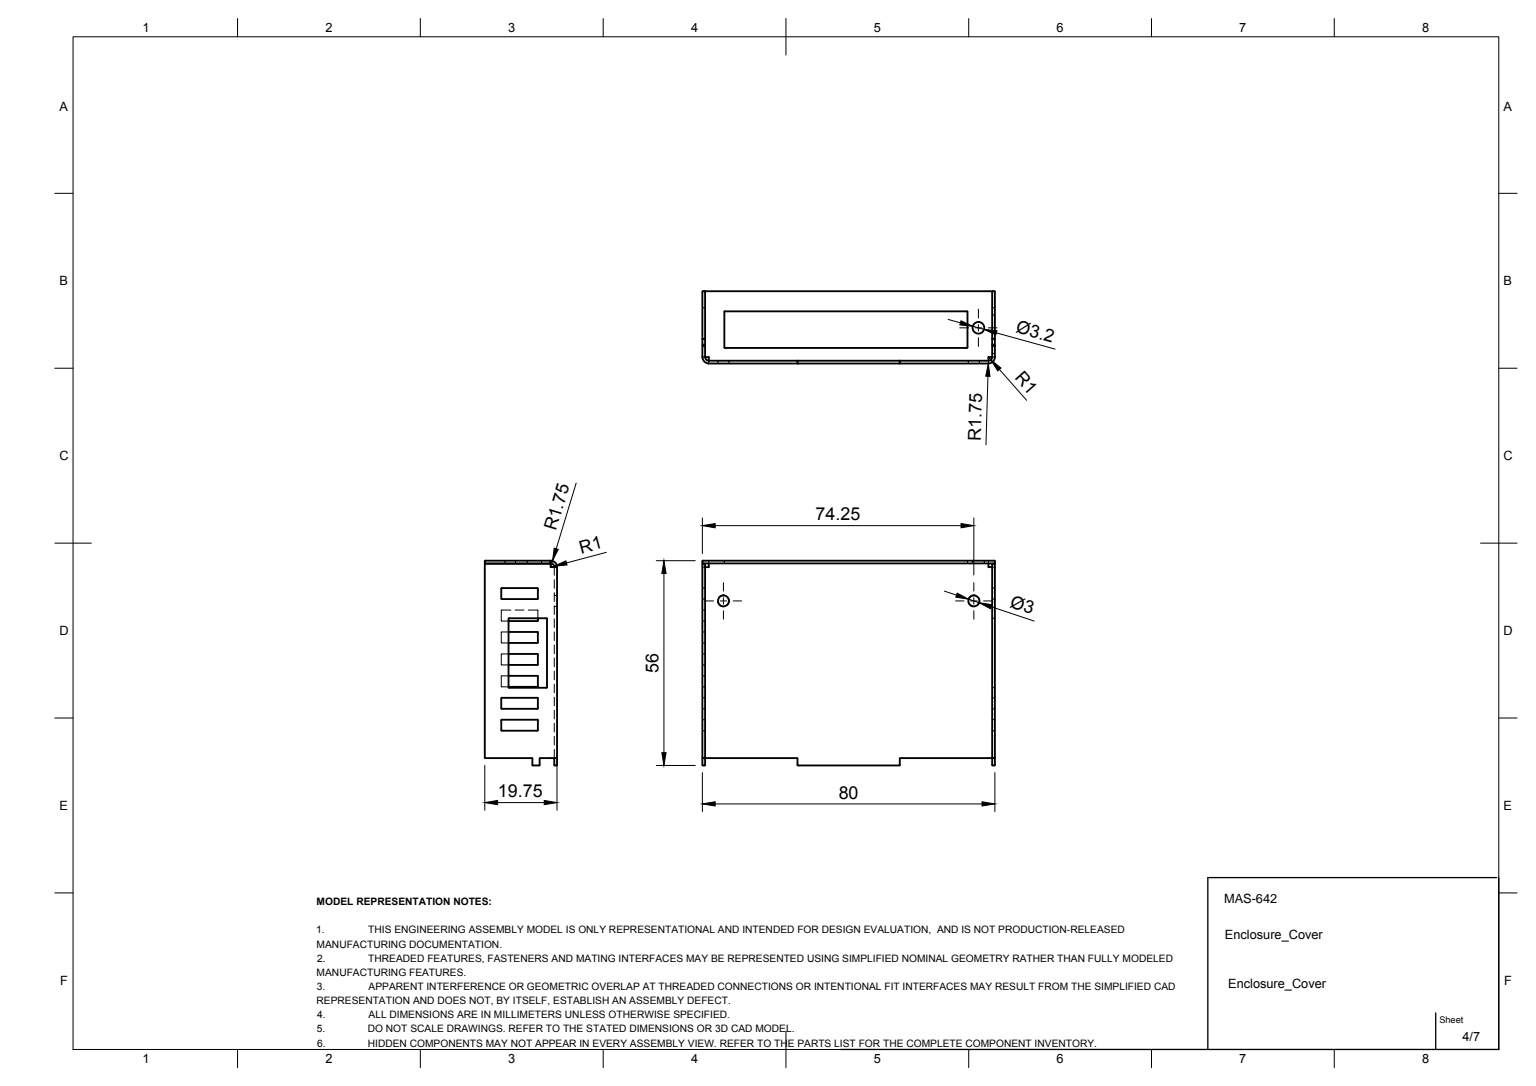
ISO-10303-21;
HEADER;
FILE_DESCRIPTION((''),'2;1');
FILE_NAME('Enclosure_Cover.step','2026-10-09T09:51:33-07:00',(''),(''),'','','');
FILE_SCHEMA (('AUTOMOTIVE_DESIGN { 1 0 10303 214 3 1 1 }'));
ENDSEC;
DATA;
#10=MECHANICAL_DESIGN_GEOMETRIC_PRESENTATION_REPRESENTATION('',(#481),#126571);
#469=SHAPE_REPRESENTATION_RELATIONSHIP('SRR','None',#126599,#475) ;
#475=ADVANCED_BREP_SHAPE_REPRESENTATION('',(#4172),#126565) ;
#481=STYLED_ITEM('',(#126638),#4172) ;
#4172=MANIFOLD_SOLID_BREP('Body1',#67686) ;
#4182=SPHERICAL_SURFACE('',#68025,0.15) ;
#4183=SPHERICAL_SURFACE('',#68034,0.15) ;
#4184=SPHERICAL_SURFACE('',#68036,0.15) ;
#4185=SPHERICAL_SURFACE('',#68045,0.15) ;
#4186=SPHERICAL_SURFACE('',#68058,0.15) ;
#4187=SPHERICAL_SURFACE('',#68067,0.15) ;
#4188=SPHERICAL_SURFACE('',#68069,0.15) ;
#4189=SPHERICAL_SURFACE('',#68081,0.15) ;
#4190=SPHERICAL_SURFACE('',#68086,0.15) ;
#4191=SPHERICAL_SURFACE('',#68107,0.15) ;
#4192=SPHERICAL_SURFACE('',#68110,0.15) ;
#4193=SPHERICAL_SURFACE('',#68130,0.15) ;
#4194=SPHERICAL_SURFACE('',#68146,0.15) ;
#4195=SPHERICAL_SURFACE('',#68149,0.15) ;
#4196=SPHERICAL_SURFACE('',#68166,0.15) ;
#4197=SPHERICAL_SURFACE('',#68168,0.15) ;
#4198=SPHERICAL_SURFACE('',#68174,0.15) ;
#4199=SPHERICAL_SURFACE('',#68177,0.15) ;
#4200=SPHERICAL_SURFACE('',#68195,0.15) ;
#4201=SPHERICAL_SURFACE('',#68201,0.15) ;
#4202=SPHERICAL_SURFACE('',#68757,0.15) ;
#4203=SPHERICAL_SURFACE('',#68763,0.15) ;
#4204=SPHERICAL_SURFACE('',#68773,0.15) ;
#4205=SPHERICAL_SURFACE('',#68775,0.15) ;
#4840=ELLIPSE('',#68022,0.212132034355858,0.149999999999913) ;
#4841=ELLIPSE('',#68024,0.212132034356981,0.150000000000627) ;
#4842=ELLIPSE('',#68079,0.21213203435611,0.150000000000114) ;
#4843=ELLIPSE('',#68090,0.212132034356462,0.150000000000298) ;
#4844=ELLIPSE('',#68749,0.212132034356202,0.150000000000162) ;
#4845=ELLIPSE('',#68753,0.212132034355904,0.149999999999933) ;
#4846=ELLIPSE('',#68760,0.212132034354929,0.149999999999304) ;
#4847=ELLIPSE('',#68762,0.212132034356004,0.150000000000028) ;
#4989=FACE_BOUND('',#20413,.T.) ;
#4990=FACE_BOUND('',#20414,.T.) ;
#4991=FACE_BOUND('',#20416,.T.) ;
#4992=FACE_BOUND('',#20417,.T.) ;
#4993=FACE_BOUND('',#20419,.T.) ;
#4994=FACE_BOUND('',#20420,.T.) ;
#4995=FACE_BOUND('',#20421,.T.) ;
#4996=FACE_BOUND('',#20422,.T.) ;
#4997=FACE_BOUND('',#20424,.T.) ;
#4998=FACE_BOUND('',#20425,.T.) ;
#4999=FACE_BOUND('',#20426,.T.) ;
#5000=FACE_BOUND('',#20427,.T.) ;
#5001=FACE_BOUND('',#20429,.T.) ;
#5002=FACE_BOUND('',#20430,.T.) ;
#5003=FACE_BOUND('',#20431,.T.) ;
#5004=FACE_BOUND('',#20432,.T.) ;
#5005=FACE_BOUND('',#20433,.T.) ;
#5006=FACE_BOUND('',#20434,.T.) ;
#5007=FACE_BOUND('',#20435,.T.) ;
#5008=FACE_BOUND('',#20437,.T.) ;
#5009=FACE_BOUND('',#20438,.T.) ;
#5010=FACE_BOUND('',#20439,.T.) ;
#5011=FACE_BOUND('',#20440,.T.) ;
#5012=FACE_BOUND('',#20441,.T.) ;
#5013=FACE_BOUND('',#20442,.T.) ;
#5014=FACE_BOUND('',#20443,.T.) ;
#5015=FACE_BOUND('',#20445,.T.) ;
#5016=FACE_BOUND('',#20446,.T.) ;
#5017=FACE_BOUND('',#20448,.T.) ;
#5018=FACE_BOUND('',#20449,.T.) ;
#5065=PLANE('',#67802) ;
#5066=PLANE('',#67807) ;
#5067=PLANE('',#67812) ;
#5068=PLANE('',#67831) ;
#5069=PLANE('',#67850) ;
#5070=PLANE('',#67881) ;
#5071=PLANE('',#67912) ;
#5072=PLANE('',#67915) ;
#5073=PLANE('',#67918) ;
#5074=PLANE('',#67919) ;
#5075=PLANE('',#67920) ;
#5076=PLANE('',#67921) ;
#5077=PLANE('',#67922) ;
#5078=PLANE('',#67923) ;
#5079=PLANE('',#67926) ;
#5080=PLANE('',#67933) ;
#5081=PLANE('',#67934) ;
#5082=PLANE('',#67935) ;
#5083=PLANE('',#67936) ;
#5084=PLANE('',#67937) ;
#5085=PLANE('',#67938) ;
#5086=PLANE('',#67939) ;
#5087=PLANE('',#67940) ;
#5088=PLANE('',#67941) ;
#5089=PLANE('',#67942) ;
#5090=PLANE('',#67943) ;
#5091=PLANE('',#67944) ;
#5092=PLANE('',#67945) ;
#5093=PLANE('',#67946) ;
#5094=PLANE('',#67949) ;
#5095=PLANE('',#67954) ;
#5096=PLANE('',#67957) ;
#5097=PLANE('',#67964) ;
#5098=PLANE('',#67965) ;
#5099=PLANE('',#67966) ;
#5100=PLANE('',#67967) ;
#5101=PLANE('',#67968) ;
#5102=PLANE('',#67969) ;
#5103=PLANE('',#67970) ;
#5104=PLANE('',#67971) ;
#5105=PLANE('',#67972) ;
#5106=PLANE('',#67973) ;
#5107=PLANE('',#67974) ;
#5108=PLANE('',#67975) ;
#5109=PLANE('',#67976) ;
#5110=PLANE('',#67977) ;
#5111=PLANE('',#67978) ;
#5112=PLANE('',#67979) ;
#5113=PLANE('',#67980) ;
#5114=PLANE('',#67981) ;
#5115=PLANE('',#67982) ;
#5116=PLANE('',#67983) ;
#5117=PLANE('',#67984) ;
#5118=PLANE('',#67985) ;
#5119=PLANE('',#67986) ;
#5120=PLANE('',#67987) ;
#5121=PLANE('',#67988) ;
#5122=PLANE('',#67989) ;
#5123=PLANE('',#67990) ;
#5124=PLANE('',#67991) ;
#5125=PLANE('',#67992) ;
#5126=PLANE('',#67993) ;
#5127=PLANE('',#67994) ;
#5128=PLANE('',#67995) ;
#5129=PLANE('',#67996) ;
#5130=PLANE('',#67997) ;
#5131=PLANE('',#67998) ;
#5132=PLANE('',#67999) ;
#5133=PLANE('',#68000) ;
#5134=PLANE('',#68001) ;
#5135=PLANE('',#68002) ;
#5136=PLANE('',#68003) ;
#5137=PLANE('',#68004) ;
#5138=PLANE('',#68005) ;
#5139=PLANE('',#68006) ;
#5140=PLANE('',#68007) ;
#5141=PLANE('',#68008) ;
#5142=PLANE('',#68009) ;
#5143=PLANE('',#68010) ;
#5144=PLANE('',#68011) ;
#5145=PLANE('',#68012) ;
#5146=PLANE('',#68013) ;
#5147=PLANE('',#68014) ;
#5148=PLANE('',#68015) ;
#5149=PLANE('',#68016) ;
#5150=PLANE('',#68017) ;
#5151=PLANE('',#68018) ;
#5152=PLANE('',#68019) ;
#5947=CYLINDRICAL_SURFACE('',#67797,1.49999999999999) ;
#5948=CYLINDRICAL_SURFACE('',#67800,1.49999999999999) ;
#5949=CYLINDRICAL_SURFACE('',#67801,1.6) ;
#5950=CYLINDRICAL_SURFACE('',#67929,1.75) ;
#5951=CYLINDRICAL_SURFACE('',#67931,1.) ;
#5952=CYLINDRICAL_SURFACE('',#67952,1.75) ;
#5953=CYLINDRICAL_SURFACE('',#67953,1.) ;
#5954=CYLINDRICAL_SURFACE('',#67960,1.75) ;
#5955=CYLINDRICAL_SURFACE('',#67962,1.) ;
#5956=CYLINDRICAL_SURFACE('',#68020,0.149999999999997) ;
#5957=CYLINDRICAL_SURFACE('',#68023,0.15) ;
#5958=CYLINDRICAL_SURFACE('',#68028,0.149999999999997) ;
#5959=CYLINDRICAL_SURFACE('',#68030,0.149999999999997) ;
#5960=CYLINDRICAL_SURFACE('',#68032,0.149999999999997) ;
#5961=CYLINDRICAL_SURFACE('',#68039,0.149999999999997) ;
#5962=CYLINDRICAL_SURFACE('',#68041,0.15) ;
#5963=CYLINDRICAL_SURFACE('',#68043,0.149999999999997) ;
#5964=CYLINDRICAL_SURFACE('',#68050,0.149999999999997) ;
#5965=CYLINDRICAL_SURFACE('',#68052,0.15) ;
#5966=CYLINDRICAL_SURFACE('',#68054,0.149999999999997) ;
#5967=CYLINDRICAL_SURFACE('',#68061,0.149999999999997) ;
#5968=CYLINDRICAL_SURFACE('',#68063,0.15) ;
#5969=CYLINDRICAL_SURFACE('',#68065,0.149999999999997) ;
#5970=CYLINDRICAL_SURFACE('',#68072,0.149999999999997) ;
#5971=CYLINDRICAL_SURFACE('',#68074,0.15) ;
#5972=CYLINDRICAL_SURFACE('',#68076,0.149999999999997) ;
#5973=CYLINDRICAL_SURFACE('',#68078,0.149999999999997) ;
#5974=CYLINDRICAL_SURFACE('',#68089,0.15) ;
#5975=CYLINDRICAL_SURFACE('',#68091,0.149999999999997) ;
#5976=CYLINDRICAL_SURFACE('',#68093,0.15) ;
#5977=CYLINDRICAL_SURFACE('',#68095,0.149999999999997) ;
#5978=CYLINDRICAL_SURFACE('',#68097,0.150000000000001) ;
#5979=CYLINDRICAL_SURFACE('',#68099,0.150000000000001) ;
#5980=CYLINDRICAL_SURFACE('',#68101,0.149999999999997) ;
#5981=CYLINDRICAL_SURFACE('',#68112,0.149999999999997) ;
#5982=CYLINDRICAL_SURFACE('',#68114,0.15) ;
#5983=CYLINDRICAL_SURFACE('',#68116,0.15) ;
#5984=CYLINDRICAL_SURFACE('',#68118,0.15) ;
#5985=CYLINDRICAL_SURFACE('',#68120,0.150000000000001) ;
#5986=CYLINDRICAL_SURFACE('',#68132,0.15) ;
#5987=CYLINDRICAL_SURFACE('',#68134,0.150000000000001) ;
#5988=CYLINDRICAL_SURFACE('',#68136,0.15) ;
#5989=CYLINDRICAL_SURFACE('',#68138,0.15) ;
#5990=CYLINDRICAL_SURFACE('',#68140,0.15) ;
#5991=CYLINDRICAL_SURFACE('',#68142,0.15) ;
#5992=CYLINDRICAL_SURFACE('',#68154,0.15) ;
#5993=CYLINDRICAL_SURFACE('',#68156,0.150000000000001) ;
#5994=CYLINDRICAL_SURFACE('',#68158,0.15) ;
#5995=CYLINDRICAL_SURFACE('',#68160,0.15) ;
#5996=CYLINDRICAL_SURFACE('',#68162,0.15) ;
#5997=CYLINDRICAL_SURFACE('',#68164,0.15) ;
#5998=CYLINDRICAL_SURFACE('',#68179,0.15) ;
#5999=CYLINDRICAL_SURFACE('',#68181,0.150000000000001) ;
#6000=CYLINDRICAL_SURFACE('',#68183,0.15) ;
#6001=CYLINDRICAL_SURFACE('',#68185,0.15) ;
#6002=CYLINDRICAL_SURFACE('',#68187,0.15) ;
#6003=CYLINDRICAL_SURFACE('',#68189,0.15) ;
#6004=CYLINDRICAL_SURFACE('',#68191,0.15) ;
#6005=CYLINDRICAL_SURFACE('',#68193,0.15) ;
#6006=CYLINDRICAL_SURFACE('',#68203,0.15) ;
#6007=CYLINDRICAL_SURFACE('',#68205,0.150000000000001) ;
#6008=CYLINDRICAL_SURFACE('',#68207,0.15) ;
#6009=CYLINDRICAL_SURFACE('',#68209,0.15) ;
#6010=CYLINDRICAL_SURFACE('',#68215,0.15) ;
#6011=CYLINDRICAL_SURFACE('',#68217,0.15) ;
#6012=CYLINDRICAL_SURFACE('',#68220,0.149999999999997) ;
#6013=CYLINDRICAL_SURFACE('',#68229,0.15) ;
#6014=CYLINDRICAL_SURFACE('',#68231,0.149999999999997) ;
#6015=CYLINDRICAL_SURFACE('',#68233,0.149999999999997) ;
#6016=CYLINDRICAL_SURFACE('',#68236,0.149999999999997) ;
#6017=CYLINDRICAL_SURFACE('',#68238,0.15) ;
#6018=CYLINDRICAL_SURFACE('',#68240,0.149999999999997) ;
#6019=CYLINDRICAL_SURFACE('',#68251,0.149999999999997) ;
#6020=CYLINDRICAL_SURFACE('',#68253,0.150000000000001) ;
#6021=CYLINDRICAL_SURFACE('',#68255,0.150000000000001) ;
#6022=CYLINDRICAL_SURFACE('',#68257,0.149999999999997) ;
#6023=CYLINDRICAL_SURFACE('',#68263,0.149999999999997) ;
#6024=CYLINDRICAL_SURFACE('',#68264,0.149999999999997) ;
#6025=CYLINDRICAL_SURFACE('',#68273,0.150000000000001) ;
#6026=CYLINDRICAL_SURFACE('',#68275,0.149999999999997) ;
#6027=CYLINDRICAL_SURFACE('',#68277,0.149999999999997) ;
#6028=CYLINDRICAL_SURFACE('',#68280,0.149999999999997) ;
#6029=CYLINDRICAL_SURFACE('',#68282,0.150000000000001) ;
#6030=CYLINDRICAL_SURFACE('',#68284,0.149999999999997) ;
#6031=CYLINDRICAL_SURFACE('',#68295,0.149999999999997) ;
#6032=CYLINDRICAL_SURFACE('',#68297,0.15) ;
#6033=CYLINDRICAL_SURFACE('',#68299,0.15) ;
#6034=CYLINDRICAL_SURFACE('',#68301,0.149999999999997) ;
#6035=CYLINDRICAL_SURFACE('',#68307,0.149999999999997) ;
#6036=CYLINDRICAL_SURFACE('',#68308,0.149999999999997) ;
#6037=CYLINDRICAL_SURFACE('',#68317,0.15) ;
#6038=CYLINDRICAL_SURFACE('',#68319,0.149999999999997) ;
#6039=CYLINDRICAL_SURFACE('',#68321,0.149999999999997) ;
#6040=CYLINDRICAL_SURFACE('',#68324,0.149999999999997) ;
#6041=CYLINDRICAL_SURFACE('',#68326,0.15) ;
#6042=CYLINDRICAL_SURFACE('',#68328,0.149999999999997) ;
#6043=CYLINDRICAL_SURFACE('',#68339,0.149999999999997) ;
#6044=CYLINDRICAL_SURFACE('',#68341,0.150000000000001) ;
#6045=CYLINDRICAL_SURFACE('',#68343,0.150000000000001) ;
#6046=CYLINDRICAL_SURFACE('',#68345,0.149999999999997) ;
#6047=CYLINDRICAL_SURFACE('',#68351,0.149999999999997) ;
#6048=CYLINDRICAL_SURFACE('',#68352,0.149999999999997) ;
#6049=CYLINDRICAL_SURFACE('',#68361,0.150000000000001) ;
#6050=CYLINDRICAL_SURFACE('',#68363,0.149999999999997) ;
#6051=CYLINDRICAL_SURFACE('',#68365,0.149999999999997) ;
#6052=CYLINDRICAL_SURFACE('',#68368,0.149999999999997) ;
#6053=CYLINDRICAL_SURFACE('',#68370,0.150000000000001) ;
#6054=CYLINDRICAL_SURFACE('',#68372,0.149999999999997) ;
#6055=CYLINDRICAL_SURFACE('',#68383,0.149999999999997) ;
#6056=CYLINDRICAL_SURFACE('',#68385,0.15) ;
#6057=CYLINDRICAL_SURFACE('',#68387,0.15) ;
#6058=CYLINDRICAL_SURFACE('',#68389,0.149999999999997) ;
#6059=CYLINDRICAL_SURFACE('',#68395,0.149999999999997) ;
#6060=CYLINDRICAL_SURFACE('',#68396,0.149999999999997) ;
#6061=CYLINDRICAL_SURFACE('',#68405,0.149999999999997) ;
#6062=CYLINDRICAL_SURFACE('',#68407,0.150000000000001) ;
#6063=CYLINDRICAL_SURFACE('',#68409,0.149999999999997) ;
#6064=CYLINDRICAL_SURFACE('',#68412,0.150000000000001) ;
#6065=CYLINDRICAL_SURFACE('',#68414,0.149999999999997) ;
#6066=CYLINDRICAL_SURFACE('',#68416,0.149999999999997) ;
#6067=CYLINDRICAL_SURFACE('',#68427,0.15) ;
#6068=CYLINDRICAL_SURFACE('',#68429,0.149999999999997) ;
#6069=CYLINDRICAL_SURFACE('',#68431,0.149999999999997) ;
#6070=CYLINDRICAL_SURFACE('',#68433,0.15) ;
#6071=CYLINDRICAL_SURFACE('',#68439,0.149999999999997) ;
#6072=CYLINDRICAL_SURFACE('',#68440,0.149999999999997) ;
#6073=CYLINDRICAL_SURFACE('',#68449,0.149999999999997) ;
#6074=CYLINDRICAL_SURFACE('',#68451,0.149999999999997) ;
#6075=CYLINDRICAL_SURFACE('',#68453,0.149999999999997) ;
#6076=CYLINDRICAL_SURFACE('',#68456,0.149999999999997) ;
#6077=CYLINDRICAL_SURFACE('',#68458,0.149999999999997) ;
#6078=CYLINDRICAL_SURFACE('',#68460,0.149999999999997) ;
#6079=CYLINDRICAL_SURFACE('',#68471,0.149999999999997) ;
#6080=CYLINDRICAL_SURFACE('',#68473,0.149999999999997) ;
#6081=CYLINDRICAL_SURFACE('',#68475,0.149999999999997) ;
#6082=CYLINDRICAL_SURFACE('',#68477,0.149999999999997) ;
#6083=CYLINDRICAL_SURFACE('',#68483,0.149999999999997) ;
#6084=CYLINDRICAL_SURFACE('',#68484,0.149999999999997) ;
#6085=CYLINDRICAL_SURFACE('',#68493,0.149999999999997) ;
#6086=CYLINDRICAL_SURFACE('',#68495,0.149999999999997) ;
#6087=CYLINDRICAL_SURFACE('',#68497,0.149999999999997) ;
#6088=CYLINDRICAL_SURFACE('',#68500,0.149999999999997) ;
#6089=CYLINDRICAL_SURFACE('',#68502,0.149999999999997) ;
#6090=CYLINDRICAL_SURFACE('',#68504,0.149999999999997) ;
#6091=CYLINDRICAL_SURFACE('',#68515,0.149999999999997) ;
#6092=CYLINDRICAL_SURFACE('',#68517,0.149999999999997) ;
#6093=CYLINDRICAL_SURFACE('',#68519,0.149999999999997) ;
#6094=CYLINDRICAL_SURFACE('',#68521,0.149999999999997) ;
#6095=CYLINDRICAL_SURFACE('',#68527,0.149999999999997) ;
#6096=CYLINDRICAL_SURFACE('',#68528,0.149999999999997) ;
#6097=CYLINDRICAL_SURFACE('',#68537,0.149999999999997) ;
#6098=CYLINDRICAL_SURFACE('',#68539,0.149999999999997) ;
#6099=CYLINDRICAL_SURFACE('',#68541,0.149999999999997) ;
#6100=CYLINDRICAL_SURFACE('',#68544,0.149999999999997) ;
#6101=CYLINDRICAL_SURFACE('',#68546,0.149999999999997) ;
#6102=CYLINDRICAL_SURFACE('',#68548,0.149999999999997) ;
#6103=CYLINDRICAL_SURFACE('',#68559,0.149999999999997) ;
#6104=CYLINDRICAL_SURFACE('',#68561,0.149999999999997) ;
#6105=CYLINDRICAL_SURFACE('',#68563,0.149999999999997) ;
#6106=CYLINDRICAL_SURFACE('',#68565,0.149999999999997) ;
#6107=CYLINDRICAL_SURFACE('',#68571,0.149999999999997) ;
#6108=CYLINDRICAL_SURFACE('',#68572,0.149999999999997) ;
#6109=CYLINDRICAL_SURFACE('',#68581,0.150000000000001) ;
#6110=CYLINDRICAL_SURFACE('',#68583,0.150000000000001) ;
#6111=CYLINDRICAL_SURFACE('',#68585,0.149999999999997) ;
#6112=CYLINDRICAL_SURFACE('',#68588,0.149999999999997) ;
#6113=CYLINDRICAL_SURFACE('',#68590,0.150000000000001) ;
#6114=CYLINDRICAL_SURFACE('',#68592,0.149999999999997) ;
#6115=CYLINDRICAL_SURFACE('',#68603,0.150000000000001) ;
#6116=CYLINDRICAL_SURFACE('',#68605,0.150000000000001) ;
#6117=CYLINDRICAL_SURFACE('',#68607,0.150000000000001) ;
#6118=CYLINDRICAL_SURFACE('',#68609,0.149999999999997) ;
#6119=CYLINDRICAL_SURFACE('',#68615,0.149999999999997) ;
#6120=CYLINDRICAL_SURFACE('',#68616,0.149999999999997) ;
#6121=CYLINDRICAL_SURFACE('',#68625,0.150000000000001) ;
#6122=CYLINDRICAL_SURFACE('',#68627,0.149999999999997) ;
#6123=CYLINDRICAL_SURFACE('',#68629,0.149999999999997) ;
#6124=CYLINDRICAL_SURFACE('',#68632,0.150000000000001) ;
#6125=CYLINDRICAL_SURFACE('',#68634,0.150000000000001) ;
#6126=CYLINDRICAL_SURFACE('',#68636,0.149999999999997) ;
#6127=CYLINDRICAL_SURFACE('',#68647,0.149999999999997) ;
#6128=CYLINDRICAL_SURFACE('',#68649,0.150000000000001) ;
#6129=CYLINDRICAL_SURFACE('',#68651,0.150000000000001) ;
#6130=CYLINDRICAL_SURFACE('',#68653,0.150000000000001) ;
#6131=CYLINDRICAL_SURFACE('',#68659,0.149999999999997) ;
#6132=CYLINDRICAL_SURFACE('',#68660,0.149999999999997) ;
#6133=CYLINDRICAL_SURFACE('',#68669,0.150000000000001) ;
#6134=CYLINDRICAL_SURFACE('',#68671,0.150000000000001) ;
#6135=CYLINDRICAL_SURFACE('',#68673,0.149999999999997) ;
#6136=CYLINDRICAL_SURFACE('',#68676,0.149999999999997) ;
#6137=CYLINDRICAL_SURFACE('',#68678,0.150000000000001) ;
#6138=CYLINDRICAL_SURFACE('',#68680,0.149999999999997) ;
#6139=CYLINDRICAL_SURFACE('',#68691,0.150000000000001) ;
#6140=CYLINDRICAL_SURFACE('',#68693,0.150000000000001) ;
#6141=CYLINDRICAL_SURFACE('',#68695,0.150000000000001) ;
#6142=CYLINDRICAL_SURFACE('',#68697,0.149999999999997) ;
#6143=CYLINDRICAL_SURFACE('',#68703,0.149999999999997) ;
#6144=CYLINDRICAL_SURFACE('',#68704,0.149999999999997) ;
#6145=CYLINDRICAL_SURFACE('',#68713,0.150000000000001) ;
#6146=CYLINDRICAL_SURFACE('',#68715,0.150000000000001) ;
#6147=CYLINDRICAL_SURFACE('',#68717,0.149999999999997) ;
#6148=CYLINDRICAL_SURFACE('',#68720,0.15) ;
#6149=CYLINDRICAL_SURFACE('',#68722,0.15) ;
#6150=CYLINDRICAL_SURFACE('',#68724,0.149999999999997) ;
#6151=CYLINDRICAL_SURFACE('',#68735,0.150000000000001) ;
#6152=CYLINDRICAL_SURFACE('',#68737,0.150000000000001) ;
#6153=CYLINDRICAL_SURFACE('',#68739,0.15) ;
#6154=CYLINDRICAL_SURFACE('',#68741,0.15) ;
#6155=CYLINDRICAL_SURFACE('',#68747,0.149999999999997) ;
#6156=CYLINDRICAL_SURFACE('',#68748,0.149999999999997) ;
#6157=CYLINDRICAL_SURFACE('',#68751,0.149999999999997) ;
#6158=CYLINDRICAL_SURFACE('',#68754,0.150000000000001) ;
#6159=CYLINDRICAL_SURFACE('',#68759,0.15) ;
#6160=CYLINDRICAL_SURFACE('',#68761,0.15) ;
#6161=CYLINDRICAL_SURFACE('',#68765,0.150000000000001) ;
#6162=CYLINDRICAL_SURFACE('',#68767,0.149999999999997) ;
#6163=CYLINDRICAL_SURFACE('',#68769,0.149999999999997) ;
#6164=CYLINDRICAL_SURFACE('',#68771,0.150000000000001) ;
#6165=CYLINDRICAL_SURFACE('',#68777,0.150000000000001) ;
#7896=LINE('',#99198,#12012) ;
#7897=LINE('',#99201,#12013) ;
#7898=LINE('',#99204,#12014) ;
#7899=LINE('',#99207,#12015) ;
#7900=LINE('',#99209,#12016) ;
#7901=LINE('',#99213,#12017) ;
#7902=LINE('',#99215,#12018) ;
#7903=LINE('',#99217,#12019) ;
#7904=LINE('',#99219,#12020) ;
#7905=LINE('',#99221,#12021) ;
#7906=LINE('',#99222,#12022) ;
#7907=LINE('',#99227,#12023) ;
#7908=LINE('',#99231,#12024) ;
#7909=LINE('',#99235,#12025) ;
#7910=LINE('',#99238,#12026) ;
#7911=LINE('',#99242,#12027) ;
#7912=LINE('',#99244,#12028) ;
#7913=LINE('',#99246,#12029) ;
#7914=LINE('',#99248,#12030) ;
#7915=LINE('',#99250,#12031) ;
#7916=LINE('',#99251,#12032) ;
#7917=LINE('',#99256,#12033) ;
#7918=LINE('',#99260,#12034) ;
#7919=LINE('',#99264,#12035) ;
#7920=LINE('',#99267,#12036) ;
#7921=LINE('',#99273,#12037) ;
#7922=LINE('',#99275,#12038) ;
#7923=LINE('',#99277,#12039) ;
#7924=LINE('',#99279,#12040) ;
#7925=LINE('',#99281,#12041) ;
#7926=LINE('',#99283,#12042) ;
#7927=LINE('',#99287,#12043) ;
#7928=LINE('',#99289,#12044) ;
#7929=LINE('',#99290,#12045) ;
#7930=LINE('',#99295,#12046) ;
#7931=LINE('',#99299,#12047) ;
#7932=LINE('',#99303,#12048) ;
#7933=LINE('',#99306,#12049) ;
#7934=LINE('',#99311,#12050) ;
#7935=LINE('',#99315,#12051) ;
#7936=LINE('',#99319,#12052) ;
#7937=LINE('',#99322,#12053) ;
#7938=LINE('',#99327,#12054) ;
#7939=LINE('',#99331,#12055) ;
#7940=LINE('',#99335,#12056) ;
#7941=LINE('',#99338,#12057) ;
#7942=LINE('',#99343,#12058) ;
#7943=LINE('',#99347,#12059) ;
#7944=LINE('',#99351,#12060) ;
#7945=LINE('',#99354,#12061) ;
#7946=LINE('',#99358,#12062) ;
#7947=LINE('',#99360,#12063) ;
#7948=LINE('',#99364,#12064) ;
#7949=LINE('',#99366,#12065) ;
#7950=LINE('',#99368,#12066) ;
#7951=LINE('',#99372,#12067) ;
#7952=LINE('',#99374,#12068) ;
#7953=LINE('',#99376,#12069) ;
#7954=LINE('',#99377,#12070) ;
#7955=LINE('',#99382,#12071) ;
#7956=LINE('',#99386,#12072) ;
#7957=LINE('',#99390,#12073) ;
#7958=LINE('',#99393,#12074) ;
#7959=LINE('',#99398,#12075) ;
#7960=LINE('',#99402,#12076) ;
#7961=LINE('',#99406,#12077) ;
#7962=LINE('',#99409,#12078) ;
#7963=LINE('',#99414,#12079) ;
#7964=LINE('',#99418,#12080) ;
#7965=LINE('',#99422,#12081) ;
#7966=LINE('',#99425,#12082) ;
#7967=LINE('',#99430,#12083) ;
#7968=LINE('',#99434,#12084) ;
#7969=LINE('',#99438,#12085) ;
#7970=LINE('',#99441,#12086) ;
#7971=LINE('',#99445,#12087) ;
#7972=LINE('',#99447,#12088) ;
#7973=LINE('',#99451,#12089) ;
#7974=LINE('',#99453,#12090) ;
#7975=LINE('',#99455,#12091) ;
#7976=LINE('',#99459,#12092) ;
#7977=LINE('',#99461,#12093) ;
#7978=LINE('',#99463,#12094) ;
#7979=LINE('',#99464,#12095) ;
#7980=LINE('',#99469,#12096) ;
#7981=LINE('',#99473,#12097) ;
#7982=LINE('',#99477,#12098) ;
#7983=LINE('',#99480,#12099) ;
#7984=LINE('',#99485,#12100) ;
#7985=LINE('',#99489,#12101) ;
#7986=LINE('',#99493,#12102) ;
#7987=LINE('',#99496,#12103) ;
#7988=LINE('',#99501,#12104) ;
#7989=LINE('',#99505,#12105) ;
#7990=LINE('',#99509,#12106) ;
#7991=LINE('',#99512,#12107) ;
#7992=LINE('',#99517,#12108) ;
#7993=LINE('',#99521,#12109) ;
#7994=LINE('',#99525,#12110) ;
#7995=LINE('',#99528,#12111) ;
#7996=LINE('',#99533,#12112) ;
#7997=LINE('',#99537,#12113) ;
#7998=LINE('',#99541,#12114) ;
#7999=LINE('',#99544,#12115) ;
#8000=LINE('',#99549,#12116) ;
#8001=LINE('',#99553,#12117) ;
#8002=LINE('',#99557,#12118) ;
#8003=LINE('',#99560,#12119) ;
#8004=LINE('',#99565,#12120) ;
#8005=LINE('',#99569,#12121) ;
#8006=LINE('',#99573,#12122) ;
#8007=LINE('',#99576,#12123) ;
#8008=LINE('',#99582,#12124) ;
#8009=LINE('',#99584,#12125) ;
#8010=LINE('',#99586,#12126) ;
#8011=LINE('',#99588,#12127) ;
#8012=LINE('',#99590,#12128) ;
#8013=LINE('',#99592,#12129) ;
#8014=LINE('',#99596,#12130) ;
#8015=LINE('',#99598,#12131) ;
#8016=LINE('',#99599,#12132) ;
#8017=LINE('',#99604,#12133) ;
#8018=LINE('',#99608,#12134) ;
#8019=LINE('',#99612,#12135) ;
#8020=LINE('',#99615,#12136) ;
#8021=LINE('',#99620,#12137) ;
#8022=LINE('',#99624,#12138) ;
#8023=LINE('',#99628,#12139) ;
#8024=LINE('',#99631,#12140) ;
#8025=LINE('',#99636,#12141) ;
#8026=LINE('',#99640,#12142) ;
#8027=LINE('',#99644,#12143) ;
#8028=LINE('',#99647,#12144) ;
#8029=LINE('',#99652,#12145) ;
#8030=LINE('',#99656,#12146) ;
#8031=LINE('',#99660,#12147) ;
#8032=LINE('',#99663,#12148) ;
#8033=LINE('',#99668,#12149) ;
#8034=LINE('',#99672,#12150) ;
#8035=LINE('',#99676,#12151) ;
#8036=LINE('',#99679,#12152) ;
#8037=LINE('',#99684,#12153) ;
#8038=LINE('',#99688,#12154) ;
#8039=LINE('',#99692,#12155) ;
#8040=LINE('',#99695,#12156) ;
#8041=LINE('',#99700,#12157) ;
#8042=LINE('',#99704,#12158) ;
#8043=LINE('',#99708,#12159) ;
#8044=LINE('',#99711,#12160) ;
#8045=LINE('',#99717,#12161) ;
#8046=LINE('',#99719,#12162) ;
#8047=LINE('',#99721,#12163) ;
#8048=LINE('',#99723,#12164) ;
#8049=LINE('',#99725,#12165) ;
#8050=LINE('',#99729,#12166) ;
#8051=LINE('',#99731,#12167) ;
#8052=LINE('',#99732,#12168) ;
#8053=LINE('',#99736,#12169) ;
#8054=LINE('',#99738,#12170) ;
#8055=LINE('',#99742,#12171) ;
#8056=LINE('',#99744,#12172) ;
#8057=LINE('',#99746,#12173) ;
#8058=LINE('',#99750,#12174) ;
#8059=LINE('',#99752,#12175) ;
#8060=LINE('',#99753,#12176) ;
#8061=LINE('',#99757,#12177) ;
#8062=LINE('',#99759,#12178) ;
#8063=LINE('',#99761,#12179) ;
#8064=LINE('',#99762,#12180) ;
#8065=LINE('',#99766,#12181) ;
#8066=LINE('',#99768,#12182) ;
#8067=LINE('',#99770,#12183) ;
#8068=LINE('',#99771,#12184) ;
#8069=LINE('',#99775,#12185) ;
#8070=LINE('',#99777,#12186) ;
#8071=LINE('',#99779,#12187) ;
#8072=LINE('',#99780,#12188) ;
#8073=LINE('',#99784,#12189) ;
#8074=LINE('',#99786,#12190) ;
#8075=LINE('',#99788,#12191) ;
#8076=LINE('',#99789,#12192) ;
#8077=LINE('',#99793,#12193) ;
#8078=LINE('',#99795,#12194) ;
#8079=LINE('',#99797,#12195) ;
#8080=LINE('',#99798,#12196) ;
#8081=LINE('',#99803,#12197) ;
#8082=LINE('',#99807,#12198) ;
#8083=LINE('',#99809,#12199) ;
#8084=LINE('',#99817,#12200) ;
#8085=LINE('',#99819,#12201) ;
#8086=LINE('',#99821,#12202) ;
#8087=LINE('',#99822,#12203) ;
#8088=LINE('',#99826,#12204) ;
#8089=LINE('',#99828,#12205) ;
#8090=LINE('',#99830,#12206) ;
#8091=LINE('',#99831,#12207) ;
#8092=LINE('',#99835,#12208) ;
#8093=LINE('',#99837,#12209) ;
#8094=LINE('',#99839,#12210) ;
#8095=LINE('',#99840,#12211) ;
#8096=LINE('',#99844,#12212) ;
#8097=LINE('',#99846,#12213) ;
#8098=LINE('',#99848,#12214) ;
#8099=LINE('',#99849,#12215) ;
#8100=LINE('',#99853,#12216) ;
#8101=LINE('',#99855,#12217) ;
#8102=LINE('',#99857,#12218) ;
#8103=LINE('',#99858,#12219) ;
#8104=LINE('',#99862,#12220) ;
#8105=LINE('',#99864,#12221) ;
#8106=LINE('',#99866,#12222) ;
#8107=LINE('',#99867,#12223) ;
#8108=LINE('',#99870,#12224) ;
#8109=LINE('',#99872,#12225) ;
#8110=LINE('',#99873,#12226) ;
#8111=LINE('',#99875,#12227) ;
#8112=LINE('',#99879,#12228) ;
#8113=LINE('',#99881,#12229) ;
#8114=LINE('',#99883,#12230) ;
#8115=LINE('',#99884,#12231) ;
#8116=LINE('',#99888,#12232) ;
#8117=LINE('',#99890,#12233) ;
#8118=LINE('',#99892,#12234) ;
#8119=LINE('',#99893,#12235) ;
#8120=LINE('',#99897,#12236) ;
#8121=LINE('',#99899,#12237) ;
#8122=LINE('',#99901,#12238) ;
#8123=LINE('',#99902,#12239) ;
#8124=LINE('',#99904,#12240) ;
#8125=LINE('',#99905,#12241) ;
#8126=LINE('',#99907,#12242) ;
#8127=LINE('',#99908,#12243) ;
#8128=LINE('',#99911,#12244) ;
#8129=LINE('',#99921,#12245) ;
#8130=LINE('',#99926,#12246) ;
#8131=LINE('',#99935,#12247) ;
#8132=LINE('',#99937,#12248) ;
#8133=LINE('',#99939,#12249) ;
#8134=LINE('',#99940,#12250) ;
#8135=LINE('',#99944,#12251) ;
#8136=LINE('',#99946,#12252) ;
#8137=LINE('',#99948,#12253) ;
#8138=LINE('',#99949,#12254) ;
#8139=LINE('',#99953,#12255) ;
#8140=LINE('',#99955,#12256) ;
#8141=LINE('',#99957,#12257) ;
#8142=LINE('',#99958,#12258) ;
#8143=LINE('',#99962,#12259) ;
#8144=LINE('',#99964,#12260) ;
#8145=LINE('',#99966,#12261) ;
#8146=LINE('',#99967,#12262) ;
#8147=LINE('',#99971,#12263) ;
#8148=LINE('',#99973,#12264) ;
#8149=LINE('',#99975,#12265) ;
#8150=LINE('',#99976,#12266) ;
#8151=LINE('',#99980,#12267) ;
#8152=LINE('',#99982,#12268) ;
#8153=LINE('',#99984,#12269) ;
#8154=LINE('',#99985,#12270) ;
#8155=LINE('',#99987,#12271) ;
#8156=LINE('',#99991,#12272) ;
#8157=LINE('',#99992,#12273) ;
#8158=LINE('',#99993,#12274) ;
#8159=LINE('',#99997,#12275) ;
#8160=LINE('',#99999,#12276) ;
#8161=LINE('',#100001,#12277) ;
#8162=LINE('',#100002,#12278) ;
#8163=LINE('',#100006,#12279) ;
#8164=LINE('',#100008,#12280) ;
#8165=LINE('',#100010,#12281) ;
#8166=LINE('',#100011,#12282) ;
#8167=LINE('',#100015,#12283) ;
#8168=LINE('',#100017,#12284) ;
#8169=LINE('',#100019,#12285) ;
#8170=LINE('',#100020,#12286) ;
#8171=LINE('',#100024,#12287) ;
#8172=LINE('',#100026,#12288) ;
#8173=LINE('',#100028,#12289) ;
#8174=LINE('',#100029,#12290) ;
#8175=LINE('',#100033,#12291) ;
#8176=LINE('',#100035,#12292) ;
#8177=LINE('',#100037,#12293) ;
#8178=LINE('',#100038,#12294) ;
#8179=LINE('',#100042,#12295) ;
#8180=LINE('',#100044,#12296) ;
#8181=LINE('',#100046,#12297) ;
#8182=LINE('',#100047,#12298) ;
#8183=LINE('',#100051,#12299) ;
#8184=LINE('',#100053,#12300) ;
#8185=LINE('',#100055,#12301) ;
#8186=LINE('',#100056,#12302) ;
#8187=LINE('',#100060,#12303) ;
#8188=LINE('',#100062,#12304) ;
#8189=LINE('',#100064,#12305) ;
#8190=LINE('',#100065,#12306) ;
#8191=LINE('',#100069,#12307) ;
#8192=LINE('',#100071,#12308) ;
#8193=LINE('',#100073,#12309) ;
#8194=LINE('',#100074,#12310) ;
#8195=LINE('',#100078,#12311) ;
#8196=LINE('',#100080,#12312) ;
#8197=LINE('',#100082,#12313) ;
#8198=LINE('',#100083,#12314) ;
#8199=LINE('',#100087,#12315) ;
#8200=LINE('',#100089,#12316) ;
#8201=LINE('',#100091,#12317) ;
#8202=LINE('',#100092,#12318) ;
#8203=LINE('',#100096,#12319) ;
#8204=LINE('',#100098,#12320) ;
#8205=LINE('',#100100,#12321) ;
#8206=LINE('',#100101,#12322) ;
#8207=LINE('',#100105,#12323) ;
#8208=LINE('',#100107,#12324) ;
#8209=LINE('',#100109,#12325) ;
#8210=LINE('',#100110,#12326) ;
#8211=LINE('',#100114,#12327) ;
#8212=LINE('',#100116,#12328) ;
#8213=LINE('',#100118,#12329) ;
#8214=LINE('',#100119,#12330) ;
#8215=LINE('',#100123,#12331) ;
#8216=LINE('',#100125,#12332) ;
#8217=LINE('',#100127,#12333) ;
#8218=LINE('',#100128,#12334) ;
#8219=LINE('',#100132,#12335) ;
#8220=LINE('',#100134,#12336) ;
#8221=LINE('',#100136,#12337) ;
#8222=LINE('',#100137,#12338) ;
#8223=LINE('',#100141,#12339) ;
#8224=LINE('',#100143,#12340) ;
#8225=LINE('',#100145,#12341) ;
#8226=LINE('',#100146,#12342) ;
#8227=LINE('',#100150,#12343) ;
#8228=LINE('',#100152,#12344) ;
#8229=LINE('',#100154,#12345) ;
#8230=LINE('',#100155,#12346) ;
#8231=LINE('',#100159,#12347) ;
#8232=LINE('',#100161,#12348) ;
#8233=LINE('',#100163,#12349) ;
#8234=LINE('',#100164,#12350) ;
#8235=LINE('',#100168,#12351) ;
#8236=LINE('',#100170,#12352) ;
#8237=LINE('',#100172,#12353) ;
#8238=LINE('',#100173,#12354) ;
#8239=LINE('',#100177,#12355) ;
#8240=LINE('',#100179,#12356) ;
#8241=LINE('',#100181,#12357) ;
#8242=LINE('',#100182,#12358) ;
#8243=LINE('',#100186,#12359) ;
#8244=LINE('',#100188,#12360) ;
#8245=LINE('',#100190,#12361) ;
#8246=LINE('',#100191,#12362) ;
#8247=LINE('',#100195,#12363) ;
#8248=LINE('',#100197,#12364) ;
#8249=LINE('',#100199,#12365) ;
#8250=LINE('',#100200,#12366) ;
#8251=LINE('',#100204,#12367) ;
#8252=LINE('',#100206,#12368) ;
#8253=LINE('',#100208,#12369) ;
#8254=LINE('',#100209,#12370) ;
#8255=LINE('',#100213,#12371) ;
#8256=LINE('',#100215,#12372) ;
#8257=LINE('',#100217,#12373) ;
#8258=LINE('',#100218,#12374) ;
#8259=LINE('',#100222,#12375) ;
#8260=LINE('',#100224,#12376) ;
#8261=LINE('',#100226,#12377) ;
#8262=LINE('',#100227,#12378) ;
#8263=LINE('',#100231,#12379) ;
#8264=LINE('',#100233,#12380) ;
#8265=LINE('',#100235,#12381) ;
#8266=LINE('',#100236,#12382) ;
#8267=LINE('',#100240,#12383) ;
#8268=LINE('',#100242,#12384) ;
#8269=LINE('',#100244,#12385) ;
#8270=LINE('',#100245,#12386) ;
#8271=LINE('',#100249,#12387) ;
#8272=LINE('',#100251,#12388) ;
#8273=LINE('',#100253,#12389) ;
#8274=LINE('',#100254,#12390) ;
#8275=LINE('',#100258,#12391) ;
#8276=LINE('',#100260,#12392) ;
#8277=LINE('',#100262,#12393) ;
#8278=LINE('',#100263,#12394) ;
#8279=LINE('',#100267,#12395) ;
#8280=LINE('',#100269,#12396) ;
#8281=LINE('',#100271,#12397) ;
#8282=LINE('',#100272,#12398) ;
#8283=LINE('',#100276,#12399) ;
#8284=LINE('',#100278,#12400) ;
#8285=LINE('',#100280,#12401) ;
#8286=LINE('',#100281,#12402) ;
#8287=LINE('',#100285,#12403) ;
#8288=LINE('',#100287,#12404) ;
#8289=LINE('',#100289,#12405) ;
#8290=LINE('',#100290,#12406) ;
#8291=LINE('',#100294,#12407) ;
#8292=LINE('',#100296,#12408) ;
#8293=LINE('',#100298,#12409) ;
#8294=LINE('',#100299,#12410) ;
#8295=LINE('',#100303,#12411) ;
#8296=LINE('',#100305,#12412) ;
#8297=LINE('',#100307,#12413) ;
#8298=LINE('',#100308,#12414) ;
#8299=LINE('',#100312,#12415) ;
#8300=LINE('',#100314,#12416) ;
#8301=LINE('',#100316,#12417) ;
#8302=LINE('',#100317,#12418) ;
#8303=LINE('',#100321,#12419) ;
#8304=LINE('',#100323,#12420) ;
#8305=LINE('',#100325,#12421) ;
#8306=LINE('',#100326,#12422) ;
#8307=LINE('',#100330,#12423) ;
#8308=LINE('',#100332,#12424) ;
#8309=LINE('',#100334,#12425) ;
#8310=LINE('',#100335,#12426) ;
#8311=LINE('',#100339,#12427) ;
#8312=LINE('',#100341,#12428) ;
#8313=LINE('',#100343,#12429) ;
#8314=LINE('',#100344,#12430) ;
#8315=LINE('',#100348,#12431) ;
#8316=LINE('',#100350,#12432) ;
#8317=LINE('',#100352,#12433) ;
#8318=LINE('',#100353,#12434) ;
#8319=LINE('',#100357,#12435) ;
#8320=LINE('',#100359,#12436) ;
#8321=LINE('',#100361,#12437) ;
#8322=LINE('',#100362,#12438) ;
#8323=LINE('',#100366,#12439) ;
#8324=LINE('',#100368,#12440) ;
#8325=LINE('',#100370,#12441) ;
#8326=LINE('',#100371,#12442) ;
#8327=LINE('',#100375,#12443) ;
#8328=LINE('',#100377,#12444) ;
#8329=LINE('',#100379,#12445) ;
#8330=LINE('',#100380,#12446) ;
#8331=LINE('',#100384,#12447) ;
#8332=LINE('',#100386,#12448) ;
#8333=LINE('',#100388,#12449) ;
#8334=LINE('',#100389,#12450) ;
#8335=LINE('',#100393,#12451) ;
#8336=LINE('',#100395,#12452) ;
#8337=LINE('',#100397,#12453) ;
#8338=LINE('',#100398,#12454) ;
#8339=LINE('',#100402,#12455) ;
#8340=LINE('',#100404,#12456) ;
#8341=LINE('',#100406,#12457) ;
#8342=LINE('',#100407,#12458) ;
#8343=LINE('',#100411,#12459) ;
#8344=LINE('',#100413,#12460) ;
#8345=LINE('',#100415,#12461) ;
#8346=LINE('',#100416,#12462) ;
#8347=LINE('',#100420,#12463) ;
#8348=LINE('',#100422,#12464) ;
#8349=LINE('',#100424,#12465) ;
#8350=LINE('',#100425,#12466) ;
#12012=VECTOR('',#76918,1.6) ;
#12013=VECTOR('',#76923,1.49999999999999) ;
#12014=VECTOR('',#76926,1.6) ;
#12015=VECTOR('',#76931,1.49999999999999) ;
#12016=VECTOR('',#76934,1.6) ;
#12017=VECTOR('',#76937,1000.) ;
#12018=VECTOR('',#76938,1000.) ;
#12019=VECTOR('',#76939,1000.) ;
#12020=VECTOR('',#76940,1000.) ;
#12021=VECTOR('',#76941,1000.) ;
#12022=VECTOR('',#76942,1000.) ;
#12023=VECTOR('',#76945,1000.) ;
#12024=VECTOR('',#76948,1000.) ;
#12025=VECTOR('',#76951,1000.) ;
#12026=VECTOR('',#76954,1000.) ;
#12027=VECTOR('',#76957,1000.) ;
#12028=VECTOR('',#76958,1000.) ;
#12029=VECTOR('',#76959,1000.) ;
#12030=VECTOR('',#76960,1000.) ;
#12031=VECTOR('',#76961,1000.) ;
#12032=VECTOR('',#76962,1000.) ;
#12033=VECTOR('',#76965,1000.) ;
#12034=VECTOR('',#76968,1000.) ;
#12035=VECTOR('',#76971,1000.) ;
#12036=VECTOR('',#76974,1000.) ;
#12037=VECTOR('',#76979,1000.) ;
#12038=VECTOR('',#76980,1000.) ;
#12039=VECTOR('',#76981,1000.) ;
#12040=VECTOR('',#76982,1000.) ;
#12041=VECTOR('',#76983,1000.) ;
#12042=VECTOR('',#76984,1000.) ;
#12043=VECTOR('',#76987,1000.) ;
#12044=VECTOR('',#76988,1000.) ;
#12045=VECTOR('',#76989,1000.) ;
#12046=VECTOR('',#76992,1000.) ;
#12047=VECTOR('',#76995,1000.) ;
#12048=VECTOR('',#76998,1000.) ;
#12049=VECTOR('',#77001,1000.) ;
#12050=VECTOR('',#77004,1000.) ;
#12051=VECTOR('',#77007,1000.) ;
#12052=VECTOR('',#77010,1000.) ;
#12053=VECTOR('',#77013,1000.) ;
#12054=VECTOR('',#77016,1000.) ;
#12055=VECTOR('',#77019,1000.) ;
#12056=VECTOR('',#77022,1000.) ;
#12057=VECTOR('',#77025,1000.) ;
#12058=VECTOR('',#77028,1000.) ;
#12059=VECTOR('',#77031,1000.) ;
#12060=VECTOR('',#77034,1000.) ;
#12061=VECTOR('',#77037,1000.) ;
#12062=VECTOR('',#77040,1000.) ;
#12063=VECTOR('',#77041,1000.) ;
#12064=VECTOR('',#77044,1000.) ;
#12065=VECTOR('',#77045,1000.) ;
#12066=VECTOR('',#77046,1000.) ;
#12067=VECTOR('',#77049,1000.) ;
#12068=VECTOR('',#77050,1000.) ;
#12069=VECTOR('',#77051,1000.) ;
#12070=VECTOR('',#77052,1000.) ;
#12071=VECTOR('',#77055,1000.) ;
#12072=VECTOR('',#77058,1000.) ;
#12073=VECTOR('',#77061,1000.) ;
#12074=VECTOR('',#77064,1000.) ;
#12075=VECTOR('',#77067,1000.) ;
#12076=VECTOR('',#77070,1000.) ;
#12077=VECTOR('',#77073,1000.) ;
#12078=VECTOR('',#77076,1000.) ;
#12079=VECTOR('',#77079,1000.) ;
#12080=VECTOR('',#77082,1000.) ;
#12081=VECTOR('',#77085,1000.) ;
#12082=VECTOR('',#77088,1000.) ;
#12083=VECTOR('',#77091,1000.) ;
#12084=VECTOR('',#77094,1000.) ;
#12085=VECTOR('',#77097,1000.) ;
#12086=VECTOR('',#77100,1000.) ;
#12087=VECTOR('',#77103,1000.) ;
#12088=VECTOR('',#77104,1000.) ;
#12089=VECTOR('',#77107,1000.) ;
#12090=VECTOR('',#77108,1000.) ;
#12091=VECTOR('',#77109,1000.) ;
#12092=VECTOR('',#77112,1000.) ;
#12093=VECTOR('',#77113,1000.) ;
#12094=VECTOR('',#77114,1000.) ;
#12095=VECTOR('',#77115,1000.) ;
#12096=VECTOR('',#77118,1000.) ;
#12097=VECTOR('',#77121,1000.) ;
#12098=VECTOR('',#77124,1000.) ;
#12099=VECTOR('',#77127,1000.) ;
#12100=VECTOR('',#77130,1000.) ;
#12101=VECTOR('',#77133,1000.) ;
#12102=VECTOR('',#77136,1000.) ;
#12103=VECTOR('',#77139,1000.) ;
#12104=VECTOR('',#77142,1000.) ;
#12105=VECTOR('',#77145,1000.) ;
#12106=VECTOR('',#77148,1000.) ;
#12107=VECTOR('',#77151,1000.) ;
#12108=VECTOR('',#77154,1000.) ;
#12109=VECTOR('',#77157,1000.) ;
#12110=VECTOR('',#77160,1000.) ;
#12111=VECTOR('',#77163,1000.) ;
#12112=VECTOR('',#77166,1000.) ;
#12113=VECTOR('',#77169,1000.) ;
#12114=VECTOR('',#77172,1000.) ;
#12115=VECTOR('',#77175,1000.) ;
#12116=VECTOR('',#77178,1000.) ;
#12117=VECTOR('',#77181,1000.) ;
#12118=VECTOR('',#77184,1000.) ;
#12119=VECTOR('',#77187,1000.) ;
#12120=VECTOR('',#77190,1000.) ;
#12121=VECTOR('',#77193,1000.) ;
#12122=VECTOR('',#77196,1000.) ;
#12123=VECTOR('',#77199,1000.) ;
#12124=VECTOR('',#77204,1000.) ;
#12125=VECTOR('',#77205,1000.) ;
#12126=VECTOR('',#77206,1000.) ;
#12127=VECTOR('',#77207,1000.) ;
#12128=VECTOR('',#77208,1000.) ;
#12129=VECTOR('',#77209,1000.) ;
#12130=VECTOR('',#77212,1000.) ;
#12131=VECTOR('',#77213,1000.) ;
#12132=VECTOR('',#77214,1000.) ;
#12133=VECTOR('',#77217,1000.) ;
#12134=VECTOR('',#77220,1000.) ;
#12135=VECTOR('',#77223,1000.) ;
#12136=VECTOR('',#77226,1000.) ;
#12137=VECTOR('',#77229,1000.) ;
#12138=VECTOR('',#77232,1000.) ;
#12139=VECTOR('',#77235,1000.) ;
#12140=VECTOR('',#77238,1000.) ;
#12141=VECTOR('',#77241,1000.) ;
#12142=VECTOR('',#77244,1000.) ;
#12143=VECTOR('',#77247,1000.) ;
#12144=VECTOR('',#77250,1000.) ;
#12145=VECTOR('',#77253,1000.) ;
#12146=VECTOR('',#77256,1000.) ;
#12147=VECTOR('',#77259,1000.) ;
#12148=VECTOR('',#77262,1000.) ;
#12149=VECTOR('',#77265,1000.) ;
#12150=VECTOR('',#77268,1000.) ;
#12151=VECTOR('',#77271,1000.) ;
#12152=VECTOR('',#77274,1000.) ;
#12153=VECTOR('',#77277,1000.) ;
#12154=VECTOR('',#77280,1000.) ;
#12155=VECTOR('',#77283,1000.) ;
#12156=VECTOR('',#77286,1000.) ;
#12157=VECTOR('',#77289,1000.) ;
#12158=VECTOR('',#77292,1000.) ;
#12159=VECTOR('',#77295,1000.) ;
#12160=VECTOR('',#77298,1000.) ;
#12161=VECTOR('',#77303,1000.) ;
#12162=VECTOR('',#77304,1000.) ;
#12163=VECTOR('',#77305,1000.) ;
#12164=VECTOR('',#77306,1000.) ;
#12165=VECTOR('',#77307,1000.) ;
#12166=VECTOR('',#77310,1000.) ;
#12167=VECTOR('',#77311,1000.) ;
#12168=VECTOR('',#77312,1000.) ;
#12169=VECTOR('',#77315,1000.) ;
#12170=VECTOR('',#77316,1000.) ;
#12171=VECTOR('',#77319,1000.) ;
#12172=VECTOR('',#77320,1000.) ;
#12173=VECTOR('',#77321,1000.) ;
#12174=VECTOR('',#77324,1000.) ;
#12175=VECTOR('',#77325,1000.) ;
#12176=VECTOR('',#77326,1000.) ;
#12177=VECTOR('',#77329,1000.) ;
#12178=VECTOR('',#77330,1000.) ;
#12179=VECTOR('',#77331,1000.) ;
#12180=VECTOR('',#77332,1000.) ;
#12181=VECTOR('',#77335,1000.) ;
#12182=VECTOR('',#77336,1000.) ;
#12183=VECTOR('',#77337,1000.) ;
#12184=VECTOR('',#77338,1000.) ;
#12185=VECTOR('',#77341,1000.) ;
#12186=VECTOR('',#77342,1000.) ;
#12187=VECTOR('',#77343,1000.) ;
#12188=VECTOR('',#77344,1000.) ;
#12189=VECTOR('',#77347,1000.) ;
#12190=VECTOR('',#77348,1000.) ;
#12191=VECTOR('',#77349,1000.) ;
#12192=VECTOR('',#77350,1000.) ;
#12193=VECTOR('',#77353,1000.) ;
#12194=VECTOR('',#77354,1000.) ;
#12195=VECTOR('',#77355,1000.) ;
#12196=VECTOR('',#77356,1000.) ;
#12197=VECTOR('',#77361,1000.) ;
#12198=VECTOR('',#77368,1000.) ;
#12199=VECTOR('',#77371,1000.) ;
#12200=VECTOR('',#77382,1000.) ;
#12201=VECTOR('',#77383,1000.) ;
#12202=VECTOR('',#77384,1000.) ;
#12203=VECTOR('',#77385,1000.) ;
#12204=VECTOR('',#77388,1000.) ;
#12205=VECTOR('',#77389,1000.) ;
#12206=VECTOR('',#77390,1000.) ;
#12207=VECTOR('',#77391,1000.) ;
#12208=VECTOR('',#77394,1000.) ;
#12209=VECTOR('',#77395,1000.) ;
#12210=VECTOR('',#77396,1000.) ;
#12211=VECTOR('',#77397,1000.) ;
#12212=VECTOR('',#77400,1000.) ;
#12213=VECTOR('',#77401,1000.) ;
#12214=VECTOR('',#77402,1000.) ;
#12215=VECTOR('',#77403,1000.) ;
#12216=VECTOR('',#77406,1000.) ;
#12217=VECTOR('',#77407,1000.) ;
#12218=VECTOR('',#77408,1000.) ;
#12219=VECTOR('',#77409,1000.) ;
#12220=VECTOR('',#77412,1000.) ;
#12221=VECTOR('',#77413,1000.) ;
#12222=VECTOR('',#77414,1000.) ;
#12223=VECTOR('',#77415,1000.) ;
#12224=VECTOR('',#77418,1000.) ;
#12225=VECTOR('',#77419,1000.) ;
#12226=VECTOR('',#77420,1000.) ;
#12227=VECTOR('',#77423,1000.) ;
#12228=VECTOR('',#77426,1000.) ;
#12229=VECTOR('',#77427,1000.) ;
#12230=VECTOR('',#77428,1000.) ;
#12231=VECTOR('',#77429,1000.) ;
#12232=VECTOR('',#77432,1000.) ;
#12233=VECTOR('',#77433,1000.) ;
#12234=VECTOR('',#77434,1000.) ;
#12235=VECTOR('',#77435,1000.) ;
#12236=VECTOR('',#77438,1000.) ;
#12237=VECTOR('',#77439,1000.) ;
#12238=VECTOR('',#77440,1000.) ;
#12239=VECTOR('',#77441,1000.) ;
#12240=VECTOR('',#77444,1000.) ;
#12241=VECTOR('',#77445,1000.) ;
#12242=VECTOR('',#77448,1000.) ;
#12243=VECTOR('',#77449,1000.) ;
#12244=VECTOR('',#77454,1000.) ;
#12245=VECTOR('',#77469,1000.) ;
#12246=VECTOR('',#77478,1000.) ;
#12247=VECTOR('',#77491,1000.) ;
#12248=VECTOR('',#77492,1000.) ;
#12249=VECTOR('',#77493,1000.) ;
#12250=VECTOR('',#77494,1000.) ;
#12251=VECTOR('',#77497,1000.) ;
#12252=VECTOR('',#77498,1000.) ;
#12253=VECTOR('',#77499,1000.) ;
#12254=VECTOR('',#77500,1000.) ;
#12255=VECTOR('',#77503,1000.) ;
#12256=VECTOR('',#77504,1000.) ;
#12257=VECTOR('',#77505,1000.) ;
#12258=VECTOR('',#77506,1000.) ;
#12259=VECTOR('',#77509,1000.) ;
#12260=VECTOR('',#77510,1000.) ;
#12261=VECTOR('',#77511,1000.) ;
#12262=VECTOR('',#77512,1000.) ;
#12263=VECTOR('',#77515,1000.) ;
#12264=VECTOR('',#77516,1000.) ;
#12265=VECTOR('',#77517,1000.) ;
#12266=VECTOR('',#77518,1000.) ;
#12267=VECTOR('',#77521,1000.) ;
#12268=VECTOR('',#77522,1000.) ;
#12269=VECTOR('',#77523,1000.) ;
#12270=VECTOR('',#77524,1000.) ;
#12271=VECTOR('',#77527,1000.) ;
#12272=VECTOR('',#77530,1000.) ;
#12273=VECTOR('',#77531,1000.) ;
#12274=VECTOR('',#77532,1000.) ;
#12275=VECTOR('',#77535,1000.) ;
#12276=VECTOR('',#77536,1000.) ;
#12277=VECTOR('',#77537,1000.) ;
#12278=VECTOR('',#77538,1000.) ;
#12279=VECTOR('',#77541,1000.) ;
#12280=VECTOR('',#77542,1000.) ;
#12281=VECTOR('',#77543,1000.) ;
#12282=VECTOR('',#77544,1000.) ;
#12283=VECTOR('',#77547,1000.) ;
#12284=VECTOR('',#77548,1000.) ;
#12285=VECTOR('',#77549,1000.) ;
#12286=VECTOR('',#77550,1000.) ;
#12287=VECTOR('',#77553,1000.) ;
#12288=VECTOR('',#77554,1000.) ;
#12289=VECTOR('',#77555,1000.) ;
#12290=VECTOR('',#77556,1000.) ;
#12291=VECTOR('',#77559,1000.) ;
#12292=VECTOR('',#77560,1000.) ;
#12293=VECTOR('',#77561,1000.) ;
#12294=VECTOR('',#77562,1000.) ;
#12295=VECTOR('',#77565,1000.) ;
#12296=VECTOR('',#77566,1000.) ;
#12297=VECTOR('',#77567,1000.) ;
#12298=VECTOR('',#77568,1000.) ;
#12299=VECTOR('',#77571,1000.) ;
#12300=VECTOR('',#77572,1000.) ;
#12301=VECTOR('',#77573,1000.) ;
#12302=VECTOR('',#77574,1000.) ;
#12303=VECTOR('',#77577,1000.) ;
#12304=VECTOR('',#77578,1000.) ;
#12305=VECTOR('',#77579,1000.) ;
#12306=VECTOR('',#77580,1000.) ;
#12307=VECTOR('',#77583,1000.) ;
#12308=VECTOR('',#77584,1000.) ;
#12309=VECTOR('',#77585,1000.) ;
#12310=VECTOR('',#77586,1000.) ;
#12311=VECTOR('',#77589,1000.) ;
#12312=VECTOR('',#77590,1000.) ;
#12313=VECTOR('',#77591,1000.) ;
#12314=VECTOR('',#77592,1000.) ;
#12315=VECTOR('',#77595,1000.) ;
#12316=VECTOR('',#77596,1000.) ;
#12317=VECTOR('',#77597,1000.) ;
#12318=VECTOR('',#77598,1000.) ;
#12319=VECTOR('',#77601,1000.) ;
#12320=VECTOR('',#77602,1000.) ;
#12321=VECTOR('',#77603,1000.) ;
#12322=VECTOR('',#77604,1000.) ;
#12323=VECTOR('',#77607,1000.) ;
#12324=VECTOR('',#77608,1000.) ;
#12325=VECTOR('',#77609,1000.) ;
#12326=VECTOR('',#77610,1000.) ;
#12327=VECTOR('',#77613,1000.) ;
#12328=VECTOR('',#77614,1000.) ;
#12329=VECTOR('',#77615,1000.) ;
#12330=VECTOR('',#77616,1000.) ;
#12331=VECTOR('',#77619,1000.) ;
#12332=VECTOR('',#77620,1000.) ;
#12333=VECTOR('',#77621,1000.) ;
#12334=VECTOR('',#77622,1000.) ;
#12335=VECTOR('',#77625,1000.) ;
#12336=VECTOR('',#77626,1000.) ;
#12337=VECTOR('',#77627,1000.) ;
#12338=VECTOR('',#77628,1000.) ;
#12339=VECTOR('',#77631,1000.) ;
#12340=VECTOR('',#77632,1000.) ;
#12341=VECTOR('',#77633,1000.) ;
#12342=VECTOR('',#77634,1000.) ;
#12343=VECTOR('',#77637,1000.) ;
#12344=VECTOR('',#77638,1000.) ;
#12345=VECTOR('',#77639,1000.) ;
#12346=VECTOR('',#77640,1000.) ;
#12347=VECTOR('',#77643,1000.) ;
#12348=VECTOR('',#77644,1000.) ;
#12349=VECTOR('',#77645,1000.) ;
#12350=VECTOR('',#77646,1000.) ;
#12351=VECTOR('',#77649,1000.) ;
#12352=VECTOR('',#77650,1000.) ;
#12353=VECTOR('',#77651,1000.) ;
#12354=VECTOR('',#77652,1000.) ;
#12355=VECTOR('',#77655,1000.) ;
#12356=VECTOR('',#77656,1000.) ;
#12357=VECTOR('',#77657,1000.) ;
#12358=VECTOR('',#77658,1000.) ;
#12359=VECTOR('',#77661,1000.) ;
#12360=VECTOR('',#77662,1000.) ;
#12361=VECTOR('',#77663,1000.) ;
#12362=VECTOR('',#77664,1000.) ;
#12363=VECTOR('',#77667,1000.) ;
#12364=VECTOR('',#77668,1000.) ;
#12365=VECTOR('',#77669,1000.) ;
#12366=VECTOR('',#77670,1000.) ;
#12367=VECTOR('',#77673,1000.) ;
#12368=VECTOR('',#77674,1000.) ;
#12369=VECTOR('',#77675,1000.) ;
#12370=VECTOR('',#77676,1000.) ;
#12371=VECTOR('',#77679,1000.) ;
#12372=VECTOR('',#77680,1000.) ;
#12373=VECTOR('',#77681,1000.) ;
#12374=VECTOR('',#77682,1000.) ;
#12375=VECTOR('',#77685,1000.) ;
#12376=VECTOR('',#77686,1000.) ;
#12377=VECTOR('',#77687,1000.) ;
#12378=VECTOR('',#77688,1000.) ;
#12379=VECTOR('',#77691,1000.) ;
#12380=VECTOR('',#77692,1000.) ;
#12381=VECTOR('',#77693,1000.) ;
#12382=VECTOR('',#77694,1000.) ;
#12383=VECTOR('',#77697,1000.) ;
#12384=VECTOR('',#77698,1000.) ;
#12385=VECTOR('',#77699,1000.) ;
#12386=VECTOR('',#77700,1000.) ;
#12387=VECTOR('',#77703,1000.) ;
#12388=VECTOR('',#77704,1000.) ;
#12389=VECTOR('',#77705,1000.) ;
#12390=VECTOR('',#77706,1000.) ;
#12391=VECTOR('',#77709,1000.) ;
#12392=VECTOR('',#77710,1000.) ;
#12393=VECTOR('',#77711,1000.) ;
#12394=VECTOR('',#77712,1000.) ;
#12395=VECTOR('',#77715,1000.) ;
#12396=VECTOR('',#77716,1000.) ;
#12397=VECTOR('',#77717,1000.) ;
#12398=VECTOR('',#77718,1000.) ;
#12399=VECTOR('',#77721,1000.) ;
#12400=VECTOR('',#77722,1000.) ;
#12401=VECTOR('',#77723,1000.) ;
#12402=VECTOR('',#77724,1000.) ;
#12403=VECTOR('',#77727,1000.) ;
#12404=VECTOR('',#77728,1000.) ;
#12405=VECTOR('',#77729,1000.) ;
#12406=VECTOR('',#77730,1000.) ;
#12407=VECTOR('',#77733,1000.) ;
#12408=VECTOR('',#77734,1000.) ;
#12409=VECTOR('',#77735,1000.) ;
#12410=VECTOR('',#77736,1000.) ;
#12411=VECTOR('',#77739,1000.) ;
#12412=VECTOR('',#77740,1000.) ;
#12413=VECTOR('',#77741,1000.) ;
#12414=VECTOR('',#77742,1000.) ;
#12415=VECTOR('',#77745,1000.) ;
#12416=VECTOR('',#77746,1000.) ;
#12417=VECTOR('',#77747,1000.) ;
#12418=VECTOR('',#77748,1000.) ;
#12419=VECTOR('',#77751,1000.) ;
#12420=VECTOR('',#77752,1000.) ;
#12421=VECTOR('',#77753,1000.) ;
#12422=VECTOR('',#77754,1000.) ;
#12423=VECTOR('',#77757,1000.) ;
#12424=VECTOR('',#77758,1000.) ;
#12425=VECTOR('',#77759,1000.) ;
#12426=VECTOR('',#77760,1000.) ;
#12427=VECTOR('',#77763,1000.) ;
#12428=VECTOR('',#77764,1000.) ;
#12429=VECTOR('',#77765,1000.) ;
#12430=VECTOR('',#77766,1000.) ;
#12431=VECTOR('',#77769,1000.) ;
#12432=VECTOR('',#77770,1000.) ;
#12433=VECTOR('',#77771,1000.) ;
#12434=VECTOR('',#77772,1000.) ;
#12435=VECTOR('',#77775,1000.) ;
#12436=VECTOR('',#77776,1000.) ;
#12437=VECTOR('',#77777,1000.) ;
#12438=VECTOR('',#77778,1000.) ;
#12439=VECTOR('',#77781,1000.) ;
#12440=VECTOR('',#77782,1000.) ;
#12441=VECTOR('',#77783,1000.) ;
#12442=VECTOR('',#77784,1000.) ;
#12443=VECTOR('',#77787,1000.) ;
#12444=VECTOR('',#77788,1000.) ;
#12445=VECTOR('',#77789,1000.) ;
#12446=VECTOR('',#77790,1000.) ;
#12447=VECTOR('',#77793,1000.) ;
#12448=VECTOR('',#77794,1000.) ;
#12449=VECTOR('',#77795,1000.) ;
#12450=VECTOR('',#77796,1000.) ;
#12451=VECTOR('',#77799,1000.) ;
#12452=VECTOR('',#77800,1000.) ;
#12453=VECTOR('',#77801,1000.) ;
#12454=VECTOR('',#77802,1000.) ;
#12455=VECTOR('',#77805,1000.) ;
#12456=VECTOR('',#77806,1000.) ;
#12457=VECTOR('',#77807,1000.) ;
#12458=VECTOR('',#77808,1000.) ;
#12459=VECTOR('',#77811,1000.) ;
#12460=VECTOR('',#77812,1000.) ;
#12461=VECTOR('',#77813,1000.) ;
#12462=VECTOR('',#77814,1000.) ;
#12463=VECTOR('',#77817,1000.) ;
#12464=VECTOR('',#77818,1000.) ;
#12465=VECTOR('',#77819,1000.) ;
#12466=VECTOR('',#77820,1000.) ;
#16128=CONICAL_SURFACE('',#67795,1.6,0.785398163397431) ;
#16129=CONICAL_SURFACE('',#67798,1.6,0.785398163397431) ;
#16159=FACE_OUTER_BOUND('',#20401,.T.) ;
#16160=FACE_OUTER_BOUND('',#20402,.T.) ;
#16161=FACE_OUTER_BOUND('',#20403,.T.) ;
#16162=FACE_OUTER_BOUND('',#20404,.T.) ;
#16163=FACE_OUTER_BOUND('',#20405,.T.) ;
#16164=FACE_OUTER_BOUND('',#20406,.T.) ;
#16165=FACE_OUTER_BOUND('',#20407,.T.) ;
#16166=FACE_OUTER_BOUND('',#20408,.T.) ;
#16167=FACE_OUTER_BOUND('',#20409,.T.) ;
#16168=FACE_OUTER_BOUND('',#20410,.T.) ;
#16169=FACE_OUTER_BOUND('',#20411,.T.) ;
#16170=FACE_OUTER_BOUND('',#20412,.T.) ;
#16171=FACE_OUTER_BOUND('',#20415,.T.) ;
#16172=FACE_OUTER_BOUND('',#20418,.T.) ;
#16173=FACE_OUTER_BOUND('',#20423,.T.) ;
#16174=FACE_OUTER_BOUND('',#20428,.T.) ;
#16175=FACE_OUTER_BOUND('',#20436,.T.) ;
#16176=FACE_OUTER_BOUND('',#20444,.T.) ;
#16177=FACE_OUTER_BOUND('',#20447,.T.) ;
#16178=FACE_OUTER_BOUND('',#20450,.T.) ;
#16179=FACE_OUTER_BOUND('',#20451,.T.) ;
#16180=FACE_OUTER_BOUND('',#20452,.T.) ;
#16181=FACE_OUTER_BOUND('',#20453,.T.) ;
#16182=FACE_OUTER_BOUND('',#20454,.T.) ;
#16183=FACE_OUTER_BOUND('',#20455,.T.) ;
#16184=FACE_OUTER_BOUND('',#20456,.T.) ;
#16185=FACE_OUTER_BOUND('',#20457,.T.) ;
#16186=FACE_OUTER_BOUND('',#20458,.T.) ;
#16187=FACE_OUTER_BOUND('',#20459,.T.) ;
#16188=FACE_OUTER_BOUND('',#20460,.T.) ;
#16189=FACE_OUTER_BOUND('',#20461,.T.) ;
#16190=FACE_OUTER_BOUND('',#20462,.T.) ;
#16191=FACE_OUTER_BOUND('',#20463,.T.) ;
#16192=FACE_OUTER_BOUND('',#20464,.T.) ;
#16193=FACE_OUTER_BOUND('',#20465,.T.) ;
#16194=FACE_OUTER_BOUND('',#20466,.T.) ;
#16195=FACE_OUTER_BOUND('',#20467,.T.) ;
#16196=FACE_OUTER_BOUND('',#20468,.T.) ;
#16197=FACE_OUTER_BOUND('',#20469,.T.) ;
#16198=FACE_OUTER_BOUND('',#20470,.T.) ;
#16199=FACE_OUTER_BOUND('',#20471,.T.) ;
#16200=FACE_OUTER_BOUND('',#20472,.T.) ;
#16201=FACE_OUTER_BOUND('',#20473,.T.) ;
#16202=FACE_OUTER_BOUND('',#20474,.T.) ;
#16203=FACE_OUTER_BOUND('',#20475,.T.) ;
#16204=FACE_OUTER_BOUND('',#20476,.T.) ;
#16205=FACE_OUTER_BOUND('',#20477,.T.) ;
#16206=FACE_OUTER_BOUND('',#20478,.T.) ;
#16207=FACE_OUTER_BOUND('',#20479,.T.) ;
#16208=FACE_OUTER_BOUND('',#20480,.T.) ;
#16209=FACE_OUTER_BOUND('',#20481,.T.) ;
#16210=FACE_OUTER_BOUND('',#20482,.T.) ;
#16211=FACE_OUTER_BOUND('',#20483,.T.) ;
#16212=FACE_OUTER_BOUND('',#20484,.T.) ;
#16213=FACE_OUTER_BOUND('',#20485,.T.) ;
#16214=FACE_OUTER_BOUND('',#20486,.T.) ;
#16215=FACE_OUTER_BOUND('',#20487,.T.) ;
#16216=FACE_OUTER_BOUND('',#20488,.T.) ;
#16217=FACE_OUTER_BOUND('',#20489,.T.) ;
#16218=FACE_OUTER_BOUND('',#20490,.T.) ;
#16219=FACE_OUTER_BOUND('',#20491,.T.) ;
#16220=FACE_OUTER_BOUND('',#20492,.T.) ;
#16221=FACE_OUTER_BOUND('',#20493,.T.) ;
#16222=FACE_OUTER_BOUND('',#20494,.T.) ;
#16223=FACE_OUTER_BOUND('',#20495,.T.) ;
#16224=FACE_OUTER_BOUND('',#20496,.T.) ;
#16225=FACE_OUTER_BOUND('',#20497,.T.) ;
#16226=FACE_OUTER_BOUND('',#20498,.T.) ;
#16227=FACE_OUTER_BOUND('',#20499,.T.) ;
#16228=FACE_OUTER_BOUND('',#20500,.T.) ;
#16229=FACE_OUTER_BOUND('',#20501,.T.) ;
#16230=FACE_OUTER_BOUND('',#20502,.T.) ;
#16231=FACE_OUTER_BOUND('',#20503,.T.) ;
#16232=FACE_OUTER_BOUND('',#20504,.T.) ;
#16233=FACE_OUTER_BOUND('',#20505,.T.) ;
#16234=FACE_OUTER_BOUND('',#20506,.T.) ;
#16235=FACE_OUTER_BOUND('',#20507,.T.) ;
#16236=FACE_OUTER_BOUND('',#20508,.T.) ;
#16237=FACE_OUTER_BOUND('',#20509,.T.) ;
#16238=FACE_OUTER_BOUND('',#20510,.T.) ;
#16239=FACE_OUTER_BOUND('',#20511,.T.) ;
#16240=FACE_OUTER_BOUND('',#20512,.T.) ;
#16241=FACE_OUTER_BOUND('',#20513,.T.) ;
#16242=FACE_OUTER_BOUND('',#20514,.T.) ;
#16243=FACE_OUTER_BOUND('',#20515,.T.) ;
#16244=FACE_OUTER_BOUND('',#20516,.T.) ;
#16245=FACE_OUTER_BOUND('',#20517,.T.) ;
#16246=FACE_OUTER_BOUND('',#20518,.T.) ;
#16247=FACE_OUTER_BOUND('',#20519,.T.) ;
#16248=FACE_OUTER_BOUND('',#20520,.T.) ;
#16249=FACE_OUTER_BOUND('',#20521,.T.) ;
#16250=FACE_OUTER_BOUND('',#20522,.T.) ;
#16251=FACE_OUTER_BOUND('',#20523,.T.) ;
#16252=FACE_OUTER_BOUND('',#20524,.T.) ;
#16253=FACE_OUTER_BOUND('',#20525,.T.) ;
#16254=FACE_OUTER_BOUND('',#20526,.T.) ;
#16255=FACE_OUTER_BOUND('',#20527,.T.) ;
#16256=FACE_OUTER_BOUND('',#20528,.T.) ;
#16257=FACE_OUTER_BOUND('',#20529,.T.) ;
#16258=FACE_OUTER_BOUND('',#20530,.T.) ;
#16259=FACE_OUTER_BOUND('',#20531,.T.) ;
#16260=FACE_OUTER_BOUND('',#20532,.T.) ;
#16261=FACE_OUTER_BOUND('',#20533,.T.) ;
#16262=FACE_OUTER_BOUND('',#20534,.T.) ;
#16263=FACE_OUTER_BOUND('',#20535,.T.) ;
#16264=FACE_OUTER_BOUND('',#20536,.T.) ;
#16265=FACE_OUTER_BOUND('',#20537,.T.) ;
#16266=FACE_OUTER_BOUND('',#20538,.T.) ;
#16267=FACE_OUTER_BOUND('',#20539,.T.) ;
#16268=FACE_OUTER_BOUND('',#20540,.T.) ;
#16269=FACE_OUTER_BOUND('',#20541,.T.) ;
#16270=FACE_OUTER_BOUND('',#20542,.T.) ;
#16271=FACE_OUTER_BOUND('',#20543,.T.) ;
#16272=FACE_OUTER_BOUND('',#20544,.T.) ;
#16273=FACE_OUTER_BOUND('',#20545,.T.) ;
#16274=FACE_OUTER_BOUND('',#20546,.T.) ;
#16275=FACE_OUTER_BOUND('',#20547,.T.) ;
#16276=FACE_OUTER_BOUND('',#20548,.T.) ;
#16277=FACE_OUTER_BOUND('',#20549,.T.) ;
#16278=FACE_OUTER_BOUND('',#20550,.T.) ;
#16279=FACE_OUTER_BOUND('',#20551,.T.) ;
#16280=FACE_OUTER_BOUND('',#20552,.T.) ;
#16281=FACE_OUTER_BOUND('',#20553,.T.) ;
#16282=FACE_OUTER_BOUND('',#20554,.T.) ;
#16283=FACE_OUTER_BOUND('',#20555,.T.) ;
#16284=FACE_OUTER_BOUND('',#20556,.T.) ;
#16285=FACE_OUTER_BOUND('',#20557,.T.) ;
#16286=FACE_OUTER_BOUND('',#20558,.T.) ;
#16287=FACE_OUTER_BOUND('',#20559,.T.) ;
#16288=FACE_OUTER_BOUND('',#20560,.T.) ;
#16289=FACE_OUTER_BOUND('',#20561,.T.) ;
#16290=FACE_OUTER_BOUND('',#20562,.T.) ;
#16291=FACE_OUTER_BOUND('',#20563,.T.) ;
#16292=FACE_OUTER_BOUND('',#20564,.T.) ;
#16293=FACE_OUTER_BOUND('',#20565,.T.) ;
#16294=FACE_OUTER_BOUND('',#20566,.T.) ;
#16295=FACE_OUTER_BOUND('',#20567,.T.) ;
#16296=FACE_OUTER_BOUND('',#20568,.T.) ;
#16297=FACE_OUTER_BOUND('',#20569,.T.) ;
#16298=FACE_OUTER_BOUND('',#20570,.T.) ;
#16299=FACE_OUTER_BOUND('',#20571,.T.) ;
#16300=FACE_OUTER_BOUND('',#20572,.T.) ;
#16301=FACE_OUTER_BOUND('',#20573,.T.) ;
#16302=FACE_OUTER_BOUND('',#20574,.T.) ;
#16303=FACE_OUTER_BOUND('',#20575,.T.) ;
#16304=FACE_OUTER_BOUND('',#20576,.T.) ;
#16305=FACE_OUTER_BOUND('',#20577,.T.) ;
#16306=FACE_OUTER_BOUND('',#20578,.T.) ;
#16307=FACE_OUTER_BOUND('',#20579,.T.) ;
#16308=FACE_OUTER_BOUND('',#20580,.T.) ;
#16309=FACE_OUTER_BOUND('',#20581,.T.) ;
#16310=FACE_OUTER_BOUND('',#20582,.T.) ;
#16311=FACE_OUTER_BOUND('',#20583,.T.) ;
#16312=FACE_OUTER_BOUND('',#20584,.T.) ;
#16313=FACE_OUTER_BOUND('',#20585,.T.) ;
#16314=FACE_OUTER_BOUND('',#20586,.T.) ;
#16315=FACE_OUTER_BOUND('',#20587,.T.) ;
#16316=FACE_OUTER_BOUND('',#20588,.T.) ;
#16317=FACE_OUTER_BOUND('',#20589,.T.) ;
#16318=FACE_OUTER_BOUND('',#20590,.T.) ;
#16319=FACE_OUTER_BOUND('',#20591,.T.) ;
#16320=FACE_OUTER_BOUND('',#20592,.T.) ;
#16321=FACE_OUTER_BOUND('',#20593,.T.) ;
#16322=FACE_OUTER_BOUND('',#20594,.T.) ;
#16323=FACE_OUTER_BOUND('',#20595,.T.) ;
#16324=FACE_OUTER_BOUND('',#20596,.T.) ;
#16325=FACE_OUTER_BOUND('',#20597,.T.) ;
#16326=FACE_OUTER_BOUND('',#20598,.T.) ;
#16327=FACE_OUTER_BOUND('',#20599,.T.) ;
#16328=FACE_OUTER_BOUND('',#20600,.T.) ;
#16329=FACE_OUTER_BOUND('',#20601,.T.) ;
#16330=FACE_OUTER_BOUND('',#20602,.T.) ;
#16331=FACE_OUTER_BOUND('',#20603,.T.) ;
#16332=FACE_OUTER_BOUND('',#20604,.T.) ;
#16333=FACE_OUTER_BOUND('',#20605,.T.) ;
#16334=FACE_OUTER_BOUND('',#20606,.T.) ;
#16335=FACE_OUTER_BOUND('',#20607,.T.) ;
#16336=FACE_OUTER_BOUND('',#20608,.T.) ;
#16337=FACE_OUTER_BOUND('',#20609,.T.) ;
#16338=FACE_OUTER_BOUND('',#20610,.T.) ;
#16339=FACE_OUTER_BOUND('',#20611,.T.) ;
#16340=FACE_OUTER_BOUND('',#20612,.T.) ;
#16341=FACE_OUTER_BOUND('',#20613,.T.) ;
#16342=FACE_OUTER_BOUND('',#20614,.T.) ;
#16343=FACE_OUTER_BOUND('',#20615,.T.) ;
#16344=FACE_OUTER_BOUND('',#20616,.T.) ;
#16345=FACE_OUTER_BOUND('',#20617,.T.) ;
#16346=FACE_OUTER_BOUND('',#20618,.T.) ;
#16347=FACE_OUTER_BOUND('',#20619,.T.) ;
#16348=FACE_OUTER_BOUND('',#20620,.T.) ;
#16349=FACE_OUTER_BOUND('',#20621,.T.) ;
#16350=FACE_OUTER_BOUND('',#20622,.T.) ;
#16351=FACE_OUTER_BOUND('',#20623,.T.) ;
#16352=FACE_OUTER_BOUND('',#20624,.T.) ;
#16353=FACE_OUTER_BOUND('',#20625,.T.) ;
#16354=FACE_OUTER_BOUND('',#20626,.T.) ;
#16355=FACE_OUTER_BOUND('',#20627,.T.) ;
#16356=FACE_OUTER_BOUND('',#20628,.T.) ;
#16357=FACE_OUTER_BOUND('',#20629,.T.) ;
#16358=FACE_OUTER_BOUND('',#20630,.T.) ;
#16359=FACE_OUTER_BOUND('',#20631,.T.) ;
#16360=FACE_OUTER_BOUND('',#20632,.T.) ;
#16361=FACE_OUTER_BOUND('',#20633,.T.) ;
#16362=FACE_OUTER_BOUND('',#20634,.T.) ;
#16363=FACE_OUTER_BOUND('',#20635,.T.) ;
#16364=FACE_OUTER_BOUND('',#20636,.T.) ;
#16365=FACE_OUTER_BOUND('',#20637,.T.) ;
#16366=FACE_OUTER_BOUND('',#20638,.T.) ;
#16367=FACE_OUTER_BOUND('',#20639,.T.) ;
#16368=FACE_OUTER_BOUND('',#20640,.T.) ;
#16369=FACE_OUTER_BOUND('',#20641,.T.) ;
#16370=FACE_OUTER_BOUND('',#20642,.T.) ;
#16371=FACE_OUTER_BOUND('',#20643,.T.) ;
#16372=FACE_OUTER_BOUND('',#20644,.T.) ;
#16373=FACE_OUTER_BOUND('',#20645,.T.) ;
#16374=FACE_OUTER_BOUND('',#20646,.T.) ;
#16375=FACE_OUTER_BOUND('',#20647,.T.) ;
#16376=FACE_OUTER_BOUND('',#20648,.T.) ;
#16377=FACE_OUTER_BOUND('',#20649,.T.) ;
#16378=FACE_OUTER_BOUND('',#20650,.T.) ;
#16379=FACE_OUTER_BOUND('',#20651,.T.) ;
#16380=FACE_OUTER_BOUND('',#20652,.T.) ;
#16381=FACE_OUTER_BOUND('',#20653,.T.) ;
#16382=FACE_OUTER_BOUND('',#20654,.T.) ;
#16383=FACE_OUTER_BOUND('',#20655,.T.) ;
#16384=FACE_OUTER_BOUND('',#20656,.T.) ;
#16385=FACE_OUTER_BOUND('',#20657,.T.) ;
#16386=FACE_OUTER_BOUND('',#20658,.T.) ;
#16387=FACE_OUTER_BOUND('',#20659,.T.) ;
#16388=FACE_OUTER_BOUND('',#20660,.T.) ;
#16389=FACE_OUTER_BOUND('',#20661,.T.) ;
#16390=FACE_OUTER_BOUND('',#20662,.T.) ;
#16391=FACE_OUTER_BOUND('',#20663,.T.) ;
#16392=FACE_OUTER_BOUND('',#20664,.T.) ;
#16393=FACE_OUTER_BOUND('',#20665,.T.) ;
#16394=FACE_OUTER_BOUND('',#20666,.T.) ;
#16395=FACE_OUTER_BOUND('',#20667,.T.) ;
#16396=FACE_OUTER_BOUND('',#20668,.T.) ;
#16397=FACE_OUTER_BOUND('',#20669,.T.) ;
#16398=FACE_OUTER_BOUND('',#20670,.T.) ;
#16399=FACE_OUTER_BOUND('',#20671,.T.) ;
#16400=FACE_OUTER_BOUND('',#20672,.T.) ;
#16401=FACE_OUTER_BOUND('',#20673,.T.) ;
#16402=FACE_OUTER_BOUND('',#20674,.T.) ;
#16403=FACE_OUTER_BOUND('',#20675,.T.) ;
#16404=FACE_OUTER_BOUND('',#20676,.T.) ;
#16405=FACE_OUTER_BOUND('',#20677,.T.) ;
#16406=FACE_OUTER_BOUND('',#20678,.T.) ;
#16407=FACE_OUTER_BOUND('',#20679,.T.) ;
#16408=FACE_OUTER_BOUND('',#20680,.T.) ;
#16409=FACE_OUTER_BOUND('',#20681,.T.) ;
#16410=FACE_OUTER_BOUND('',#20682,.T.) ;
#16411=FACE_OUTER_BOUND('',#20683,.T.) ;
#16412=FACE_OUTER_BOUND('',#20684,.T.) ;
#16413=FACE_OUTER_BOUND('',#20685,.T.) ;
#16414=FACE_OUTER_BOUND('',#20686,.T.) ;
#16415=FACE_OUTER_BOUND('',#20687,.T.) ;
#16416=FACE_OUTER_BOUND('',#20688,.T.) ;
#16417=FACE_OUTER_BOUND('',#20689,.T.) ;
#16418=FACE_OUTER_BOUND('',#20690,.T.) ;
#16419=FACE_OUTER_BOUND('',#20691,.T.) ;
#16420=FACE_OUTER_BOUND('',#20692,.T.) ;
#16421=FACE_OUTER_BOUND('',#20693,.T.) ;
#16422=FACE_OUTER_BOUND('',#20694,.T.) ;
#16423=FACE_OUTER_BOUND('',#20695,.T.) ;
#16424=FACE_OUTER_BOUND('',#20696,.T.) ;
#16425=FACE_OUTER_BOUND('',#20697,.T.) ;
#16426=FACE_OUTER_BOUND('',#20698,.T.) ;
#16427=FACE_OUTER_BOUND('',#20699,.T.) ;
#16428=FACE_OUTER_BOUND('',#20700,.T.) ;
#16429=FACE_OUTER_BOUND('',#20701,.T.) ;
#16430=FACE_OUTER_BOUND('',#20702,.T.) ;
#16431=FACE_OUTER_BOUND('',#20703,.T.) ;
#16432=FACE_OUTER_BOUND('',#20704,.T.) ;
#16433=FACE_OUTER_BOUND('',#20705,.T.) ;
#16434=FACE_OUTER_BOUND('',#20706,.T.) ;
#16435=FACE_OUTER_BOUND('',#20707,.T.) ;
#16436=FACE_OUTER_BOUND('',#20708,.T.) ;
#16437=FACE_OUTER_BOUND('',#20709,.T.) ;
#16438=FACE_OUTER_BOUND('',#20710,.T.) ;
#16439=FACE_OUTER_BOUND('',#20711,.T.) ;
#16440=FACE_OUTER_BOUND('',#20712,.T.) ;
#16441=FACE_OUTER_BOUND('',#20713,.T.) ;
#16442=FACE_OUTER_BOUND('',#20714,.T.) ;
#16443=FACE_OUTER_BOUND('',#20715,.T.) ;
#16444=FACE_OUTER_BOUND('',#20716,.T.) ;
#16445=FACE_OUTER_BOUND('',#20717,.T.) ;
#16446=FACE_OUTER_BOUND('',#20718,.T.) ;
#16447=FACE_OUTER_BOUND('',#20719,.T.) ;
#16448=FACE_OUTER_BOUND('',#20720,.T.) ;
#16449=FACE_OUTER_BOUND('',#20721,.T.) ;
#16450=FACE_OUTER_BOUND('',#20722,.T.) ;
#16451=FACE_OUTER_BOUND('',#20723,.T.) ;
#16452=FACE_OUTER_BOUND('',#20724,.T.) ;
#16453=FACE_OUTER_BOUND('',#20725,.T.) ;
#16454=FACE_OUTER_BOUND('',#20726,.T.) ;
#16455=FACE_OUTER_BOUND('',#20727,.T.) ;
#16456=FACE_OUTER_BOUND('',#20728,.T.) ;
#16457=FACE_OUTER_BOUND('',#20729,.T.) ;
#16458=FACE_OUTER_BOUND('',#20730,.T.) ;
#16459=FACE_OUTER_BOUND('',#20731,.T.) ;
#16460=FACE_OUTER_BOUND('',#20732,.T.) ;
#16461=FACE_OUTER_BOUND('',#20733,.T.) ;
#16462=FACE_OUTER_BOUND('',#20734,.T.) ;
#16463=FACE_OUTER_BOUND('',#20735,.T.) ;
#16464=FACE_OUTER_BOUND('',#20736,.T.) ;
#16465=FACE_OUTER_BOUND('',#20737,.T.) ;
#16466=FACE_OUTER_BOUND('',#20738,.T.) ;
#16467=FACE_OUTER_BOUND('',#20739,.T.) ;
#16468=FACE_OUTER_BOUND('',#20740,.T.) ;
#16469=FACE_OUTER_BOUND('',#20741,.T.) ;
#16470=FACE_OUTER_BOUND('',#20742,.T.) ;
#16471=FACE_OUTER_BOUND('',#20743,.T.) ;
#16472=FACE_OUTER_BOUND('',#20744,.T.) ;
#16473=FACE_OUTER_BOUND('',#20745,.T.) ;
#16474=FACE_OUTER_BOUND('',#20746,.T.) ;
#16475=FACE_OUTER_BOUND('',#20747,.T.) ;
#16476=FACE_OUTER_BOUND('',#20748,.T.) ;
#16477=FACE_OUTER_BOUND('',#20749,.T.) ;
#16478=FACE_OUTER_BOUND('',#20750,.T.) ;
#16479=FACE_OUTER_BOUND('',#20751,.T.) ;
#16480=FACE_OUTER_BOUND('',#20752,.T.) ;
#16481=FACE_OUTER_BOUND('',#20753,.T.) ;
#16482=FACE_OUTER_BOUND('',#20754,.T.) ;
#16483=FACE_OUTER_BOUND('',#20755,.T.) ;
#16484=FACE_OUTER_BOUND('',#20756,.T.) ;
#16485=FACE_OUTER_BOUND('',#20757,.T.) ;
#16486=FACE_OUTER_BOUND('',#20758,.T.) ;
#16487=FACE_OUTER_BOUND('',#20759,.T.) ;
#16488=FACE_OUTER_BOUND('',#20760,.T.) ;
#16489=FACE_OUTER_BOUND('',#20761,.T.) ;
#16490=FACE_OUTER_BOUND('',#20762,.T.) ;
#16491=FACE_OUTER_BOUND('',#20763,.T.) ;
#16492=FACE_OUTER_BOUND('',#20764,.T.) ;
#16493=FACE_OUTER_BOUND('',#20765,.T.) ;
#16494=FACE_OUTER_BOUND('',#20766,.T.) ;
#16495=FACE_OUTER_BOUND('',#20767,.T.) ;
#16496=FACE_OUTER_BOUND('',#20768,.T.) ;
#16497=FACE_OUTER_BOUND('',#20769,.T.) ;
#16498=FACE_OUTER_BOUND('',#20770,.T.) ;
#16499=FACE_OUTER_BOUND('',#20771,.T.) ;
#16500=FACE_OUTER_BOUND('',#20772,.T.) ;
#16501=FACE_OUTER_BOUND('',#20773,.T.) ;
#16502=FACE_OUTER_BOUND('',#20774,.T.) ;
#16503=FACE_OUTER_BOUND('',#20775,.T.) ;
#16504=FACE_OUTER_BOUND('',#20776,.T.) ;
#16505=FACE_OUTER_BOUND('',#20777,.T.) ;
#16506=FACE_OUTER_BOUND('',#20778,.T.) ;
#16507=FACE_OUTER_BOUND('',#20779,.T.) ;
#16508=FACE_OUTER_BOUND('',#20780,.T.) ;
#16509=FACE_OUTER_BOUND('',#20781,.T.) ;
#16510=FACE_OUTER_BOUND('',#20782,.T.) ;
#16511=FACE_OUTER_BOUND('',#20783,.T.) ;
#16512=FACE_OUTER_BOUND('',#20784,.T.) ;
#16513=FACE_OUTER_BOUND('',#20785,.T.) ;
#16514=FACE_OUTER_BOUND('',#20786,.T.) ;
#16515=FACE_OUTER_BOUND('',#20787,.T.) ;
#16516=FACE_OUTER_BOUND('',#20788,.T.) ;
#16517=FACE_OUTER_BOUND('',#20789,.T.) ;
#16518=FACE_OUTER_BOUND('',#20790,.T.) ;
#16519=FACE_OUTER_BOUND('',#20791,.T.) ;
#16520=FACE_OUTER_BOUND('',#20792,.T.) ;
#16521=FACE_OUTER_BOUND('',#20793,.T.) ;
#16522=FACE_OUTER_BOUND('',#20794,.T.) ;
#16523=FACE_OUTER_BOUND('',#20795,.T.) ;
#16524=FACE_OUTER_BOUND('',#20796,.T.) ;
#16525=FACE_OUTER_BOUND('',#20797,.T.) ;
#16526=FACE_OUTER_BOUND('',#20798,.T.) ;
#16527=FACE_OUTER_BOUND('',#20799,.T.) ;
#16528=FACE_OUTER_BOUND('',#20800,.T.) ;
#16529=FACE_OUTER_BOUND('',#20801,.T.) ;
#16530=FACE_OUTER_BOUND('',#20802,.T.) ;
#16531=FACE_OUTER_BOUND('',#20803,.T.) ;
#16532=FACE_OUTER_BOUND('',#20804,.T.) ;
#16533=FACE_OUTER_BOUND('',#20805,.T.) ;
#16534=FACE_OUTER_BOUND('',#20806,.T.) ;
#16535=FACE_OUTER_BOUND('',#20807,.T.) ;
#16536=FACE_OUTER_BOUND('',#20808,.T.) ;
#16537=FACE_OUTER_BOUND('',#20809,.T.) ;
#16538=FACE_OUTER_BOUND('',#20810,.T.) ;
#16539=FACE_OUTER_BOUND('',#20811,.T.) ;
#16540=FACE_OUTER_BOUND('',#20812,.T.) ;
#16541=FACE_OUTER_BOUND('',#20813,.T.) ;
#16542=FACE_OUTER_BOUND('',#20814,.T.) ;
#16543=FACE_OUTER_BOUND('',#20815,.T.) ;
#16544=FACE_OUTER_BOUND('',#20816,.T.) ;
#16545=FACE_OUTER_BOUND('',#20817,.T.) ;
#16546=FACE_OUTER_BOUND('',#20818,.T.) ;
#16547=FACE_OUTER_BOUND('',#20819,.T.) ;
#16548=FACE_OUTER_BOUND('',#20820,.T.) ;
#16549=FACE_OUTER_BOUND('',#20821,.T.) ;
#16550=FACE_OUTER_BOUND('',#20822,.T.) ;
#16551=FACE_OUTER_BOUND('',#20823,.T.) ;
#16552=FACE_OUTER_BOUND('',#20824,.T.) ;
#16553=FACE_OUTER_BOUND('',#20825,.T.) ;
#16554=FACE_OUTER_BOUND('',#20826,.T.) ;
#16555=FACE_OUTER_BOUND('',#20827,.T.) ;
#16556=FACE_OUTER_BOUND('',#20828,.T.) ;
#16557=FACE_OUTER_BOUND('',#20829,.T.) ;
#16558=FACE_OUTER_BOUND('',#20830,.T.) ;
#16559=FACE_OUTER_BOUND('',#20831,.T.) ;
#16560=FACE_OUTER_BOUND('',#20832,.T.) ;
#16561=FACE_OUTER_BOUND('',#20833,.T.) ;
#16562=FACE_OUTER_BOUND('',#20834,.T.) ;
#16563=FACE_OUTER_BOUND('',#20835,.T.) ;
#16564=FACE_OUTER_BOUND('',#20836,.T.) ;
#16565=FACE_OUTER_BOUND('',#20837,.T.) ;
#16566=FACE_OUTER_BOUND('',#20838,.T.) ;
#16567=FACE_OUTER_BOUND('',#20839,.T.) ;
#16568=FACE_OUTER_BOUND('',#20840,.T.) ;
#16569=FACE_OUTER_BOUND('',#20841,.T.) ;
#16570=FACE_OUTER_BOUND('',#20842,.T.) ;
#16571=FACE_OUTER_BOUND('',#20843,.T.) ;
#16572=FACE_OUTER_BOUND('',#20844,.T.) ;
#16573=FACE_OUTER_BOUND('',#20845,.T.) ;
#16574=FACE_OUTER_BOUND('',#20846,.T.) ;
#16575=FACE_OUTER_BOUND('',#20847,.T.) ;
#16576=FACE_OUTER_BOUND('',#20848,.T.) ;
#16577=FACE_OUTER_BOUND('',#20849,.T.) ;
#16578=FACE_OUTER_BOUND('',#20850,.T.) ;
#16579=FACE_OUTER_BOUND('',#20851,.T.) ;
#16580=FACE_OUTER_BOUND('',#20852,.T.) ;
#16581=FACE_OUTER_BOUND('',#20853,.T.) ;
#16582=FACE_OUTER_BOUND('',#20854,.T.) ;
#16583=FACE_OUTER_BOUND('',#20855,.T.) ;
#16584=FACE_OUTER_BOUND('',#20856,.T.) ;
#16585=FACE_OUTER_BOUND('',#20857,.T.) ;
#16586=FACE_OUTER_BOUND('',#20858,.T.) ;
#16587=FACE_OUTER_BOUND('',#20859,.T.) ;
#16588=FACE_OUTER_BOUND('',#20860,.T.) ;
#16589=FACE_OUTER_BOUND('',#20861,.T.) ;
#16590=FACE_OUTER_BOUND('',#20862,.T.) ;
#16591=FACE_OUTER_BOUND('',#20863,.T.) ;
#16592=FACE_OUTER_BOUND('',#20864,.T.) ;
#16593=FACE_OUTER_BOUND('',#20865,.T.) ;
#16594=FACE_OUTER_BOUND('',#20866,.T.) ;
#16595=FACE_OUTER_BOUND('',#20867,.T.) ;
#16596=FACE_OUTER_BOUND('',#20868,.T.) ;
#16597=FACE_OUTER_BOUND('',#20869,.T.) ;
#16598=FACE_OUTER_BOUND('',#20870,.T.) ;
#16599=FACE_OUTER_BOUND('',#20871,.T.) ;
#16600=FACE_OUTER_BOUND('',#20872,.T.) ;
#16601=FACE_OUTER_BOUND('',#20873,.T.) ;
#16602=FACE_OUTER_BOUND('',#20874,.T.) ;
#16603=FACE_OUTER_BOUND('',#20875,.T.) ;
#16604=FACE_OUTER_BOUND('',#20876,.T.) ;
#16605=FACE_OUTER_BOUND('',#20877,.T.) ;
#16606=FACE_OUTER_BOUND('',#20878,.T.) ;
#16607=FACE_OUTER_BOUND('',#20879,.T.) ;
#16608=FACE_OUTER_BOUND('',#20880,.T.) ;
#16609=FACE_OUTER_BOUND('',#20881,.T.) ;
#20401=EDGE_LOOP('',(#44066,#44067,#44068,#44069,#44070)) ;
#20402=EDGE_LOOP('',(#44071,#44072,#44073,#44074,#44075)) ;
#20403=EDGE_LOOP('',(#44076,#44077,#44078,#44079,#44080,#44081)) ;
#20404=EDGE_LOOP('',(#44082,#44083,#44084,#44085)) ;
#20405=EDGE_LOOP('',(#44086,#44087,#44088,#44089,#44090,#44091)) ;
#20406=EDGE_LOOP('',(#44092,#44093,#44094,#44095)) ;
#20407=EDGE_LOOP('',(#44096,#44097,#44098,#44099,#44100)) ;
#20408=EDGE_LOOP('',(#44101,#44102,#44103,#44104,#44105)) ;
#20409=EDGE_LOOP('',(#44106,#44107,#44108,#44109,#44110)) ;
#20410=EDGE_LOOP('',(#44111,#44112,#44113,#44114,#44115)) ;
#20411=EDGE_LOOP('',(#44116,#44117,#44118,#44119,#44120,#44121)) ;
#20412=EDGE_LOOP('',(#44122,#44123,#44124,#44125,#44126,#44127)) ;
#20413=EDGE_LOOP('',(#44128,#44129,#44130,#44131,#44132,#44133,#44134,#44135)) ;
#20414=EDGE_LOOP('',(#44136)) ;
#20415=EDGE_LOOP('',(#44137,#44138,#44139,#44140,#44141,#44142)) ;
#20416=EDGE_LOOP('',(#44143,#44144,#44145,#44146,#44147,#44148,#44149,#44150)) ;
#20417=EDGE_LOOP('',(#44151)) ;
#20418=EDGE_LOOP('',(#44152,#44153,#44154,#44155,#44156,#44157,#44158,#44159,
#44160,#44161,#44162)) ;
#20419=EDGE_LOOP('',(#44163,#44164,#44165,#44166,#44167,#44168,#44169,#44170)) ;
#20420=EDGE_LOOP('',(#44171,#44172,#44173,#44174,#44175,#44176,#44177,#44178)) ;
#20421=EDGE_LOOP('',(#44179,#44180,#44181,#44182,#44183,#44184,#44185,#44186)) ;
#20422=EDGE_LOOP('',(#44187,#44188,#44189,#44190,#44191,#44192,#44193,#44194)) ;
#20423=EDGE_LOOP('',(#44195,#44196,#44197,#44198,#44199,#44200,#44201,#44202,
#44203,#44204,#44205)) ;
#20424=EDGE_LOOP('',(#44206,#44207,#44208,#44209,#44210,#44211,#44212,#44213)) ;
#20425=EDGE_LOOP('',(#44214,#44215,#44216,#44217,#44218,#44219,#44220,#44221)) ;
#20426=EDGE_LOOP('',(#44222,#44223,#44224,#44225,#44226,#44227,#44228,#44229)) ;
#20427=EDGE_LOOP('',(#44230,#44231,#44232,#44233,#44234,#44235,#44236,#44237)) ;
#20428=EDGE_LOOP('',(#44238,#44239,#44240,#44241,#44242,#44243,#44244,#44245,
#44246,#44247,#44248)) ;
#20429=EDGE_LOOP('',(#44249,#44250,#44251,#44252,#44253,#44254,#44255,#44256)) ;
#20430=EDGE_LOOP('',(#44257,#44258,#44259,#44260,#44261,#44262,#44263,#44264)) ;
#20431=EDGE_LOOP('',(#44265,#44266,#44267,#44268,#44269,#44270,#44271,#44272)) ;
#20432=EDGE_LOOP('',(#44273,#44274,#44275,#44276,#44277,#44278,#44279,#44280)) ;
#20433=EDGE_LOOP('',(#44281,#44282,#44283,#44284,#44285,#44286,#44287,#44288)) ;
#20434=EDGE_LOOP('',(#44289,#44290,#44291,#44292,#44293,#44294,#44295,#44296)) ;
#20435=EDGE_LOOP('',(#44297,#44298,#44299,#44300,#44301,#44302,#44303,#44304)) ;
#20436=EDGE_LOOP('',(#44305,#44306,#44307,#44308,#44309,#44310,#44311,#44312,
#44313,#44314,#44315)) ;
#20437=EDGE_LOOP('',(#44316,#44317,#44318,#44319,#44320,#44321,#44322,#44323)) ;
#20438=EDGE_LOOP('',(#44324,#44325,#44326,#44327,#44328,#44329,#44330,#44331)) ;
#20439=EDGE_LOOP('',(#44332,#44333,#44334,#44335,#44336,#44337,#44338,#44339)) ;
#20440=EDGE_LOOP('',(#44340,#44341,#44342,#44343,#44344,#44345,#44346,#44347)) ;
#20441=EDGE_LOOP('',(#44348,#44349,#44350,#44351,#44352,#44353,#44354,#44355)) ;
#20442=EDGE_LOOP('',(#44356,#44357,#44358,#44359,#44360,#44361,#44362,#44363)) ;
#20443=EDGE_LOOP('',(#44364,#44365,#44366,#44367,#44368,#44369,#44370,#44371)) ;
#20444=EDGE_LOOP('',(#44372,#44373,#44374,#44375,#44376,#44377,#44378,#44379,
#44380,#44381)) ;
#20445=EDGE_LOOP('',(#44382)) ;
#20446=EDGE_LOOP('',(#44383)) ;
#20447=EDGE_LOOP('',(#44384,#44385,#44386,#44387,#44388,#44389,#44390,#44391,
#44392,#44393)) ;
#20448=EDGE_LOOP('',(#44394)) ;
#20449=EDGE_LOOP('',(#44395)) ;
#20450=EDGE_LOOP('',(#44396,#44397,#44398,#44399)) ;
#20451=EDGE_LOOP('',(#44400,#44401,#44402,#44403)) ;
#20452=EDGE_LOOP('',(#44404,#44405,#44406,#44407)) ;
#20453=EDGE_LOOP('',(#44408,#44409,#44410,#44411)) ;
#20454=EDGE_LOOP('',(#44412,#44413,#44414,#44415)) ;
#20455=EDGE_LOOP('',(#44416,#44417,#44418,#44419)) ;
#20456=EDGE_LOOP('',(#44420,#44421,#44422,#44423)) ;
#20457=EDGE_LOOP('',(#44424,#44425,#44426,#44427)) ;
#20458=EDGE_LOOP('',(#44428,#44429,#44430,#44431)) ;
#20459=EDGE_LOOP('',(#44432,#44433,#44434,#44435)) ;
#20460=EDGE_LOOP('',(#44436,#44437,#44438,#44439)) ;
#20461=EDGE_LOOP('',(#44440,#44441,#44442,#44443)) ;
#20462=EDGE_LOOP('',(#44444,#44445,#44446,#44447)) ;
#20463=EDGE_LOOP('',(#44448,#44449,#44450,#44451)) ;
#20464=EDGE_LOOP('',(#44452,#44453,#44454,#44455)) ;
#20465=EDGE_LOOP('',(#44456,#44457,#44458,#44459)) ;
#20466=EDGE_LOOP('',(#44460,#44461,#44462,#44463)) ;
#20467=EDGE_LOOP('',(#44464,#44465,#44466,#44467)) ;
#20468=EDGE_LOOP('',(#44468,#44469,#44470,#44471)) ;
#20469=EDGE_LOOP('',(#44472,#44473,#44474,#44475)) ;
#20470=EDGE_LOOP('',(#44476,#44477,#44478,#44479)) ;
#20471=EDGE_LOOP('',(#44480,#44481,#44482,#44483)) ;
#20472=EDGE_LOOP('',(#44484,#44485,#44486,#44487)) ;
#20473=EDGE_LOOP('',(#44488,#44489,#44490,#44491)) ;
#20474=EDGE_LOOP('',(#44492,#44493,#44494,#44495)) ;
#20475=EDGE_LOOP('',(#44496,#44497,#44498,#44499)) ;
#20476=EDGE_LOOP('',(#44500,#44501,#44502,#44503)) ;
#20477=EDGE_LOOP('',(#44504,#44505,#44506,#44507)) ;
#20478=EDGE_LOOP('',(#44508,#44509,#44510,#44511)) ;
#20479=EDGE_LOOP('',(#44512,#44513,#44514,#44515)) ;
#20480=EDGE_LOOP('',(#44516,#44517,#44518,#44519)) ;
#20481=EDGE_LOOP('',(#44520,#44521,#44522,#44523)) ;
#20482=EDGE_LOOP('',(#44524,#44525,#44526,#44527)) ;
#20483=EDGE_LOOP('',(#44528,#44529,#44530,#44531)) ;
#20484=EDGE_LOOP('',(#44532,#44533,#44534,#44535)) ;
#20485=EDGE_LOOP('',(#44536,#44537,#44538,#44539)) ;
#20486=EDGE_LOOP('',(#44540,#44541,#44542,#44543)) ;
#20487=EDGE_LOOP('',(#44544,#44545,#44546,#44547)) ;
#20488=EDGE_LOOP('',(#44548,#44549,#44550,#44551)) ;
#20489=EDGE_LOOP('',(#44552,#44553,#44554,#44555)) ;
#20490=EDGE_LOOP('',(#44556,#44557,#44558,#44559)) ;
#20491=EDGE_LOOP('',(#44560,#44561,#44562,#44563)) ;
#20492=EDGE_LOOP('',(#44564,#44565,#44566,#44567)) ;
#20493=EDGE_LOOP('',(#44568,#44569,#44570,#44571)) ;
#20494=EDGE_LOOP('',(#44572,#44573,#44574,#44575)) ;
#20495=EDGE_LOOP('',(#44576,#44577,#44578,#44579)) ;
#20496=EDGE_LOOP('',(#44580,#44581,#44582,#44583)) ;
#20497=EDGE_LOOP('',(#44584,#44585,#44586,#44587)) ;
#20498=EDGE_LOOP('',(#44588,#44589,#44590,#44591)) ;
#20499=EDGE_LOOP('',(#44592,#44593,#44594,#44595)) ;
#20500=EDGE_LOOP('',(#44596,#44597,#44598,#44599)) ;
#20501=EDGE_LOOP('',(#44600,#44601,#44602,#44603)) ;
#20502=EDGE_LOOP('',(#44604,#44605,#44606,#44607)) ;
#20503=EDGE_LOOP('',(#44608,#44609,#44610,#44611)) ;
#20504=EDGE_LOOP('',(#44612,#44613,#44614,#44615)) ;
#20505=EDGE_LOOP('',(#44616,#44617,#44618,#44619)) ;
#20506=EDGE_LOOP('',(#44620,#44621,#44622,#44623)) ;
#20507=EDGE_LOOP('',(#44624,#44625,#44626,#44627)) ;
#20508=EDGE_LOOP('',(#44628,#44629,#44630,#44631)) ;
#20509=EDGE_LOOP('',(#44632,#44633,#44634,#44635)) ;
#20510=EDGE_LOOP('',(#44636,#44637,#44638,#44639)) ;
#20511=EDGE_LOOP('',(#44640,#44641,#44642,#44643)) ;
#20512=EDGE_LOOP('',(#44644,#44645,#44646,#44647)) ;
#20513=EDGE_LOOP('',(#44648,#44649,#44650,#44651)) ;
#20514=EDGE_LOOP('',(#44652,#44653,#44654,#44655)) ;
#20515=EDGE_LOOP('',(#44656,#44657,#44658,#44659)) ;
#20516=EDGE_LOOP('',(#44660,#44661,#44662,#44663)) ;
#20517=EDGE_LOOP('',(#44664,#44665,#44666,#44667)) ;
#20518=EDGE_LOOP('',(#44668,#44669,#44670,#44671)) ;
#20519=EDGE_LOOP('',(#44672,#44673,#44674,#44675)) ;
#20520=EDGE_LOOP('',(#44676,#44677,#44678,#44679)) ;
#20521=EDGE_LOOP('',(#44680,#44681,#44682,#44683)) ;
#20522=EDGE_LOOP('',(#44684,#44685,#44686,#44687)) ;
#20523=EDGE_LOOP('',(#44688,#44689,#44690,#44691)) ;
#20524=EDGE_LOOP('',(#44692,#44693,#44694,#44695)) ;
#20525=EDGE_LOOP('',(#44696,#44697,#44698,#44699)) ;
#20526=EDGE_LOOP('',(#44700,#44701,#44702,#44703)) ;
#20527=EDGE_LOOP('',(#44704,#44705,#44706,#44707)) ;
#20528=EDGE_LOOP('',(#44708,#44709,#44710,#44711)) ;
#20529=EDGE_LOOP('',(#44712,#44713,#44714,#44715)) ;
#20530=EDGE_LOOP('',(#44716,#44717,#44718,#44719)) ;
#20531=EDGE_LOOP('',(#44720,#44721,#44722,#44723)) ;
#20532=EDGE_LOOP('',(#44724,#44725,#44726,#44727)) ;
#20533=EDGE_LOOP('',(#44728,#44729,#44730,#44731)) ;
#20534=EDGE_LOOP('',(#44732,#44733,#44734,#44735)) ;
#20535=EDGE_LOOP('',(#44736,#44737,#44738,#44739)) ;
#20536=EDGE_LOOP('',(#44740,#44741,#44742,#44743)) ;
#20537=EDGE_LOOP('',(#44744,#44745,#44746,#44747)) ;
#20538=EDGE_LOOP('',(#44748,#44749,#44750)) ;
#20539=EDGE_LOOP('',(#44751,#44752,#44753,#44754)) ;
#20540=EDGE_LOOP('',(#44755,#44756,#44757,#44758)) ;
#20541=EDGE_LOOP('',(#44759,#44760,#44761,#44762)) ;
#20542=EDGE_LOOP('',(#44763,#44764,#44765)) ;
#20543=EDGE_LOOP('',(#44766,#44767,#44768)) ;
#20544=EDGE_LOOP('',(#44769,#44770,#44771,#44772)) ;
#20545=EDGE_LOOP('',(#44773,#44774,#44775,#44776)) ;
#20546=EDGE_LOOP('',(#44777,#44778,#44779,#44780)) ;
#20547=EDGE_LOOP('',(#44781,#44782,#44783)) ;
#20548=EDGE_LOOP('',(#44784,#44785,#44786,#44787)) ;
#20549=EDGE_LOOP('',(#44788,#44789,#44790,#44791)) ;
#20550=EDGE_LOOP('',(#44792,#44793,#44794,#44795)) ;
#20551=EDGE_LOOP('',(#44796,#44797,#44798,#44799)) ;
#20552=EDGE_LOOP('',(#44800,#44801,#44802,#44803)) ;
#20553=EDGE_LOOP('',(#44804,#44805,#44806)) ;
#20554=EDGE_LOOP('',(#44807,#44808,#44809,#44810)) ;
#20555=EDGE_LOOP('',(#44811,#44812,#44813,#44814)) ;
#20556=EDGE_LOOP('',(#44815,#44816,#44817,#44818)) ;
#20557=EDGE_LOOP('',(#44819,#44820,#44821)) ;
#20558=EDGE_LOOP('',(#44822,#44823,#44824)) ;
#20559=EDGE_LOOP('',(#44825,#44826,#44827,#44828)) ;
#20560=EDGE_LOOP('',(#44829,#44830,#44831,#44832)) ;
#20561=EDGE_LOOP('',(#44833,#44834,#44835,#44836)) ;
#20562=EDGE_LOOP('',(#44837,#44838,#44839,#44840)) ;
#20563=EDGE_LOOP('',(#44841,#44842,#44843)) ;
#20564=EDGE_LOOP('',(#44844,#44845,#44846,#44847)) ;
#20565=EDGE_LOOP('',(#44848,#44849,#44850)) ;
#20566=EDGE_LOOP('',(#44851,#44852,#44853,#44854)) ;
#20567=EDGE_LOOP('',(#44855,#44856,#44857,#44858)) ;
#20568=EDGE_LOOP('',(#44859,#44860,#44861,#44862)) ;
#20569=EDGE_LOOP('',(#44863,#44864,#44865,#44866)) ;
#20570=EDGE_LOOP('',(#44867,#44868,#44869,#44870)) ;
#20571=EDGE_LOOP('',(#44871,#44872,#44873,#44874)) ;
#20572=EDGE_LOOP('',(#44875,#44876,#44877,#44878)) ;
#20573=EDGE_LOOP('',(#44879,#44880,#44881,#44882)) ;
#20574=EDGE_LOOP('',(#44883,#44884,#44885,#44886)) ;
#20575=EDGE_LOOP('',(#44887,#44888,#44889)) ;
#20576=EDGE_LOOP('',(#44890,#44891,#44892)) ;
#20577=EDGE_LOOP('',(#44893,#44894,#44895,#44896)) ;
#20578=EDGE_LOOP('',(#44897,#44898,#44899,#44900)) ;
#20579=EDGE_LOOP('',(#44901,#44902,#44903,#44904)) ;
#20580=EDGE_LOOP('',(#44905,#44906,#44907,#44908)) ;
#20581=EDGE_LOOP('',(#44909,#44910,#44911,#44912)) ;
#20582=EDGE_LOOP('',(#44913,#44914,#44915,#44916)) ;
#20583=EDGE_LOOP('',(#44917,#44918,#44919,#44920)) ;
#20584=EDGE_LOOP('',(#44921,#44922,#44923,#44924)) ;
#20585=EDGE_LOOP('',(#44925,#44926,#44927)) ;
#20586=EDGE_LOOP('',(#44928,#44929,#44930,#44931)) ;
#20587=EDGE_LOOP('',(#44932,#44933,#44934,#44935)) ;
#20588=EDGE_LOOP('',(#44936,#44937,#44938,#44939)) ;
#20589=EDGE_LOOP('',(#44940,#44941,#44942,#44943)) ;
#20590=EDGE_LOOP('',(#44944,#44945,#44946,#44947)) ;
#20591=EDGE_LOOP('',(#44948,#44949,#44950,#44951)) ;
#20592=EDGE_LOOP('',(#44952,#44953,#44954,#44955)) ;
#20593=EDGE_LOOP('',(#44956,#44957,#44958)) ;
#20594=EDGE_LOOP('',(#44959,#44960,#44961)) ;
#20595=EDGE_LOOP('',(#44962,#44963,#44964,#44965)) ;
#20596=EDGE_LOOP('',(#44966,#44967,#44968,#44969)) ;
#20597=EDGE_LOOP('',(#44970,#44971,#44972,#44973)) ;
#20598=EDGE_LOOP('',(#44974,#44975,#44976,#44977)) ;
#20599=EDGE_LOOP('',(#44978,#44979,#44980,#44981)) ;
#20600=EDGE_LOOP('',(#44982,#44983,#44984,#44985)) ;
#20601=EDGE_LOOP('',(#44986,#44987,#44988,#44989)) ;
#20602=EDGE_LOOP('',(#44990,#44991,#44992)) ;
#20603=EDGE_LOOP('',(#44993,#44994,#44995)) ;
#20604=EDGE_LOOP('',(#44996,#44997,#44998,#44999)) ;
#20605=EDGE_LOOP('',(#45000,#45001,#45002)) ;
#20606=EDGE_LOOP('',(#45003,#45004,#45005)) ;
#20607=EDGE_LOOP('',(#45006,#45007,#45008,#45009)) ;
#20608=EDGE_LOOP('',(#45010,#45011,#45012,#45013)) ;
#20609=EDGE_LOOP('',(#45014,#45015,#45016,#45017)) ;
#20610=EDGE_LOOP('',(#45018,#45019,#45020,#45021)) ;
#20611=EDGE_LOOP('',(#45022,#45023,#45024,#45025)) ;
#20612=EDGE_LOOP('',(#45026,#45027,#45028,#45029)) ;
#20613=EDGE_LOOP('',(#45030,#45031,#45032,#45033)) ;
#20614=EDGE_LOOP('',(#45034,#45035,#45036,#45037)) ;
#20615=EDGE_LOOP('',(#45038,#45039,#45040)) ;
#20616=EDGE_LOOP('',(#45041,#45042,#45043,#45044)) ;
#20617=EDGE_LOOP('',(#45045,#45046,#45047,#45048)) ;
#20618=EDGE_LOOP('',(#45049,#45050,#45051)) ;
#20619=EDGE_LOOP('',(#45052,#45053,#45054,#45055)) ;
#20620=EDGE_LOOP('',(#45056,#45057,#45058,#45059)) ;
#20621=EDGE_LOOP('',(#45060,#45061,#45062,#45063)) ;
#20622=EDGE_LOOP('',(#45064,#45065,#45066,#45067)) ;
#20623=EDGE_LOOP('',(#45068,#45069,#45070,#45071)) ;
#20624=EDGE_LOOP('',(#45072,#45073,#45074,#45075)) ;
#20625=EDGE_LOOP('',(#45076,#45077,#45078,#45079)) ;
#20626=EDGE_LOOP('',(#45080,#45081,#45082,#45083)) ;
#20627=EDGE_LOOP('',(#45084,#45085,#45086,#45087)) ;
#20628=EDGE_LOOP('',(#45088,#45089,#45090,#45091)) ;
#20629=EDGE_LOOP('',(#45092,#45093,#45094,#45095)) ;
#20630=EDGE_LOOP('',(#45096,#45097,#45098,#45099)) ;
#20631=EDGE_LOOP('',(#45100,#45101,#45102,#45103)) ;
#20632=EDGE_LOOP('',(#45104,#45105,#45106,#45107)) ;
#20633=EDGE_LOOP('',(#45108,#45109,#45110,#45111)) ;
#20634=EDGE_LOOP('',(#45112,#45113,#45114,#45115)) ;
#20635=EDGE_LOOP('',(#45116,#45117,#45118,#45119)) ;
#20636=EDGE_LOOP('',(#45120,#45121,#45122,#45123)) ;
#20637=EDGE_LOOP('',(#45124,#45125,#45126,#45127)) ;
#20638=EDGE_LOOP('',(#45128,#45129,#45130,#45131)) ;
#20639=EDGE_LOOP('',(#45132,#45133,#45134,#45135)) ;
#20640=EDGE_LOOP('',(#45136,#45137,#45138,#45139)) ;
#20641=EDGE_LOOP('',(#45140,#45141,#45142,#45143)) ;
#20642=EDGE_LOOP('',(#45144,#45145,#45146,#45147)) ;
#20643=EDGE_LOOP('',(#45148,#45149,#45150,#45151)) ;
#20644=EDGE_LOOP('',(#45152,#45153,#45154,#45155)) ;
#20645=EDGE_LOOP('',(#45156,#45157,#45158,#45159)) ;
#20646=EDGE_LOOP('',(#45160,#45161,#45162,#45163)) ;
#20647=EDGE_LOOP('',(#45164,#45165,#45166,#45167)) ;
#20648=EDGE_LOOP('',(#45168,#45169,#45170,#45171)) ;
#20649=EDGE_LOOP('',(#45172,#45173,#45174,#45175)) ;
#20650=EDGE_LOOP('',(#45176,#45177,#45178,#45179)) ;
#20651=EDGE_LOOP('',(#45180,#45181,#45182,#45183)) ;
#20652=EDGE_LOOP('',(#45184,#45185,#45186,#45187)) ;
#20653=EDGE_LOOP('',(#45188,#45189,#45190,#45191)) ;
#20654=EDGE_LOOP('',(#45192,#45193,#45194,#45195)) ;
#20655=EDGE_LOOP('',(#45196,#45197,#45198,#45199)) ;
#20656=EDGE_LOOP('',(#45200,#45201,#45202,#45203)) ;
#20657=EDGE_LOOP('',(#45204,#45205,#45206,#45207)) ;
#20658=EDGE_LOOP('',(#45208,#45209,#45210,#45211)) ;
#20659=EDGE_LOOP('',(#45212,#45213,#45214,#45215)) ;
#20660=EDGE_LOOP('',(#45216,#45217,#45218,#45219)) ;
#20661=EDGE_LOOP('',(#45220,#45221,#45222,#45223)) ;
#20662=EDGE_LOOP('',(#45224,#45225,#45226,#45227)) ;
#20663=EDGE_LOOP('',(#45228,#45229,#45230,#45231)) ;
#20664=EDGE_LOOP('',(#45232,#45233,#45234,#45235)) ;
#20665=EDGE_LOOP('',(#45236,#45237,#45238,#45239)) ;
#20666=EDGE_LOOP('',(#45240,#45241,#45242,#45243)) ;
#20667=EDGE_LOOP('',(#45244,#45245,#45246,#45247)) ;
#20668=EDGE_LOOP('',(#45248,#45249,#45250,#45251)) ;
#20669=EDGE_LOOP('',(#45252,#45253,#45254,#45255)) ;
#20670=EDGE_LOOP('',(#45256,#45257,#45258,#45259)) ;
#20671=EDGE_LOOP('',(#45260,#45261,#45262,#45263)) ;
#20672=EDGE_LOOP('',(#45264,#45265,#45266,#45267)) ;
#20673=EDGE_LOOP('',(#45268,#45269,#45270,#45271)) ;
#20674=EDGE_LOOP('',(#45272,#45273,#45274,#45275)) ;
#20675=EDGE_LOOP('',(#45276,#45277,#45278,#45279)) ;
#20676=EDGE_LOOP('',(#45280,#45281,#45282,#45283)) ;
#20677=EDGE_LOOP('',(#45284,#45285,#45286,#45287)) ;
#20678=EDGE_LOOP('',(#45288,#45289,#45290,#45291)) ;
#20679=EDGE_LOOP('',(#45292,#45293,#45294,#45295)) ;
#20680=EDGE_LOOP('',(#45296,#45297,#45298,#45299)) ;
#20681=EDGE_LOOP('',(#45300,#45301,#45302,#45303)) ;
#20682=EDGE_LOOP('',(#45304,#45305,#45306,#45307)) ;
#20683=EDGE_LOOP('',(#45308,#45309,#45310,#45311)) ;
#20684=EDGE_LOOP('',(#45312,#45313,#45314,#45315)) ;
#20685=EDGE_LOOP('',(#45316,#45317,#45318,#45319)) ;
#20686=EDGE_LOOP('',(#45320,#45321,#45322,#45323)) ;
#20687=EDGE_LOOP('',(#45324,#45325,#45326,#45327)) ;
#20688=EDGE_LOOP('',(#45328,#45329,#45330,#45331)) ;
#20689=EDGE_LOOP('',(#45332,#45333,#45334,#45335)) ;
#20690=EDGE_LOOP('',(#45336,#45337,#45338,#45339)) ;
#20691=EDGE_LOOP('',(#45340,#45341,#45342,#45343)) ;
#20692=EDGE_LOOP('',(#45344,#45345,#45346,#45347)) ;
#20693=EDGE_LOOP('',(#45348,#45349,#45350,#45351)) ;
#20694=EDGE_LOOP('',(#45352,#45353,#45354,#45355)) ;
#20695=EDGE_LOOP('',(#45356,#45357,#45358,#45359)) ;
#20696=EDGE_LOOP('',(#45360,#45361,#45362,#45363)) ;
#20697=EDGE_LOOP('',(#45364,#45365,#45366,#45367)) ;
#20698=EDGE_LOOP('',(#45368,#45369,#45370,#45371)) ;
#20699=EDGE_LOOP('',(#45372,#45373,#45374,#45375)) ;
#20700=EDGE_LOOP('',(#45376,#45377,#45378,#45379)) ;
#20701=EDGE_LOOP('',(#45380,#45381,#45382,#45383)) ;
#20702=EDGE_LOOP('',(#45384,#45385,#45386,#45387)) ;
#20703=EDGE_LOOP('',(#45388,#45389,#45390,#45391)) ;
#20704=EDGE_LOOP('',(#45392,#45393,#45394,#45395)) ;
#20705=EDGE_LOOP('',(#45396,#45397,#45398,#45399)) ;
#20706=EDGE_LOOP('',(#45400,#45401,#45402,#45403)) ;
#20707=EDGE_LOOP('',(#45404,#45405,#45406,#45407)) ;
#20708=EDGE_LOOP('',(#45408,#45409,#45410,#45411)) ;
#20709=EDGE_LOOP('',(#45412,#45413,#45414,#45415)) ;
#20710=EDGE_LOOP('',(#45416,#45417,#45418,#45419)) ;
#20711=EDGE_LOOP('',(#45420,#45421,#45422,#45423)) ;
#20712=EDGE_LOOP('',(#45424,#45425,#45426,#45427)) ;
#20713=EDGE_LOOP('',(#45428,#45429,#45430,#45431)) ;
#20714=EDGE_LOOP('',(#45432,#45433,#45434,#45435)) ;
#20715=EDGE_LOOP('',(#45436,#45437,#45438,#45439)) ;
#20716=EDGE_LOOP('',(#45440,#45441,#45442,#45443)) ;
#20717=EDGE_LOOP('',(#45444,#45445,#45446,#45447)) ;
#20718=EDGE_LOOP('',(#45448,#45449,#45450,#45451)) ;
#20719=EDGE_LOOP('',(#45452,#45453,#45454,#45455)) ;
#20720=EDGE_LOOP('',(#45456,#45457,#45458,#45459)) ;
#20721=EDGE_LOOP('',(#45460,#45461,#45462,#45463)) ;
#20722=EDGE_LOOP('',(#45464,#45465,#45466,#45467)) ;
#20723=EDGE_LOOP('',(#45468,#45469,#45470,#45471)) ;
#20724=EDGE_LOOP('',(#45472,#45473,#45474,#45475)) ;
#20725=EDGE_LOOP('',(#45476,#45477,#45478,#45479)) ;
#20726=EDGE_LOOP('',(#45480,#45481,#45482,#45483)) ;
#20727=EDGE_LOOP('',(#45484,#45485,#45486,#45487)) ;
#20728=EDGE_LOOP('',(#45488,#45489,#45490,#45491)) ;
#20729=EDGE_LOOP('',(#45492,#45493,#45494,#45495)) ;
#20730=EDGE_LOOP('',(#45496,#45497,#45498,#45499)) ;
#20731=EDGE_LOOP('',(#45500,#45501,#45502,#45503)) ;
#20732=EDGE_LOOP('',(#45504,#45505,#45506,#45507)) ;
#20733=EDGE_LOOP('',(#45508,#45509,#45510,#45511)) ;
#20734=EDGE_LOOP('',(#45512,#45513,#45514,#45515)) ;
#20735=EDGE_LOOP('',(#45516,#45517,#45518,#45519)) ;
#20736=EDGE_LOOP('',(#45520,#45521,#45522,#45523)) ;
#20737=EDGE_LOOP('',(#45524,#45525,#45526,#45527)) ;
#20738=EDGE_LOOP('',(#45528,#45529,#45530,#45531)) ;
#20739=EDGE_LOOP('',(#45532,#45533,#45534,#45535)) ;
#20740=EDGE_LOOP('',(#45536,#45537,#45538,#45539)) ;
#20741=EDGE_LOOP('',(#45540,#45541,#45542,#45543)) ;
#20742=EDGE_LOOP('',(#45544,#45545,#45546,#45547)) ;
#20743=EDGE_LOOP('',(#45548,#45549,#45550,#45551)) ;
#20744=EDGE_LOOP('',(#45552,#45553,#45554,#45555)) ;
#20745=EDGE_LOOP('',(#45556,#45557,#45558,#45559)) ;
#20746=EDGE_LOOP('',(#45560,#45561,#45562,#45563)) ;
#20747=EDGE_LOOP('',(#45564,#45565,#45566,#45567)) ;
#20748=EDGE_LOOP('',(#45568,#45569,#45570,#45571)) ;
#20749=EDGE_LOOP('',(#45572,#45573,#45574,#45575)) ;
#20750=EDGE_LOOP('',(#45576,#45577,#45578,#45579)) ;
#20751=EDGE_LOOP('',(#45580,#45581,#45582,#45583)) ;
#20752=EDGE_LOOP('',(#45584,#45585,#45586,#45587)) ;
#20753=EDGE_LOOP('',(#45588,#45589,#45590,#45591)) ;
#20754=EDGE_LOOP('',(#45592,#45593,#45594,#45595)) ;
#20755=EDGE_LOOP('',(#45596,#45597,#45598,#45599)) ;
#20756=EDGE_LOOP('',(#45600,#45601,#45602,#45603)) ;
#20757=EDGE_LOOP('',(#45604,#45605,#45606,#45607)) ;
#20758=EDGE_LOOP('',(#45608,#45609,#45610,#45611)) ;
#20759=EDGE_LOOP('',(#45612,#45613,#45614,#45615)) ;
#20760=EDGE_LOOP('',(#45616,#45617,#45618,#45619)) ;
#20761=EDGE_LOOP('',(#45620,#45621,#45622,#45623)) ;
#20762=EDGE_LOOP('',(#45624,#45625,#45626,#45627)) ;
#20763=EDGE_LOOP('',(#45628,#45629,#45630,#45631)) ;
#20764=EDGE_LOOP('',(#45632,#45633,#45634,#45635)) ;
#20765=EDGE_LOOP('',(#45636,#45637,#45638,#45639)) ;
#20766=EDGE_LOOP('',(#45640,#45641,#45642,#45643)) ;
#20767=EDGE_LOOP('',(#45644,#45645,#45646,#45647)) ;
#20768=EDGE_LOOP('',(#45648,#45649,#45650,#45651)) ;
#20769=EDGE_LOOP('',(#45652,#45653,#45654,#45655)) ;
#20770=EDGE_LOOP('',(#45656,#45657,#45658,#45659)) ;
#20771=EDGE_LOOP('',(#45660,#45661,#45662,#45663)) ;
#20772=EDGE_LOOP('',(#45664,#45665,#45666,#45667)) ;
#20773=EDGE_LOOP('',(#45668,#45669,#45670,#45671)) ;
#20774=EDGE_LOOP('',(#45672,#45673,#45674,#45675)) ;
#20775=EDGE_LOOP('',(#45676,#45677,#45678,#45679)) ;
#20776=EDGE_LOOP('',(#45680,#45681,#45682,#45683)) ;
#20777=EDGE_LOOP('',(#45684,#45685,#45686,#45687)) ;
#20778=EDGE_LOOP('',(#45688,#45689,#45690,#45691)) ;
#20779=EDGE_LOOP('',(#45692,#45693,#45694,#45695)) ;
#20780=EDGE_LOOP('',(#45696,#45697,#45698,#45699)) ;
#20781=EDGE_LOOP('',(#45700,#45701,#45702,#45703)) ;
#20782=EDGE_LOOP('',(#45704,#45705,#45706,#45707)) ;
#20783=EDGE_LOOP('',(#45708,#45709,#45710,#45711)) ;
#20784=EDGE_LOOP('',(#45712,#45713,#45714,#45715)) ;
#20785=EDGE_LOOP('',(#45716,#45717,#45718,#45719)) ;
#20786=EDGE_LOOP('',(#45720,#45721,#45722,#45723)) ;
#20787=EDGE_LOOP('',(#45724,#45725,#45726,#45727)) ;
#20788=EDGE_LOOP('',(#45728,#45729,#45730,#45731)) ;
#20789=EDGE_LOOP('',(#45732,#45733,#45734,#45735)) ;
#20790=EDGE_LOOP('',(#45736,#45737,#45738,#45739)) ;
#20791=EDGE_LOOP('',(#45740,#45741,#45742,#45743)) ;
#20792=EDGE_LOOP('',(#45744,#45745,#45746,#45747)) ;
#20793=EDGE_LOOP('',(#45748,#45749,#45750,#45751)) ;
#20794=EDGE_LOOP('',(#45752,#45753,#45754,#45755)) ;
#20795=EDGE_LOOP('',(#45756,#45757,#45758,#45759)) ;
#20796=EDGE_LOOP('',(#45760,#45761,#45762,#45763)) ;
#20797=EDGE_LOOP('',(#45764,#45765,#45766,#45767)) ;
#20798=EDGE_LOOP('',(#45768,#45769,#45770,#45771)) ;
#20799=EDGE_LOOP('',(#45772,#45773,#45774,#45775)) ;
#20800=EDGE_LOOP('',(#45776,#45777,#45778,#45779)) ;
#20801=EDGE_LOOP('',(#45780,#45781,#45782,#45783)) ;
#20802=EDGE_LOOP('',(#45784,#45785,#45786,#45787)) ;
#20803=EDGE_LOOP('',(#45788,#45789,#45790,#45791)) ;
#20804=EDGE_LOOP('',(#45792,#45793,#45794,#45795)) ;
#20805=EDGE_LOOP('',(#45796,#45797,#45798,#45799)) ;
#20806=EDGE_LOOP('',(#45800,#45801,#45802,#45803)) ;
#20807=EDGE_LOOP('',(#45804,#45805,#45806,#45807)) ;
#20808=EDGE_LOOP('',(#45808,#45809,#45810,#45811)) ;
#20809=EDGE_LOOP('',(#45812,#45813,#45814,#45815)) ;
#20810=EDGE_LOOP('',(#45816,#45817,#45818,#45819)) ;
#20811=EDGE_LOOP('',(#45820,#45821,#45822,#45823)) ;
#20812=EDGE_LOOP('',(#45824,#45825,#45826,#45827)) ;
#20813=EDGE_LOOP('',(#45828,#45829,#45830,#45831)) ;
#20814=EDGE_LOOP('',(#45832,#45833,#45834,#45835)) ;
#20815=EDGE_LOOP('',(#45836,#45837,#45838,#45839)) ;
#20816=EDGE_LOOP('',(#45840,#45841,#45842,#45843)) ;
#20817=EDGE_LOOP('',(#45844,#45845,#45846,#45847)) ;
#20818=EDGE_LOOP('',(#45848,#45849,#45850,#45851)) ;
#20819=EDGE_LOOP('',(#45852,#45853,#45854,#45855)) ;
#20820=EDGE_LOOP('',(#45856,#45857,#45858,#45859)) ;
#20821=EDGE_LOOP('',(#45860,#45861,#45862,#45863)) ;
#20822=EDGE_LOOP('',(#45864,#45865,#45866,#45867)) ;
#20823=EDGE_LOOP('',(#45868,#45869,#45870,#45871)) ;
#20824=EDGE_LOOP('',(#45872,#45873,#45874,#45875)) ;
#20825=EDGE_LOOP('',(#45876,#45877,#45878,#45879)) ;
#20826=EDGE_LOOP('',(#45880,#45881,#45882,#45883)) ;
#20827=EDGE_LOOP('',(#45884,#45885,#45886,#45887)) ;
#20828=EDGE_LOOP('',(#45888,#45889,#45890,#45891)) ;
#20829=EDGE_LOOP('',(#45892,#45893,#45894,#45895)) ;
#20830=EDGE_LOOP('',(#45896,#45897,#45898,#45899)) ;
#20831=EDGE_LOOP('',(#45900,#45901,#45902,#45903)) ;
#20832=EDGE_LOOP('',(#45904,#45905,#45906,#45907)) ;
#20833=EDGE_LOOP('',(#45908,#45909,#45910,#45911)) ;
#20834=EDGE_LOOP('',(#45912,#45913,#45914,#45915)) ;
#20835=EDGE_LOOP('',(#45916,#45917,#45918,#45919)) ;
#20836=EDGE_LOOP('',(#45920,#45921,#45922,#45923)) ;
#20837=EDGE_LOOP('',(#45924,#45925,#45926,#45927)) ;
#20838=EDGE_LOOP('',(#45928,#45929,#45930,#45931)) ;
#20839=EDGE_LOOP('',(#45932,#45933,#45934,#45935)) ;
#20840=EDGE_LOOP('',(#45936,#45937,#45938,#45939)) ;
#20841=EDGE_LOOP('',(#45940,#45941,#45942,#45943)) ;
#20842=EDGE_LOOP('',(#45944,#45945,#45946,#45947)) ;
#20843=EDGE_LOOP('',(#45948,#45949,#45950,#45951)) ;
#20844=EDGE_LOOP('',(#45952,#45953,#45954,#45955)) ;
#20845=EDGE_LOOP('',(#45956,#45957,#45958,#45959)) ;
#20846=EDGE_LOOP('',(#45960,#45961,#45962,#45963)) ;
#20847=EDGE_LOOP('',(#45964,#45965,#45966,#45967)) ;
#20848=EDGE_LOOP('',(#45968,#45969,#45970,#45971)) ;
#20849=EDGE_LOOP('',(#45972,#45973,#45974,#45975)) ;
#20850=EDGE_LOOP('',(#45976,#45977,#45978,#45979)) ;
#20851=EDGE_LOOP('',(#45980,#45981,#45982,#45983)) ;
#20852=EDGE_LOOP('',(#45984,#45985,#45986,#45987)) ;
#20853=EDGE_LOOP('',(#45988,#45989,#45990,#45991)) ;
#20854=EDGE_LOOP('',(#45992,#45993,#45994,#45995)) ;
#20855=EDGE_LOOP('',(#45996,#45997,#45998,#45999)) ;
#20856=EDGE_LOOP('',(#46000,#46001,#46002,#46003)) ;
#20857=EDGE_LOOP('',(#46004,#46005,#46006,#46007)) ;
#20858=EDGE_LOOP('',(#46008,#46009,#46010,#46011)) ;
#20859=EDGE_LOOP('',(#46012,#46013,#46014,#46015)) ;
#20860=EDGE_LOOP('',(#46016,#46017,#46018,#46019)) ;
#20861=EDGE_LOOP('',(#46020,#46021,#46022,#46023)) ;
#20862=EDGE_LOOP('',(#46024,#46025,#46026,#46027)) ;
#20863=EDGE_LOOP('',(#46028,#46029,#46030,#46031)) ;
#20864=EDGE_LOOP('',(#46032,#46033,#46034,#46035)) ;
#20865=EDGE_LOOP('',(#46036,#46037,#46038,#46039)) ;
#20866=EDGE_LOOP('',(#46040,#46041,#46042,#46043)) ;
#20867=EDGE_LOOP('',(#46044,#46045,#46046,#46047)) ;
#20868=EDGE_LOOP('',(#46048,#46049,#46050,#46051)) ;
#20869=EDGE_LOOP('',(#46052,#46053,#46054,#46055)) ;
#20870=EDGE_LOOP('',(#46056,#46057,#46058,#46059)) ;
#20871=EDGE_LOOP('',(#46060,#46061,#46062)) ;
#20872=EDGE_LOOP('',(#46063,#46064,#46065,#46066)) ;
#20873=EDGE_LOOP('',(#46067,#46068,#46069,#46070)) ;
#20874=EDGE_LOOP('',(#46071,#46072,#46073)) ;
#20875=EDGE_LOOP('',(#46074,#46075,#46076,#46077)) ;
#20876=EDGE_LOOP('',(#46078,#46079,#46080,#46081)) ;
#20877=EDGE_LOOP('',(#46082,#46083,#46084,#46085)) ;
#20878=EDGE_LOOP('',(#46086,#46087,#46088,#46089)) ;
#20879=EDGE_LOOP('',(#46090,#46091,#46092)) ;
#20880=EDGE_LOOP('',(#46093,#46094,#46095)) ;
#20881=EDGE_LOOP('',(#46096,#46097,#46098,#46099)) ;
#24719=CIRCLE('',#67766,1.6) ;
#24720=CIRCLE('',#67767,1.6) ;
#24721=CIRCLE('',#67768,0.15) ;
#24722=CIRCLE('',#67769,1.75) ;
#24723=CIRCLE('',#67771,1.75) ;
#24724=CIRCLE('',#67772,0.15) ;
#24725=CIRCLE('',#67773,1.6) ;
#24726=CIRCLE('',#67774,1.6) ;
#24727=CIRCLE('',#67776,1.54393398282201) ;
#24728=CIRCLE('',#67777,1.54393398282201) ;
#24729=CIRCLE('',#67778,0.15) ;
#24730=CIRCLE('',#67779,1.49999999999999) ;
#24731=CIRCLE('',#67780,1.49999999999999) ;
#24732=CIRCLE('',#67782,1.64999999999999) ;
#24733=CIRCLE('',#67783,0.15) ;
#24734=CIRCLE('',#67784,1.49999999999999) ;
#24735=CIRCLE('',#67786,1.54393398282201) ;
#24736=CIRCLE('',#67787,1.54393398282201) ;
#24737=CIRCLE('',#67788,0.15) ;
#24738=CIRCLE('',#67789,1.49999999999999) ;
#24739=CIRCLE('',#67790,1.49999999999999) ;
#24740=CIRCLE('',#67792,1.64999999999999) ;
#24741=CIRCLE('',#67793,0.15) ;
#24742=CIRCLE('',#67794,1.49999999999999) ;
#24743=CIRCLE('',#67796,1.6) ;
#24744=CIRCLE('',#67799,1.6) ;
#24745=CIRCLE('',#67803,0.3) ;
#24746=CIRCLE('',#67804,0.3) ;
#24747=CIRCLE('',#67805,0.3) ;
#24748=CIRCLE('',#67806,0.3) ;
#24749=CIRCLE('',#67808,0.3) ;
#24750=CIRCLE('',#67809,0.3) ;
#24751=CIRCLE('',#67810,0.3) ;
#24752=CIRCLE('',#67811,0.3) ;
#24753=CIRCLE('',#67813,0.3) ;
#24754=CIRCLE('',#67814,0.3) ;
#24755=CIRCLE('',#67815,0.3) ;
#24756=CIRCLE('',#67816,0.3) ;
#24757=CIRCLE('',#67817,0.3) ;
#24758=CIRCLE('',#67818,0.3) ;
#24759=CIRCLE('',#67819,0.3) ;
#24760=CIRCLE('',#67820,0.3) ;
#24761=CIRCLE('',#67821,0.3) ;
#24762=CIRCLE('',#67822,0.3) ;
#24763=CIRCLE('',#67823,0.3) ;
#24764=CIRCLE('',#67824,0.3) ;
#24765=CIRCLE('',#67825,0.3) ;
#24766=CIRCLE('',#67826,0.3) ;
#24767=CIRCLE('',#67827,0.3) ;
#24768=CIRCLE('',#67828,0.3) ;
#24769=CIRCLE('',#67829,0.3) ;
#24770=CIRCLE('',#67830,0.3) ;
#24771=CIRCLE('',#67832,0.3) ;
#24772=CIRCLE('',#67833,0.3) ;
#24773=CIRCLE('',#67834,0.3) ;
#24774=CIRCLE('',#67835,0.3) ;
#24775=CIRCLE('',#67836,0.3) ;
#24776=CIRCLE('',#67837,0.3) ;
#24777=CIRCLE('',#67838,0.3) ;
#24778=CIRCLE('',#67839,0.3) ;
#24779=CIRCLE('',#67840,0.3) ;
#24780=CIRCLE('',#67841,0.3) ;
#24781=CIRCLE('',#67842,0.3) ;
#24782=CIRCLE('',#67843,0.3) ;
#24783=CIRCLE('',#67844,0.3) ;
#24784=CIRCLE('',#67845,0.3) ;
#24785=CIRCLE('',#67846,0.3) ;
#24786=CIRCLE('',#67847,0.3) ;
#24787=CIRCLE('',#67848,0.3) ;
#24788=CIRCLE('',#67849,0.3) ;
#24789=CIRCLE('',#67851,0.3) ;
#24790=CIRCLE('',#67852,0.3) ;
#24791=CIRCLE('',#67853,0.3) ;
#24792=CIRCLE('',#67854,0.3) ;
#24793=CIRCLE('',#67855,0.300000000000001) ;
#24794=CIRCLE('',#67856,0.3) ;
#24795=CIRCLE('',#67857,0.300000000000002) ;
#24796=CIRCLE('',#67858,0.300000000000002) ;
#24797=CIRCLE('',#67859,0.300000000000002) ;
#24798=CIRCLE('',#67860,0.300000000000002) ;
#24799=CIRCLE('',#67861,0.300000000000002) ;
#24800=CIRCLE('',#67862,0.300000000000002) ;
#24801=CIRCLE('',#67863,0.300000000000002) ;
#24802=CIRCLE('',#67864,0.300000000000002) ;
#24803=CIRCLE('',#67865,0.300000000000002) ;
#24804=CIRCLE('',#67866,0.300000000000002) ;
#24805=CIRCLE('',#67867,0.300000000000002) ;
#24806=CIRCLE('',#67868,0.300000000000002) ;
#24807=CIRCLE('',#67869,0.300000000000002) ;
#24808=CIRCLE('',#67870,0.300000000000002) ;
#24809=CIRCLE('',#67871,0.300000000000002) ;
#24810=CIRCLE('',#67872,0.300000000000002) ;
#24811=CIRCLE('',#67873,0.300000000000002) ;
#24812=CIRCLE('',#67874,0.300000000000002) ;
#24813=CIRCLE('',#67875,0.300000000000002) ;
#24814=CIRCLE('',#67876,0.300000000000002) ;
#24815=CIRCLE('',#67877,0.3) ;
#24816=CIRCLE('',#67878,0.3) ;
#24817=CIRCLE('',#67879,0.300000000000002) ;
#24818=CIRCLE('',#67880,0.300000000000002) ;
#24819=CIRCLE('',#67882,0.3) ;
#24820=CIRCLE('',#67883,0.3) ;
#24821=CIRCLE('',#67884,0.3) ;
#24822=CIRCLE('',#67885,0.3) ;
#24823=CIRCLE('',#67886,0.3) ;
#24824=CIRCLE('',#67887,0.300000000000001) ;
#24825=CIRCLE('',#67888,0.300000000000002) ;
#24826=CIRCLE('',#67889,0.300000000000002) ;
#24827=CIRCLE('',#67890,0.300000000000002) ;
#24828=CIRCLE('',#67891,0.300000000000002) ;
#24829=CIRCLE('',#67892,0.300000000000002) ;
#24830=CIRCLE('',#67893,0.300000000000002) ;
#24831=CIRCLE('',#67894,0.300000000000002) ;
#24832=CIRCLE('',#67895,0.300000000000002) ;
#24833=CIRCLE('',#67896,0.300000000000002) ;
#24834=CIRCLE('',#67897,0.300000000000002) ;
#24835=CIRCLE('',#67898,0.300000000000002) ;
#24836=CIRCLE('',#67899,0.300000000000002) ;
#24837=CIRCLE('',#67900,0.300000000000002) ;
#24838=CIRCLE('',#67901,0.300000000000002) ;
#24839=CIRCLE('',#67902,0.300000000000002) ;
#24840=CIRCLE('',#67903,0.300000000000002) ;
#24841=CIRCLE('',#67904,0.300000000000002) ;
#24842=CIRCLE('',#67905,0.300000000000002) ;
#24843=CIRCLE('',#67906,0.300000000000002) ;
#24844=CIRCLE('',#67907,0.300000000000002) ;
#24845=CIRCLE('',#67908,0.3) ;
#24846=CIRCLE('',#67909,0.3) ;
#24847=CIRCLE('',#67910,0.300000000000002) ;
#24848=CIRCLE('',#67911,0.300000000000002) ;
#24849=CIRCLE('',#67913,0.3) ;
#24850=CIRCLE('',#67914,0.3) ;
#24851=CIRCLE('',#67916,0.3) ;
#24852=CIRCLE('',#67917,0.3) ;
#24853=CIRCLE('',#67924,1.15) ;
#24854=CIRCLE('',#67925,1.6) ;
#24855=CIRCLE('',#67927,1.) ;
#24856=CIRCLE('',#67928,1.75) ;
#24857=CIRCLE('',#67930,1.75) ;
#24858=CIRCLE('',#67932,1.) ;
#24859=CIRCLE('',#67947,1.) ;
#24860=CIRCLE('',#67948,1.75) ;
#24861=CIRCLE('',#67950,1.) ;
#24862=CIRCLE('',#67951,1.75) ;
#24863=CIRCLE('',#67955,1.15) ;
#24864=CIRCLE('',#67956,1.6) ;
#24865=CIRCLE('',#67958,1.) ;
#24866=CIRCLE('',#67959,1.75) ;
#24867=CIRCLE('',#67961,1.75) ;
#24868=CIRCLE('',#67963,1.) ;
#24869=CIRCLE('',#68021,0.149999999999997) ;
#24870=CIRCLE('',#68026,0.149999999999997) ;
#24871=CIRCLE('',#68027,0.149999999999997) ;
#24872=CIRCLE('',#68029,0.149999999999997) ;
#24873=CIRCLE('',#68031,0.149999999999997) ;
#24874=CIRCLE('',#68033,0.149999999999997) ;
#24875=CIRCLE('',#68035,0.149999999999997) ;
#24876=CIRCLE('',#68037,0.149999999999997) ;
#24877=CIRCLE('',#68038,0.15) ;
#24878=CIRCLE('',#68040,0.149999999999997) ;
#24879=CIRCLE('',#68042,0.15) ;
#24880=CIRCLE('',#68044,0.149999999999997) ;
#24881=CIRCLE('',#68046,0.149999999999997) ;
#24882=CIRCLE('',#68048,0.15) ;
#24883=CIRCLE('',#68049,0.149999999999997) ;
#24884=CIRCLE('',#68051,0.149999999999997) ;
#24885=CIRCLE('',#68053,0.15) ;
#24886=CIRCLE('',#68055,0.149999999999997) ;
#24887=CIRCLE('',#68057,0.149999999999997) ;
#24888=CIRCLE('',#68059,0.149999999999997) ;
#24889=CIRCLE('',#68060,0.15) ;
#24890=CIRCLE('',#68062,0.149999999999997) ;
#24891=CIRCLE('',#68064,0.15) ;
#24892=CIRCLE('',#68066,0.149999999999997) ;
#24893=CIRCLE('',#68068,0.149999999999997) ;
#24894=CIRCLE('',#68070,0.149999999999997) ;
#24895=CIRCLE('',#68071,0.15) ;
#24896=CIRCLE('',#68073,0.149999999999997) ;
#24897=CIRCLE('',#68075,0.15) ;
#24898=CIRCLE('',#68077,0.149999999999997) ;
#24899=CIRCLE('',#68080,0.149999999999997) ;
#24900=CIRCLE('',#68082,0.15) ;
#24901=CIRCLE('',#68084,0.15) ;
#24902=CIRCLE('',#68085,0.149999999999997) ;
#24903=CIRCLE('',#68087,0.149999999999997) ;
#24904=CIRCLE('',#68088,0.149999999999997) ;
#24905=CIRCLE('',#68092,0.149999999999997) ;
#24906=CIRCLE('',#68094,0.15) ;
#24907=CIRCLE('',#68096,0.15) ;
#24908=CIRCLE('',#68098,0.149999999999997) ;
#24909=CIRCLE('',#68100,0.149999999999997) ;
#24910=CIRCLE('',#68102,0.149999999999997) ;
#24911=CIRCLE('',#68104,0.149999999999997) ;
#24912=CIRCLE('',#68106,0.15) ;
#24913=CIRCLE('',#68108,0.15) ;
#24914=CIRCLE('',#68109,0.149999999999997) ;
#24915=CIRCLE('',#68111,0.149999999999997) ;
#24916=CIRCLE('',#68113,0.149999999999997) ;
#24917=CIRCLE('',#68115,0.15) ;
#24918=CIRCLE('',#68117,0.149999999999997) ;
#24919=CIRCLE('',#68119,0.15) ;
#24920=CIRCLE('',#68121,0.150000000000001) ;
#24921=CIRCLE('',#68123,0.15) ;
#24922=CIRCLE('',#68125,0.150000000000001) ;
#24923=CIRCLE('',#68126,0.150000000000001) ;
#24924=CIRCLE('',#68128,0.149999999999997) ;
#24925=CIRCLE('',#68129,0.15) ;
#24926=CIRCLE('',#68131,0.149999999999997) ;
#24927=CIRCLE('',#68133,0.15) ;
#24928=CIRCLE('',#68135,0.150000000000001) ;
#24929=CIRCLE('',#68137,0.150000000000001) ;
#24930=CIRCLE('',#68139,0.149999999999997) ;
#24931=CIRCLE('',#68141,0.15) ;
#24932=CIRCLE('',#68143,0.149999999999997) ;
#24933=CIRCLE('',#68145,0.150000000000001) ;
#24934=CIRCLE('',#68147,0.15) ;
#24935=CIRCLE('',#68148,0.150000000000001) ;
#24936=CIRCLE('',#68150,0.15) ;
#24937=CIRCLE('',#68151,0.15) ;
#24938=CIRCLE('',#68153,0.149999999999997) ;
#24939=CIRCLE('',#68155,0.150000000000001) ;
#24940=CIRCLE('',#68157,0.150000000000001) ;
#24941=CIRCLE('',#68159,0.15) ;
#24942=CIRCLE('',#68161,0.149999999999997) ;
#24943=CIRCLE('',#68163,0.15) ;
#24944=CIRCLE('',#68165,0.149999999999997) ;
#24945=CIRCLE('',#68167,0.15) ;
#24946=CIRCLE('',#68169,0.15) ;
#24947=CIRCLE('',#68170,0.150000000000001) ;
#24948=CIRCLE('',#68172,0.15) ;
#24949=CIRCLE('',#68173,0.15) ;
#24950=CIRCLE('',#68175,0.15) ;
#24951=CIRCLE('',#68176,0.15) ;
#24952=CIRCLE('',#68178,0.149999999999997) ;
#24953=CIRCLE('',#68180,0.15) ;
#24954=CIRCLE('',#68182,0.150000000000001) ;
#24955=CIRCLE('',#68184,0.150000000000001) ;
#24956=CIRCLE('',#68186,0.15) ;
#24957=CIRCLE('',#68188,0.149999999999997) ;
#24958=CIRCLE('',#68190,0.149999999999997) ;
#24959=CIRCLE('',#68192,0.15) ;
#24960=CIRCLE('',#68194,0.149999999999997) ;
#24961=CIRCLE('',#68196,0.150000000000001) ;
#24962=CIRCLE('',#68198,0.150000000000001) ;
#24963=CIRCLE('',#68200,0.15) ;
#24964=CIRCLE('',#68202,0.149999999999997) ;
#24965=CIRCLE('',#68204,0.150000000000001) ;
#24966=CIRCLE('',#68206,0.150000000000001) ;
#24967=CIRCLE('',#68208,0.15) ;
#24968=CIRCLE('',#68210,0.149999999999997) ;
#24969=CIRCLE('',#68212,0.15) ;
#24970=CIRCLE('',#68214,0.149999999999997) ;
#24971=CIRCLE('',#68216,0.15) ;
#24972=CIRCLE('',#68218,0.15) ;
#24973=CIRCLE('',#68221,0.149999999999997) ;
#24974=CIRCLE('',#68222,0.149999999999997) ;
#24975=CIRCLE('',#68224,0.15) ;
#24976=CIRCLE('',#68225,0.149999999999997) ;
#24977=CIRCLE('',#68227,0.149999999999997) ;
#24978=CIRCLE('',#68228,0.15) ;
#24979=CIRCLE('',#68230,0.15) ;
#24980=CIRCLE('',#68232,0.149999999999997) ;
#24981=CIRCLE('',#68234,0.149999999999997) ;
#24982=CIRCLE('',#68235,0.149999999999997) ;
#24983=CIRCLE('',#68237,0.149999999999997) ;
#24984=CIRCLE('',#68239,0.15) ;
#24985=CIRCLE('',#68241,0.149999999999997) ;
#24986=CIRCLE('',#68242,0.149999999999997) ;
#24987=CIRCLE('',#68244,0.149999999999997) ;
#24988=CIRCLE('',#68246,0.150000000000001) ;
#24989=CIRCLE('',#68248,0.150000000000001) ;
#24990=CIRCLE('',#68250,0.149999999999997) ;
#24991=CIRCLE('',#68252,0.149999999999997) ;
#24992=CIRCLE('',#68254,0.150000000000001) ;
#24993=CIRCLE('',#68256,0.150000000000001) ;
#24994=CIRCLE('',#68258,0.149999999999997) ;
#24995=CIRCLE('',#68260,0.149999999999997) ;
#24996=CIRCLE('',#68262,0.149999999999997) ;
#24997=CIRCLE('',#68265,0.149999999999997) ;
#24998=CIRCLE('',#68266,0.149999999999997) ;
#24999=CIRCLE('',#68268,0.150000000000001) ;
#25000=CIRCLE('',#68269,0.149999999999997) ;
#25001=CIRCLE('',#68271,0.149999999999997) ;
#25002=CIRCLE('',#68272,0.150000000000001) ;
#25003=CIRCLE('',#68274,0.150000000000001) ;
#25004=CIRCLE('',#68276,0.149999999999997) ;
#25005=CIRCLE('',#68278,0.149999999999997) ;
#25006=CIRCLE('',#68279,0.149999999999997) ;
#25007=CIRCLE('',#68281,0.149999999999997) ;
#25008=CIRCLE('',#68283,0.150000000000001) ;
#25009=CIRCLE('',#68285,0.149999999999997) ;
#25010=CIRCLE('',#68286,0.149999999999997) ;
#25011=CIRCLE('',#68288,0.149999999999997) ;
#25012=CIRCLE('',#68290,0.15) ;
#25013=CIRCLE('',#68292,0.15) ;
#25014=CIRCLE('',#68294,0.149999999999997) ;
#25015=CIRCLE('',#68296,0.149999999999997) ;
#25016=CIRCLE('',#68298,0.15) ;
#25017=CIRCLE('',#68300,0.15) ;
#25018=CIRCLE('',#68302,0.149999999999997) ;
#25019=CIRCLE('',#68304,0.149999999999997) ;
#25020=CIRCLE('',#68306,0.149999999999997) ;
#25021=CIRCLE('',#68309,0.149999999999997) ;
#25022=CIRCLE('',#68310,0.149999999999997) ;
#25023=CIRCLE('',#68312,0.15) ;
#25024=CIRCLE('',#68313,0.149999999999997) ;
#25025=CIRCLE('',#68315,0.149999999999997) ;
#25026=CIRCLE('',#68316,0.15) ;
#25027=CIRCLE('',#68318,0.15) ;
#25028=CIRCLE('',#68320,0.149999999999997) ;
#25029=CIRCLE('',#68322,0.149999999999997) ;
#25030=CIRCLE('',#68323,0.149999999999997) ;
#25031=CIRCLE('',#68325,0.149999999999997) ;
#25032=CIRCLE('',#68327,0.15) ;
#25033=CIRCLE('',#68329,0.149999999999997) ;
#25034=CIRCLE('',#68330,0.149999999999997) ;
#25035=CIRCLE('',#68332,0.149999999999997) ;
#25036=CIRCLE('',#68334,0.150000000000001) ;
#25037=CIRCLE('',#68336,0.150000000000001) ;
#25038=CIRCLE('',#68338,0.149999999999997) ;
#25039=CIRCLE('',#68340,0.149999999999997) ;
#25040=CIRCLE('',#68342,0.150000000000001) ;
#25041=CIRCLE('',#68344,0.150000000000001) ;
#25042=CIRCLE('',#68346,0.149999999999997) ;
#25043=CIRCLE('',#68348,0.149999999999997) ;
#25044=CIRCLE('',#68350,0.149999999999997) ;
#25045=CIRCLE('',#68353,0.149999999999997) ;
#25046=CIRCLE('',#68354,0.149999999999997) ;
#25047=CIRCLE('',#68356,0.150000000000001) ;
#25048=CIRCLE('',#68357,0.149999999999997) ;
#25049=CIRCLE('',#68359,0.149999999999997) ;
#25050=CIRCLE('',#68360,0.150000000000001) ;
#25051=CIRCLE('',#68362,0.150000000000001) ;
#25052=CIRCLE('',#68364,0.149999999999997) ;
#25053=CIRCLE('',#68366,0.149999999999997) ;
#25054=CIRCLE('',#68367,0.149999999999997) ;
#25055=CIRCLE('',#68369,0.149999999999997) ;
#25056=CIRCLE('',#68371,0.150000000000001) ;
#25057=CIRCLE('',#68373,0.149999999999997) ;
#25058=CIRCLE('',#68374,0.149999999999997) ;
#25059=CIRCLE('',#68376,0.149999999999997) ;
#25060=CIRCLE('',#68378,0.15) ;
#25061=CIRCLE('',#68380,0.15) ;
#25062=CIRCLE('',#68382,0.149999999999997) ;
#25063=CIRCLE('',#68384,0.149999999999997) ;
#25064=CIRCLE('',#68386,0.15) ;
#25065=CIRCLE('',#68388,0.15) ;
#25066=CIRCLE('',#68390,0.149999999999997) ;
#25067=CIRCLE('',#68392,0.149999999999997) ;
#25068=CIRCLE('',#68394,0.149999999999997) ;
#25069=CIRCLE('',#68397,0.149999999999997) ;
#25070=CIRCLE('',#68398,0.149999999999997) ;
#25071=CIRCLE('',#68400,0.149999999999997) ;
#25072=CIRCLE('',#68401,0.150000000000001) ;
#25073=CIRCLE('',#68403,0.150000000000001) ;
#25074=CIRCLE('',#68404,0.149999999999997) ;
#25075=CIRCLE('',#68406,0.149999999999997) ;
#25076=CIRCLE('',#68408,0.150000000000001) ;
#25077=CIRCLE('',#68410,0.149999999999997) ;
#25078=CIRCLE('',#68411,0.149999999999997) ;
#25079=CIRCLE('',#68413,0.150000000000001) ;
#25080=CIRCLE('',#68415,0.149999999999997) ;
#25081=CIRCLE('',#68417,0.149999999999997) ;
#25082=CIRCLE('',#68418,0.149999999999997) ;
#25083=CIRCLE('',#68420,0.15) ;
#25084=CIRCLE('',#68422,0.149999999999997) ;
#25085=CIRCLE('',#68424,0.149999999999997) ;
#25086=CIRCLE('',#68426,0.15) ;
#25087=CIRCLE('',#68428,0.15) ;
#25088=CIRCLE('',#68430,0.149999999999997) ;
#25089=CIRCLE('',#68432,0.149999999999997) ;
#25090=CIRCLE('',#68434,0.15) ;
#25091=CIRCLE('',#68436,0.149999999999997) ;
#25092=CIRCLE('',#68438,0.149999999999997) ;
#25093=CIRCLE('',#68441,0.149999999999997) ;
#25094=CIRCLE('',#68442,0.149999999999997) ;
#25095=CIRCLE('',#68444,0.149999999999997) ;
#25096=CIRCLE('',#68445,0.149999999999997) ;
#25097=CIRCLE('',#68447,0.149999999999997) ;
#25098=CIRCLE('',#68448,0.149999999999997) ;
#25099=CIRCLE('',#68450,0.149999999999997) ;
#25100=CIRCLE('',#68452,0.149999999999997) ;
#25101=CIRCLE('',#68454,0.149999999999997) ;
#25102=CIRCLE('',#68455,0.149999999999997) ;
#25103=CIRCLE('',#68457,0.149999999999997) ;
#25104=CIRCLE('',#68459,0.149999999999997) ;
#25105=CIRCLE('',#68461,0.149999999999997) ;
#25106=CIRCLE('',#68462,0.149999999999997) ;
#25107=CIRCLE('',#68464,0.149999999999997) ;
#25108=CIRCLE('',#68466,0.149999999999997) ;
#25109=CIRCLE('',#68468,0.149999999999997) ;
#25110=CIRCLE('',#68470,0.149999999999997) ;
#25111=CIRCLE('',#68472,0.149999999999997) ;
#25112=CIRCLE('',#68474,0.149999999999997) ;
#25113=CIRCLE('',#68476,0.149999999999997) ;
#25114=CIRCLE('',#68478,0.149999999999997) ;
#25115=CIRCLE('',#68480,0.149999999999997) ;
#25116=CIRCLE('',#68482,0.149999999999997) ;
#25117=CIRCLE('',#68485,0.149999999999997) ;
#25118=CIRCLE('',#68486,0.149999999999997) ;
#25119=CIRCLE('',#68488,0.149999999999997) ;
#25120=CIRCLE('',#68489,0.149999999999997) ;
#25121=CIRCLE('',#68491,0.149999999999997) ;
#25122=CIRCLE('',#68492,0.149999999999997) ;
#25123=CIRCLE('',#68494,0.149999999999997) ;
#25124=CIRCLE('',#68496,0.149999999999997) ;
#25125=CIRCLE('',#68498,0.149999999999997) ;
#25126=CIRCLE('',#68499,0.149999999999997) ;
#25127=CIRCLE('',#68501,0.149999999999997) ;
#25128=CIRCLE('',#68503,0.149999999999997) ;
#25129=CIRCLE('',#68505,0.149999999999997) ;
#25130=CIRCLE('',#68506,0.149999999999997) ;
#25131=CIRCLE('',#68508,0.149999999999997) ;
#25132=CIRCLE('',#68510,0.149999999999997) ;
#25133=CIRCLE('',#68512,0.149999999999997) ;
#25134=CIRCLE('',#68514,0.149999999999997) ;
#25135=CIRCLE('',#68516,0.149999999999997) ;
#25136=CIRCLE('',#68518,0.149999999999997) ;
#25137=CIRCLE('',#68520,0.149999999999997) ;
#25138=CIRCLE('',#68522,0.149999999999997) ;
#25139=CIRCLE('',#68524,0.149999999999997) ;
#25140=CIRCLE('',#68526,0.149999999999997) ;
#25141=CIRCLE('',#68529,0.149999999999997) ;
#25142=CIRCLE('',#68530,0.149999999999997) ;
#25143=CIRCLE('',#68532,0.149999999999997) ;
#25144=CIRCLE('',#68533,0.149999999999997) ;
#25145=CIRCLE('',#68535,0.149999999999997) ;
#25146=CIRCLE('',#68536,0.149999999999997) ;
#25147=CIRCLE('',#68538,0.149999999999997) ;
#25148=CIRCLE('',#68540,0.149999999999997) ;
#25149=CIRCLE('',#68542,0.149999999999997) ;
#25150=CIRCLE('',#68543,0.149999999999997) ;
#25151=CIRCLE('',#68545,0.149999999999997) ;
#25152=CIRCLE('',#68547,0.149999999999997) ;
#25153=CIRCLE('',#68549,0.149999999999997) ;
#25154=CIRCLE('',#68550,0.149999999999997) ;
#25155=CIRCLE('',#68552,0.149999999999997) ;
#25156=CIRCLE('',#68554,0.149999999999997) ;
#25157=CIRCLE('',#68556,0.149999999999997) ;
#25158=CIRCLE('',#68558,0.149999999999997) ;
#25159=CIRCLE('',#68560,0.149999999999997) ;
#25160=CIRCLE('',#68562,0.149999999999997) ;
#25161=CIRCLE('',#68564,0.149999999999997) ;
#25162=CIRCLE('',#68566,0.149999999999997) ;
#25163=CIRCLE('',#68568,0.149999999999997) ;
#25164=CIRCLE('',#68570,0.149999999999997) ;
#25165=CIRCLE('',#68573,0.149999999999997) ;
#25166=CIRCLE('',#68574,0.149999999999997) ;
#25167=CIRCLE('',#68576,0.150000000000001) ;
#25168=CIRCLE('',#68577,0.149999999999997) ;
#25169=CIRCLE('',#68579,0.149999999999997) ;
#25170=CIRCLE('',#68580,0.150000000000001) ;
#25171=CIRCLE('',#68582,0.150000000000001) ;
#25172=CIRCLE('',#68584,0.149999999999997) ;
#25173=CIRCLE('',#68586,0.149999999999997) ;
#25174=CIRCLE('',#68587,0.149999999999997) ;
#25175=CIRCLE('',#68589,0.149999999999997) ;
#25176=CIRCLE('',#68591,0.150000000000001) ;
#25177=CIRCLE('',#68593,0.149999999999997) ;
#25178=CIRCLE('',#68594,0.149999999999997) ;
#25179=CIRCLE('',#68596,0.149999999999997) ;
#25180=CIRCLE('',#68598,0.150000000000001) ;
#25181=CIRCLE('',#68600,0.150000000000001) ;
#25182=CIRCLE('',#68602,0.149999999999997) ;
#25183=CIRCLE('',#68604,0.149999999999997) ;
#25184=CIRCLE('',#68606,0.150000000000001) ;
#25185=CIRCLE('',#68608,0.150000000000001) ;
#25186=CIRCLE('',#68610,0.149999999999997) ;
#25187=CIRCLE('',#68612,0.149999999999997) ;
#25188=CIRCLE('',#68614,0.149999999999997) ;
#25189=CIRCLE('',#68617,0.149999999999997) ;
#25190=CIRCLE('',#68618,0.149999999999997) ;
#25191=CIRCLE('',#68620,0.150000000000001) ;
#25192=CIRCLE('',#68621,0.149999999999997) ;
#25193=CIRCLE('',#68623,0.149999999999997) ;
#25194=CIRCLE('',#68624,0.150000000000001) ;
#25195=CIRCLE('',#68626,0.150000000000001) ;
#25196=CIRCLE('',#68628,0.149999999999997) ;
#25197=CIRCLE('',#68630,0.149999999999997) ;
#25198=CIRCLE('',#68631,0.149999999999997) ;
#25199=CIRCLE('',#68633,0.149999999999997) ;
#25200=CIRCLE('',#68635,0.150000000000001) ;
#25201=CIRCLE('',#68637,0.149999999999997) ;
#25202=CIRCLE('',#68638,0.149999999999997) ;
#25203=CIRCLE('',#68640,0.149999999999997) ;
#25204=CIRCLE('',#68642,0.150000000000001) ;
#25205=CIRCLE('',#68644,0.150000000000001) ;
#25206=CIRCLE('',#68646,0.149999999999997) ;
#25207=CIRCLE('',#68648,0.149999999999997) ;
#25208=CIRCLE('',#68650,0.150000000000001) ;
#25209=CIRCLE('',#68652,0.150000000000001) ;
#25210=CIRCLE('',#68654,0.149999999999997) ;
#25211=CIRCLE('',#68656,0.149999999999997) ;
#25212=CIRCLE('',#68658,0.149999999999997) ;
#25213=CIRCLE('',#68661,0.149999999999997) ;
#25214=CIRCLE('',#68662,0.149999999999997) ;
#25215=CIRCLE('',#68664,0.150000000000001) ;
#25216=CIRCLE('',#68665,0.149999999999997) ;
#25217=CIRCLE('',#68667,0.149999999999997) ;
#25218=CIRCLE('',#68668,0.150000000000001) ;
#25219=CIRCLE('',#68670,0.150000000000001) ;
#25220=CIRCLE('',#68672,0.149999999999997) ;
#25221=CIRCLE('',#68674,0.149999999999997) ;
#25222=CIRCLE('',#68675,0.149999999999997) ;
#25223=CIRCLE('',#68677,0.149999999999997) ;
#25224=CIRCLE('',#68679,0.150000000000001) ;
#25225=CIRCLE('',#68681,0.149999999999997) ;
#25226=CIRCLE('',#68682,0.149999999999997) ;
#25227=CIRCLE('',#68684,0.149999999999997) ;
#25228=CIRCLE('',#68686,0.150000000000001) ;
#25229=CIRCLE('',#68688,0.150000000000001) ;
#25230=CIRCLE('',#68690,0.149999999999997) ;
#25231=CIRCLE('',#68692,0.149999999999997) ;
#25232=CIRCLE('',#68694,0.150000000000001) ;
#25233=CIRCLE('',#68696,0.150000000000001) ;
#25234=CIRCLE('',#68698,0.149999999999997) ;
#25235=CIRCLE('',#68700,0.149999999999997) ;
#25236=CIRCLE('',#68702,0.149999999999997) ;
#25237=CIRCLE('',#68705,0.149999999999997) ;
#25238=CIRCLE('',#68706,0.149999999999997) ;
#25239=CIRCLE('',#68708,0.150000000000001) ;
#25240=CIRCLE('',#68709,0.149999999999997) ;
#25241=CIRCLE('',#68711,0.149999999999997) ;
#25242=CIRCLE('',#68712,0.15) ;
#25243=CIRCLE('',#68714,0.150000000000001) ;
#25244=CIRCLE('',#68716,0.149999999999997) ;
#25245=CIRCLE('',#68718,0.149999999999997) ;
#25246=CIRCLE('',#68719,0.149999999999997) ;
#25247=CIRCLE('',#68721,0.149999999999997) ;
#25248=CIRCLE('',#68723,0.15) ;
#25249=CIRCLE('',#68725,0.149999999999997) ;
#25250=CIRCLE('',#68726,0.149999999999997) ;
#25251=CIRCLE('',#68728,0.149999999999997) ;
#25252=CIRCLE('',#68730,0.150000000000001) ;
#25253=CIRCLE('',#68732,0.15) ;
#25254=CIRCLE('',#68734,0.149999999999997) ;
#25255=CIRCLE('',#68736,0.149999999999997) ;
#25256=CIRCLE('',#68738,0.150000000000001) ;
#25257=CIRCLE('',#68740,0.15) ;
#25258=CIRCLE('',#68742,0.149999999999997) ;
#25259=CIRCLE('',#68744,0.149999999999997) ;
#25260=CIRCLE('',#68746,0.149999999999997) ;
#25261=CIRCLE('',#68750,0.149999999999997) ;
#25262=CIRCLE('',#68752,0.149999999999997) ;
#25263=CIRCLE('',#68755,0.150000000000001) ;
#25264=CIRCLE('',#68756,0.149999999999997) ;
#25265=CIRCLE('',#68758,0.149999999999997) ;
#25266=CIRCLE('',#68764,0.149999999999997) ;
#25267=CIRCLE('',#68766,0.149999999999997) ;
#25268=CIRCLE('',#68768,0.149999999999997) ;
#25269=CIRCLE('',#68770,0.149999999999997) ;
#25270=CIRCLE('',#68772,0.149999999999997) ;
#25271=CIRCLE('',#68774,0.149999999999997) ;
#25272=CIRCLE('',#68776,0.149999999999997) ;
#29494=VERTEX_POINT('',#99149) ;
#29495=VERTEX_POINT('',#99150) ;
#29496=VERTEX_POINT('',#99153) ;
#29497=VERTEX_POINT('',#99157) ;
#29498=VERTEX_POINT('',#99159) ;
#29499=VERTEX_POINT('',#99161) ;
#29500=VERTEX_POINT('',#99165) ;
#29501=VERTEX_POINT('',#99166) ;
#29502=VERTEX_POINT('',#99169) ;
#29503=VERTEX_POINT('',#99171) ;
#29504=VERTEX_POINT('',#99175) ;
#29505=VERTEX_POINT('',#99177) ;
#29506=VERTEX_POINT('',#99181) ;
#29507=VERTEX_POINT('',#99182) ;
#29508=VERTEX_POINT('',#99185) ;
#29509=VERTEX_POINT('',#99187) ;
#29510=VERTEX_POINT('',#99191) ;
#29511=VERTEX_POINT('',#99193) ;
#29512=VERTEX_POINT('',#99197) ;
#29513=VERTEX_POINT('',#99203) ;
#29514=VERTEX_POINT('',#99211) ;
#29515=VERTEX_POINT('',#99212) ;
#29516=VERTEX_POINT('',#99214) ;
#29517=VERTEX_POINT('',#99216) ;
#29518=VERTEX_POINT('',#99218) ;
#29519=VERTEX_POINT('',#99220) ;
#29520=VERTEX_POINT('',#99223) ;
#29521=VERTEX_POINT('',#99224) ;
#29522=VERTEX_POINT('',#99226) ;
#29523=VERTEX_POINT('',#99228) ;
#29524=VERTEX_POINT('',#99230) ;
#29525=VERTEX_POINT('',#99232) ;
#29526=VERTEX_POINT('',#99234) ;
#29527=VERTEX_POINT('',#99236) ;
#29528=VERTEX_POINT('',#99240) ;
#29529=VERTEX_POINT('',#99241) ;
#29530=VERTEX_POINT('',#99243) ;
#29531=VERTEX_POINT('',#99245) ;
#29532=VERTEX_POINT('',#99247) ;
#29533=VERTEX_POINT('',#99249) ;
#29534=VERTEX_POINT('',#99252) ;
#29535=VERTEX_POINT('',#99253) ;
#29536=VERTEX_POINT('',#99255) ;
#29537=VERTEX_POINT('',#99257) ;
#29538=VERTEX_POINT('',#99259) ;
#29539=VERTEX_POINT('',#99261) ;
#29540=VERTEX_POINT('',#99263) ;
#29541=VERTEX_POINT('',#99265) ;
#29542=VERTEX_POINT('',#99269) ;
#29543=VERTEX_POINT('',#99270) ;
#29544=VERTEX_POINT('',#99272) ;
#29545=VERTEX_POINT('',#99274) ;
#29546=VERTEX_POINT('',#99276) ;
#29547=VERTEX_POINT('',#99278) ;
#29548=VERTEX_POINT('',#99280) ;
#29549=VERTEX_POINT('',#99282) ;
#29550=VERTEX_POINT('',#99284) ;
#29551=VERTEX_POINT('',#99286) ;
#29552=VERTEX_POINT('',#99288) ;
#29553=VERTEX_POINT('',#99291) ;
#29554=VERTEX_POINT('',#99292) ;
#29555=VERTEX_POINT('',#99294) ;
#29556=VERTEX_POINT('',#99296) ;
#29557=VERTEX_POINT('',#99298) ;
#29558=VERTEX_POINT('',#99300) ;
#29559=VERTEX_POINT('',#99302) ;
#29560=VERTEX_POINT('',#99304) ;
#29561=VERTEX_POINT('',#99307) ;
#29562=VERTEX_POINT('',#99308) ;
#29563=VERTEX_POINT('',#99310) ;
#29564=VERTEX_POINT('',#99312) ;
#29565=VERTEX_POINT('',#99314) ;
#29566=VERTEX_POINT('',#99316) ;
#29567=VERTEX_POINT('',#99318) ;
#29568=VERTEX_POINT('',#99320) ;
#29569=VERTEX_POINT('',#99323) ;
#29570=VERTEX_POINT('',#99324) ;
#29571=VERTEX_POINT('',#99326) ;
#29572=VERTEX_POINT('',#99328) ;
#29573=VERTEX_POINT('',#99330) ;
#29574=VERTEX_POINT('',#99332) ;
#29575=VERTEX_POINT('',#99334) ;
#29576=VERTEX_POINT('',#99336) ;
#29577=VERTEX_POINT('',#99339) ;
#29578=VERTEX_POINT('',#99340) ;
#29579=VERTEX_POINT('',#99342) ;
#29580=VERTEX_POINT('',#99344) ;
#29581=VERTEX_POINT('',#99346) ;
#29582=VERTEX_POINT('',#99348) ;
#29583=VERTEX_POINT('',#99350) ;
#29584=VERTEX_POINT('',#99352) ;
#29585=VERTEX_POINT('',#99356) ;
#29586=VERTEX_POINT('',#99357) ;
#29587=VERTEX_POINT('',#99359) ;
#29588=VERTEX_POINT('',#99361) ;
#29589=VERTEX_POINT('',#99363) ;
#29590=VERTEX_POINT('',#99365) ;
#29591=VERTEX_POINT('',#99367) ;
#29592=VERTEX_POINT('',#99369) ;
#29593=VERTEX_POINT('',#99371) ;
#29594=VERTEX_POINT('',#99373) ;
#29595=VERTEX_POINT('',#99375) ;
#29596=VERTEX_POINT('',#99378) ;
#29597=VERTEX_POINT('',#99379) ;
#29598=VERTEX_POINT('',#99381) ;
#29599=VERTEX_POINT('',#99383) ;
#29600=VERTEX_POINT('',#99385) ;
#29601=VERTEX_POINT('',#99387) ;
#29602=VERTEX_POINT('',#99389) ;
#29603=VERTEX_POINT('',#99391) ;
#29604=VERTEX_POINT('',#99394) ;
#29605=VERTEX_POINT('',#99395) ;
#29606=VERTEX_POINT('',#99397) ;
#29607=VERTEX_POINT('',#99399) ;
#29608=VERTEX_POINT('',#99401) ;
#29609=VERTEX_POINT('',#99403) ;
#29610=VERTEX_POINT('',#99405) ;
#29611=VERTEX_POINT('',#99407) ;
#29612=VERTEX_POINT('',#99410) ;
#29613=VERTEX_POINT('',#99411) ;
#29614=VERTEX_POINT('',#99413) ;
#29615=VERTEX_POINT('',#99415) ;
#29616=VERTEX_POINT('',#99417) ;
#29617=VERTEX_POINT('',#99419) ;
#29618=VERTEX_POINT('',#99421) ;
#29619=VERTEX_POINT('',#99423) ;
#29620=VERTEX_POINT('',#99426) ;
#29621=VERTEX_POINT('',#99427) ;
#29622=VERTEX_POINT('',#99429) ;
#29623=VERTEX_POINT('',#99431) ;
#29624=VERTEX_POINT('',#99433) ;
#29625=VERTEX_POINT('',#99435) ;
#29626=VERTEX_POINT('',#99437) ;
#29627=VERTEX_POINT('',#99439) ;
#29628=VERTEX_POINT('',#99443) ;
#29629=VERTEX_POINT('',#99444) ;
#29630=VERTEX_POINT('',#99446) ;
#29631=VERTEX_POINT('',#99448) ;
#29632=VERTEX_POINT('',#99450) ;
#29633=VERTEX_POINT('',#99452) ;
#29634=VERTEX_POINT('',#99454) ;
#29635=VERTEX_POINT('',#99456) ;
#29636=VERTEX_POINT('',#99458) ;
#29637=VERTEX_POINT('',#99460) ;
#29638=VERTEX_POINT('',#99462) ;
#29639=VERTEX_POINT('',#99465) ;
#29640=VERTEX_POINT('',#99466) ;
#29641=VERTEX_POINT('',#99468) ;
#29642=VERTEX_POINT('',#99470) ;
#29643=VERTEX_POINT('',#99472) ;
#29644=VERTEX_POINT('',#99474) ;
#29645=VERTEX_POINT('',#99476) ;
#29646=VERTEX_POINT('',#99478) ;
#29647=VERTEX_POINT('',#99481) ;
#29648=VERTEX_POINT('',#99482) ;
#29649=VERTEX_POINT('',#99484) ;
#29650=VERTEX_POINT('',#99486) ;
#29651=VERTEX_POINT('',#99488) ;
#29652=VERTEX_POINT('',#99490) ;
#29653=VERTEX_POINT('',#99492) ;
#29654=VERTEX_POINT('',#99494) ;
#29655=VERTEX_POINT('',#99497) ;
#29656=VERTEX_POINT('',#99498) ;
#29657=VERTEX_POINT('',#99500) ;
#29658=VERTEX_POINT('',#99502) ;
#29659=VERTEX_POINT('',#99504) ;
#29660=VERTEX_POINT('',#99506) ;
#29661=VERTEX_POINT('',#99508) ;
#29662=VERTEX_POINT('',#99510) ;
#29663=VERTEX_POINT('',#99513) ;
#29664=VERTEX_POINT('',#99514) ;
#29665=VERTEX_POINT('',#99516) ;
#29666=VERTEX_POINT('',#99518) ;
#29667=VERTEX_POINT('',#99520) ;
#29668=VERTEX_POINT('',#99522) ;
#29669=VERTEX_POINT('',#99524) ;
#29670=VERTEX_POINT('',#99526) ;
#29671=VERTEX_POINT('',#99529) ;
#29672=VERTEX_POINT('',#99530) ;
#29673=VERTEX_POINT('',#99532) ;
#29674=VERTEX_POINT('',#99534) ;
#29675=VERTEX_POINT('',#99536) ;
#29676=VERTEX_POINT('',#99538) ;
#29677=VERTEX_POINT('',#99540) ;
#29678=VERTEX_POINT('',#99542) ;
#29679=VERTEX_POINT('',#99545) ;
#29680=VERTEX_POINT('',#99546) ;
#29681=VERTEX_POINT('',#99548) ;
#29682=VERTEX_POINT('',#99550) ;
#29683=VERTEX_POINT('',#99552) ;
#29684=VERTEX_POINT('',#99554) ;
#29685=VERTEX_POINT('',#99556) ;
#29686=VERTEX_POINT('',#99558) ;
#29687=VERTEX_POINT('',#99561) ;
#29688=VERTEX_POINT('',#99562) ;
#29689=VERTEX_POINT('',#99564) ;
#29690=VERTEX_POINT('',#99566) ;
#29691=VERTEX_POINT('',#99568) ;
#29692=VERTEX_POINT('',#99570) ;
#29693=VERTEX_POINT('',#99572) ;
#29694=VERTEX_POINT('',#99574) ;
#29695=VERTEX_POINT('',#99578) ;
#29696=VERTEX_POINT('',#99579) ;
#29697=VERTEX_POINT('',#99581) ;
#29698=VERTEX_POINT('',#99583) ;
#29699=VERTEX_POINT('',#99585) ;
#29700=VERTEX_POINT('',#99587) ;
#29701=VERTEX_POINT('',#99589) ;
#29702=VERTEX_POINT('',#99591) ;
#29703=VERTEX_POINT('',#99593) ;
#29704=VERTEX_POINT('',#99595) ;
#29705=VERTEX_POINT('',#99597) ;
#29706=VERTEX_POINT('',#99600) ;
#29707=VERTEX_POINT('',#99601) ;
#29708=VERTEX_POINT('',#99603) ;
#29709=VERTEX_POINT('',#99605) ;
#29710=VERTEX_POINT('',#99607) ;
#29711=VERTEX_POINT('',#99609) ;
#29712=VERTEX_POINT('',#99611) ;
#29713=VERTEX_POINT('',#99613) ;
#29714=VERTEX_POINT('',#99616) ;
#29715=VERTEX_POINT('',#99617) ;
#29716=VERTEX_POINT('',#99619) ;
#29717=VERTEX_POINT('',#99621) ;
#29718=VERTEX_POINT('',#99623) ;
#29719=VERTEX_POINT('',#99625) ;
#29720=VERTEX_POINT('',#99627) ;
#29721=VERTEX_POINT('',#99629) ;
#29722=VERTEX_POINT('',#99632) ;
#29723=VERTEX_POINT('',#99633) ;
#29724=VERTEX_POINT('',#99635) ;
#29725=VERTEX_POINT('',#99637) ;
#29726=VERTEX_POINT('',#99639) ;
#29727=VERTEX_POINT('',#99641) ;
#29728=VERTEX_POINT('',#99643) ;
#29729=VERTEX_POINT('',#99645) ;
#29730=VERTEX_POINT('',#99648) ;
#29731=VERTEX_POINT('',#99649) ;
#29732=VERTEX_POINT('',#99651) ;
#29733=VERTEX_POINT('',#99653) ;
#29734=VERTEX_POINT('',#99655) ;
#29735=VERTEX_POINT('',#99657) ;
#29736=VERTEX_POINT('',#99659) ;
#29737=VERTEX_POINT('',#99661) ;
#29738=VERTEX_POINT('',#99664) ;
#29739=VERTEX_POINT('',#99665) ;
#29740=VERTEX_POINT('',#99667) ;
#29741=VERTEX_POINT('',#99669) ;
#29742=VERTEX_POINT('',#99671) ;
#29743=VERTEX_POINT('',#99673) ;
#29744=VERTEX_POINT('',#99675) ;
#29745=VERTEX_POINT('',#99677) ;
#29746=VERTEX_POINT('',#99680) ;
#29747=VERTEX_POINT('',#99681) ;
#29748=VERTEX_POINT('',#99683) ;
#29749=VERTEX_POINT('',#99685) ;
#29750=VERTEX_POINT('',#99687) ;
#29751=VERTEX_POINT('',#99689) ;
#29752=VERTEX_POINT('',#99691) ;
#29753=VERTEX_POINT('',#99693) ;
#29754=VERTEX_POINT('',#99696) ;
#29755=VERTEX_POINT('',#99697) ;
#29756=VERTEX_POINT('',#99699) ;
#29757=VERTEX_POINT('',#99701) ;
#29758=VERTEX_POINT('',#99703) ;
#29759=VERTEX_POINT('',#99705) ;
#29760=VERTEX_POINT('',#99707) ;
#29761=VERTEX_POINT('',#99709) ;
#29762=VERTEX_POINT('',#99713) ;
#29763=VERTEX_POINT('',#99714) ;
#29764=VERTEX_POINT('',#99716) ;
#29765=VERTEX_POINT('',#99718) ;
#29766=VERTEX_POINT('',#99720) ;
#29767=VERTEX_POINT('',#99722) ;
#29768=VERTEX_POINT('',#99724) ;
#29769=VERTEX_POINT('',#99726) ;
#29770=VERTEX_POINT('',#99728) ;
#29771=VERTEX_POINT('',#99730) ;
#29772=VERTEX_POINT('',#99734) ;
#29773=VERTEX_POINT('',#99735) ;
#29774=VERTEX_POINT('',#99737) ;
#29775=VERTEX_POINT('',#99739) ;
#29776=VERTEX_POINT('',#99741) ;
#29777=VERTEX_POINT('',#99743) ;
#29778=VERTEX_POINT('',#99745) ;
#29779=VERTEX_POINT('',#99747) ;
#29780=VERTEX_POINT('',#99749) ;
#29781=VERTEX_POINT('',#99751) ;
#29782=VERTEX_POINT('',#99755) ;
#29783=VERTEX_POINT('',#99756) ;
#29784=VERTEX_POINT('',#99758) ;
#29785=VERTEX_POINT('',#99760) ;
#29786=VERTEX_POINT('',#99764) ;
#29787=VERTEX_POINT('',#99765) ;
#29788=VERTEX_POINT('',#99767) ;
#29789=VERTEX_POINT('',#99769) ;
#29790=VERTEX_POINT('',#99773) ;
#29791=VERTEX_POINT('',#99774) ;
#29792=VERTEX_POINT('',#99776) ;
#29793=VERTEX_POINT('',#99778) ;
#29794=VERTEX_POINT('',#99782) ;
#29795=VERTEX_POINT('',#99783) ;
#29796=VERTEX_POINT('',#99785) ;
#29797=VERTEX_POINT('',#99787) ;
#29798=VERTEX_POINT('',#99791) ;
#29799=VERTEX_POINT('',#99792) ;
#29800=VERTEX_POINT('',#99794) ;
#29801=VERTEX_POINT('',#99796) ;
#29802=VERTEX_POINT('',#99800) ;
#29803=VERTEX_POINT('',#99802) ;
#29804=VERTEX_POINT('',#99815) ;
#29805=VERTEX_POINT('',#99816) ;
#29806=VERTEX_POINT('',#99818) ;
#29807=VERTEX_POINT('',#99820) ;
#29808=VERTEX_POINT('',#99824) ;
#29809=VERTEX_POINT('',#99825) ;
#29810=VERTEX_POINT('',#99827) ;
#29811=VERTEX_POINT('',#99829) ;
#29812=VERTEX_POINT('',#99833) ;
#29813=VERTEX_POINT('',#99834) ;
#29814=VERTEX_POINT('',#99836) ;
#29815=VERTEX_POINT('',#99838) ;
#29816=VERTEX_POINT('',#99842) ;
#29817=VERTEX_POINT('',#99843) ;
#29818=VERTEX_POINT('',#99845) ;
#29819=VERTEX_POINT('',#99847) ;
#29820=VERTEX_POINT('',#99851) ;
#29821=VERTEX_POINT('',#99852) ;
#29822=VERTEX_POINT('',#99854) ;
#29823=VERTEX_POINT('',#99856) ;
#29824=VERTEX_POINT('',#99860) ;
#29825=VERTEX_POINT('',#99861) ;
#29826=VERTEX_POINT('',#99863) ;
#29827=VERTEX_POINT('',#99865) ;
#29828=VERTEX_POINT('',#99869) ;
#29829=VERTEX_POINT('',#99871) ;
#29830=VERTEX_POINT('',#99877) ;
#29831=VERTEX_POINT('',#99878) ;
#29832=VERTEX_POINT('',#99880) ;
#29833=VERTEX_POINT('',#99882) ;
#29834=VERTEX_POINT('',#99886) ;
#29835=VERTEX_POINT('',#99887) ;
#29836=VERTEX_POINT('',#99889) ;
#29837=VERTEX_POINT('',#99891) ;
#29838=VERTEX_POINT('',#99895) ;
#29839=VERTEX_POINT('',#99896) ;
#29840=VERTEX_POINT('',#99898) ;
#29841=VERTEX_POINT('',#99900) ;
#29842=VERTEX_POINT('',#99919) ;
#29843=VERTEX_POINT('',#99920) ;
#29844=VERTEX_POINT('',#99933) ;
#29845=VERTEX_POINT('',#99934) ;
#29846=VERTEX_POINT('',#99936) ;
#29847=VERTEX_POINT('',#99938) ;
#29848=VERTEX_POINT('',#99942) ;
#29849=VERTEX_POINT('',#99943) ;
#29850=VERTEX_POINT('',#99945) ;
#29851=VERTEX_POINT('',#99947) ;
#29852=VERTEX_POINT('',#99951) ;
#29853=VERTEX_POINT('',#99952) ;
#29854=VERTEX_POINT('',#99954) ;
#29855=VERTEX_POINT('',#99956) ;
#29856=VERTEX_POINT('',#99960) ;
#29857=VERTEX_POINT('',#99961) ;
#29858=VERTEX_POINT('',#99963) ;
#29859=VERTEX_POINT('',#99965) ;
#29860=VERTEX_POINT('',#99969) ;
#29861=VERTEX_POINT('',#99970) ;
#29862=VERTEX_POINT('',#99972) ;
#29863=VERTEX_POINT('',#99974) ;
#29864=VERTEX_POINT('',#99978) ;
#29865=VERTEX_POINT('',#99979) ;
#29866=VERTEX_POINT('',#99981) ;
#29867=VERTEX_POINT('',#99983) ;
#29868=VERTEX_POINT('',#99989) ;
#29869=VERTEX_POINT('',#99990) ;
#29870=VERTEX_POINT('',#99995) ;
#29871=VERTEX_POINT('',#99996) ;
#29872=VERTEX_POINT('',#99998) ;
#29873=VERTEX_POINT('',#100000) ;
#29874=VERTEX_POINT('',#100004) ;
#29875=VERTEX_POINT('',#100005) ;
#29876=VERTEX_POINT('',#100007) ;
#29877=VERTEX_POINT('',#100009) ;
#29878=VERTEX_POINT('',#100013) ;
#29879=VERTEX_POINT('',#100014) ;
#29880=VERTEX_POINT('',#100016) ;
#29881=VERTEX_POINT('',#100018) ;
#29882=VERTEX_POINT('',#100022) ;
#29883=VERTEX_POINT('',#100023) ;
#29884=VERTEX_POINT('',#100025) ;
#29885=VERTEX_POINT('',#100027) ;
#29886=VERTEX_POINT('',#100031) ;
#29887=VERTEX_POINT('',#100032) ;
#29888=VERTEX_POINT('',#100034) ;
#29889=VERTEX_POINT('',#100036) ;
#29890=VERTEX_POINT('',#100040) ;
#29891=VERTEX_POINT('',#100041) ;
#29892=VERTEX_POINT('',#100043) ;
#29893=VERTEX_POINT('',#100045) ;
#29894=VERTEX_POINT('',#100049) ;
#29895=VERTEX_POINT('',#100050) ;
#29896=VERTEX_POINT('',#100052) ;
#29897=VERTEX_POINT('',#100054) ;
#29898=VERTEX_POINT('',#100058) ;
#29899=VERTEX_POINT('',#100059) ;
#29900=VERTEX_POINT('',#100061) ;
#29901=VERTEX_POINT('',#100063) ;
#29902=VERTEX_POINT('',#100067) ;
#29903=VERTEX_POINT('',#100068) ;
#29904=VERTEX_POINT('',#100070) ;
#29905=VERTEX_POINT('',#100072) ;
#29906=VERTEX_POINT('',#100076) ;
#29907=VERTEX_POINT('',#100077) ;
#29908=VERTEX_POINT('',#100079) ;
#29909=VERTEX_POINT('',#100081) ;
#29910=VERTEX_POINT('',#100085) ;
#29911=VERTEX_POINT('',#100086) ;
#29912=VERTEX_POINT('',#100088) ;
#29913=VERTEX_POINT('',#100090) ;
#29914=VERTEX_POINT('',#100094) ;
#29915=VERTEX_POINT('',#100095) ;
#29916=VERTEX_POINT('',#100097) ;
#29917=VERTEX_POINT('',#100099) ;
#29918=VERTEX_POINT('',#100103) ;
#29919=VERTEX_POINT('',#100104) ;
#29920=VERTEX_POINT('',#100106) ;
#29921=VERTEX_POINT('',#100108) ;
#29922=VERTEX_POINT('',#100112) ;
#29923=VERTEX_POINT('',#100113) ;
#29924=VERTEX_POINT('',#100115) ;
#29925=VERTEX_POINT('',#100117) ;
#29926=VERTEX_POINT('',#100121) ;
#29927=VERTEX_POINT('',#100122) ;
#29928=VERTEX_POINT('',#100124) ;
#29929=VERTEX_POINT('',#100126) ;
#29930=VERTEX_POINT('',#100130) ;
#29931=VERTEX_POINT('',#100131) ;
#29932=VERTEX_POINT('',#100133) ;
#29933=VERTEX_POINT('',#100135) ;
#29934=VERTEX_POINT('',#100139) ;
#29935=VERTEX_POINT('',#100140) ;
#29936=VERTEX_POINT('',#100142) ;
#29937=VERTEX_POINT('',#100144) ;
#29938=VERTEX_POINT('',#100148) ;
#29939=VERTEX_POINT('',#100149) ;
#29940=VERTEX_POINT('',#100151) ;
#29941=VERTEX_POINT('',#100153) ;
#29942=VERTEX_POINT('',#100157) ;
#29943=VERTEX_POINT('',#100158) ;
#29944=VERTEX_POINT('',#100160) ;
#29945=VERTEX_POINT('',#100162) ;
#29946=VERTEX_POINT('',#100166) ;
#29947=VERTEX_POINT('',#100167) ;
#29948=VERTEX_POINT('',#100169) ;
#29949=VERTEX_POINT('',#100171) ;
#29950=VERTEX_POINT('',#100175) ;
#29951=VERTEX_POINT('',#100176) ;
#29952=VERTEX_POINT('',#100178) ;
#29953=VERTEX_POINT('',#100180) ;
#29954=VERTEX_POINT('',#100184) ;
#29955=VERTEX_POINT('',#100185) ;
#29956=VERTEX_POINT('',#100187) ;
#29957=VERTEX_POINT('',#100189) ;
#29958=VERTEX_POINT('',#100193) ;
#29959=VERTEX_POINT('',#100194) ;
#29960=VERTEX_POINT('',#100196) ;
#29961=VERTEX_POINT('',#100198) ;
#29962=VERTEX_POINT('',#100202) ;
#29963=VERTEX_POINT('',#100203) ;
#29964=VERTEX_POINT('',#100205) ;
#29965=VERTEX_POINT('',#100207) ;
#29966=VERTEX_POINT('',#100211) ;
#29967=VERTEX_POINT('',#100212) ;
#29968=VERTEX_POINT('',#100214) ;
#29969=VERTEX_POINT('',#100216) ;
#29970=VERTEX_POINT('',#100220) ;
#29971=VERTEX_POINT('',#100221) ;
#29972=VERTEX_POINT('',#100223) ;
#29973=VERTEX_POINT('',#100225) ;
#29974=VERTEX_POINT('',#100229) ;
#29975=VERTEX_POINT('',#100230) ;
#29976=VERTEX_POINT('',#100232) ;
#29977=VERTEX_POINT('',#100234) ;
#29978=VERTEX_POINT('',#100238) ;
#29979=VERTEX_POINT('',#100239) ;
#29980=VERTEX_POINT('',#100241) ;
#29981=VERTEX_POINT('',#100243) ;
#29982=VERTEX_POINT('',#100247) ;
#29983=VERTEX_POINT('',#100248) ;
#29984=VERTEX_POINT('',#100250) ;
#29985=VERTEX_POINT('',#100252) ;
#29986=VERTEX_POINT('',#100256) ;
#29987=VERTEX_POINT('',#100257) ;
#29988=VERTEX_POINT('',#100259) ;
#29989=VERTEX_POINT('',#100261) ;
#29990=VERTEX_POINT('',#100265) ;
#29991=VERTEX_POINT('',#100266) ;
#29992=VERTEX_POINT('',#100268) ;
#29993=VERTEX_POINT('',#100270) ;
#29994=VERTEX_POINT('',#100274) ;
#29995=VERTEX_POINT('',#100275) ;
#29996=VERTEX_POINT('',#100277) ;
#29997=VERTEX_POINT('',#100279) ;
#29998=VERTEX_POINT('',#100283) ;
#29999=VERTEX_POINT('',#100284) ;
#30000=VERTEX_POINT('',#100286) ;
#30001=VERTEX_POINT('',#100288) ;
#30002=VERTEX_POINT('',#100292) ;
#30003=VERTEX_POINT('',#100293) ;
#30004=VERTEX_POINT('',#100295) ;
#30005=VERTEX_POINT('',#100297) ;
#30006=VERTEX_POINT('',#100301) ;
#30007=VERTEX_POINT('',#100302) ;
#30008=VERTEX_POINT('',#100304) ;
#30009=VERTEX_POINT('',#100306) ;
#30010=VERTEX_POINT('',#100310) ;
#30011=VERTEX_POINT('',#100311) ;
#30012=VERTEX_POINT('',#100313) ;
#30013=VERTEX_POINT('',#100315) ;
#30014=VERTEX_POINT('',#100319) ;
#30015=VERTEX_POINT('',#100320) ;
#30016=VERTEX_POINT('',#100322) ;
#30017=VERTEX_POINT('',#100324) ;
#30018=VERTEX_POINT('',#100328) ;
#30019=VERTEX_POINT('',#100329) ;
#30020=VERTEX_POINT('',#100331) ;
#30021=VERTEX_POINT('',#100333) ;
#30022=VERTEX_POINT('',#100337) ;
#30023=VERTEX_POINT('',#100338) ;
#30024=VERTEX_POINT('',#100340) ;
#30025=VERTEX_POINT('',#100342) ;
#30026=VERTEX_POINT('',#100346) ;
#30027=VERTEX_POINT('',#100347) ;
#30028=VERTEX_POINT('',#100349) ;
#30029=VERTEX_POINT('',#100351) ;
#30030=VERTEX_POINT('',#100355) ;
#30031=VERTEX_POINT('',#100356) ;
#30032=VERTEX_POINT('',#100358) ;
#30033=VERTEX_POINT('',#100360) ;
#30034=VERTEX_POINT('',#100364) ;
#30035=VERTEX_POINT('',#100365) ;
#30036=VERTEX_POINT('',#100367) ;
#30037=VERTEX_POINT('',#100369) ;
#30038=VERTEX_POINT('',#100373) ;
#30039=VERTEX_POINT('',#100374) ;
#30040=VERTEX_POINT('',#100376) ;
#30041=VERTEX_POINT('',#100378) ;
#30042=VERTEX_POINT('',#100382) ;
#30043=VERTEX_POINT('',#100383) ;
#30044=VERTEX_POINT('',#100385) ;
#30045=VERTEX_POINT('',#100387) ;
#30046=VERTEX_POINT('',#100391) ;
#30047=VERTEX_POINT('',#100392) ;
#30048=VERTEX_POINT('',#100394) ;
#30049=VERTEX_POINT('',#100396) ;
#30050=VERTEX_POINT('',#100400) ;
#30051=VERTEX_POINT('',#100401) ;
#30052=VERTEX_POINT('',#100403) ;
#30053=VERTEX_POINT('',#100405) ;
#30054=VERTEX_POINT('',#100409) ;
#30055=VERTEX_POINT('',#100410) ;
#30056=VERTEX_POINT('',#100412) ;
#30057=VERTEX_POINT('',#100414) ;
#30058=VERTEX_POINT('',#100418) ;
#30059=VERTEX_POINT('',#100419) ;
#30060=VERTEX_POINT('',#100421) ;
#30061=VERTEX_POINT('',#100423) ;
#34692=EDGE_CURVE('',#29494,#29495,#24719,.T.) ;
#34693=EDGE_CURVE('',#29495,#29494,#24720,.T.) ;
#34694=EDGE_CURVE('',#29495,#29496,#24721,.T.) ;
#34695=EDGE_CURVE('',#29496,#29496,#24722,.T.) ;
#34696=EDGE_CURVE('',#29497,#29497,#24723,.T.) ;
#34697=EDGE_CURVE('',#29497,#29498,#24724,.T.) ;
#34698=EDGE_CURVE('',#29499,#29498,#24725,.T.) ;
#34699=EDGE_CURVE('',#29498,#29499,#24726,.T.) ;
#34700=EDGE_CURVE('',#29500,#29501,#24727,.T.) ;
#34701=EDGE_CURVE('',#29501,#29500,#24728,.T.) ;
#34702=EDGE_CURVE('',#29501,#29502,#24729,.T.) ;
#34703=EDGE_CURVE('',#29503,#29502,#24730,.T.) ;
#34704=EDGE_CURVE('',#29502,#29503,#24731,.T.) ;
#34705=EDGE_CURVE('',#29504,#29504,#24732,.T.) ;
#34706=EDGE_CURVE('',#29504,#29505,#24733,.T.) ;
#34707=EDGE_CURVE('',#29505,#29505,#24734,.T.) ;
#34708=EDGE_CURVE('',#29506,#29507,#24735,.T.) ;
#34709=EDGE_CURVE('',#29507,#29506,#24736,.T.) ;
#34710=EDGE_CURVE('',#29507,#29508,#24737,.T.) ;
#34711=EDGE_CURVE('',#29509,#29508,#24738,.T.) ;
#34712=EDGE_CURVE('',#29508,#29509,#24739,.T.) ;
#34713=EDGE_CURVE('',#29510,#29510,#24740,.T.) ;
#34714=EDGE_CURVE('',#29510,#29511,#24741,.T.) ;
#34715=EDGE_CURVE('',#29511,#29511,#24742,.T.) ;
#34716=EDGE_CURVE('',#29506,#29512,#7896,.T.) ;
#34717=EDGE_CURVE('',#29512,#29512,#24743,.T.) ;
#34718=EDGE_CURVE('',#29511,#29509,#7897,.T.) ;
#34719=EDGE_CURVE('',#29500,#29513,#7898,.T.) ;
#34720=EDGE_CURVE('',#29513,#29513,#24744,.T.) ;
#34721=EDGE_CURVE('',#29505,#29503,#7899,.T.) ;
#34722=EDGE_CURVE('',#29494,#29499,#7900,.T.) ;
#34723=EDGE_CURVE('',#29514,#29515,#7901,.T.) ;
#34724=EDGE_CURVE('',#29515,#29516,#7902,.T.) ;
#34725=EDGE_CURVE('',#29516,#29517,#7903,.T.) ;
#34726=EDGE_CURVE('',#29517,#29518,#7904,.T.) ;
#34727=EDGE_CURVE('',#29519,#29518,#7905,.T.) ;
#34728=EDGE_CURVE('',#29514,#29519,#7906,.T.) ;
#34729=EDGE_CURVE('',#29520,#29521,#24745,.T.) ;
#34730=EDGE_CURVE('',#29520,#29522,#7907,.T.) ;
#34731=EDGE_CURVE('',#29523,#29522,#24746,.T.) ;
#34732=EDGE_CURVE('',#29523,#29524,#7908,.T.) ;
#34733=EDGE_CURVE('',#29525,#29524,#24747,.T.) ;
#34734=EDGE_CURVE('',#29525,#29526,#7909,.T.) ;
#34735=EDGE_CURVE('',#29527,#29526,#24748,.T.) ;
#34736=EDGE_CURVE('',#29527,#29521,#7910,.T.) ;
#34737=EDGE_CURVE('',#29528,#29529,#7911,.T.) ;
#34738=EDGE_CURVE('',#29529,#29530,#7912,.T.) ;
#34739=EDGE_CURVE('',#29531,#29530,#7913,.T.) ;
#34740=EDGE_CURVE('',#29532,#29531,#7914,.T.) ;
#34741=EDGE_CURVE('',#29532,#29533,#7915,.T.) ;
#34742=EDGE_CURVE('',#29533,#29528,#7916,.T.) ;
#34743=EDGE_CURVE('',#29534,#29535,#24749,.T.) ;
#34744=EDGE_CURVE('',#29534,#29536,#7917,.T.) ;
#34745=EDGE_CURVE('',#29537,#29536,#24750,.T.) ;
#34746=EDGE_CURVE('',#29537,#29538,#7918,.T.) ;
#34747=EDGE_CURVE('',#29539,#29538,#24751,.T.) ;
#34748=EDGE_CURVE('',#29539,#29540,#7919,.T.) ;
#34749=EDGE_CURVE('',#29541,#29540,#24752,.T.) ;
#34750=EDGE_CURVE('',#29541,#29535,#7920,.T.) ;
#34751=EDGE_CURVE('',#29542,#29543,#24753,.T.) ;
#34752=EDGE_CURVE('',#29542,#29544,#7921,.T.) ;
#34753=EDGE_CURVE('',#29545,#29544,#7922,.T.) ;
#34754=EDGE_CURVE('',#29546,#29545,#7923,.T.) ;
#34755=EDGE_CURVE('',#29546,#29547,#7924,.T.) ;
#34756=EDGE_CURVE('',#29547,#29548,#7925,.T.) ;
#34757=EDGE_CURVE('',#29548,#29549,#7926,.T.) ;
#34758=EDGE_CURVE('',#29550,#29549,#24754,.T.) ;
#34759=EDGE_CURVE('',#29550,#29551,#7927,.T.) ;
#34760=EDGE_CURVE('',#29551,#29552,#7928,.T.) ;
#34761=EDGE_CURVE('',#29552,#29543,#7929,.T.) ;
#34762=EDGE_CURVE('',#29553,#29554,#24755,.T.) ;
#34763=EDGE_CURVE('',#29553,#29555,#7930,.T.) ;
#34764=EDGE_CURVE('',#29556,#29555,#24756,.T.) ;
#34765=EDGE_CURVE('',#29556,#29557,#7931,.T.) ;
#34766=EDGE_CURVE('',#29558,#29557,#24757,.T.) ;
#34767=EDGE_CURVE('',#29558,#29559,#7932,.T.) ;
#34768=EDGE_CURVE('',#29560,#29559,#24758,.T.) ;
#34769=EDGE_CURVE('',#29560,#29554,#7933,.T.) ;
#34770=EDGE_CURVE('',#29561,#29562,#24759,.T.) ;
#34771=EDGE_CURVE('',#29561,#29563,#7934,.T.) ;
#34772=EDGE_CURVE('',#29564,#29563,#24760,.T.) ;
#34773=EDGE_CURVE('',#29564,#29565,#7935,.T.) ;
#34774=EDGE_CURVE('',#29566,#29565,#24761,.T.) ;
#34775=EDGE_CURVE('',#29566,#29567,#7936,.T.) ;
#34776=EDGE_CURVE('',#29568,#29567,#24762,.T.) ;
#34777=EDGE_CURVE('',#29568,#29562,#7937,.T.) ;
#34778=EDGE_CURVE('',#29569,#29570,#24763,.T.) ;
#34779=EDGE_CURVE('',#29569,#29571,#7938,.T.) ;
#34780=EDGE_CURVE('',#29572,#29571,#24764,.T.) ;
#34781=EDGE_CURVE('',#29572,#29573,#7939,.T.) ;
#34782=EDGE_CURVE('',#29574,#29573,#24765,.T.) ;
#34783=EDGE_CURVE('',#29574,#29575,#7940,.T.) ;
#34784=EDGE_CURVE('',#29576,#29575,#24766,.T.) ;
#34785=EDGE_CURVE('',#29576,#29570,#7941,.T.) ;
#34786=EDGE_CURVE('',#29577,#29578,#24767,.T.) ;
#34787=EDGE_CURVE('',#29577,#29579,#7942,.T.) ;
#34788=EDGE_CURVE('',#29580,#29579,#24768,.T.) ;
#34789=EDGE_CURVE('',#29580,#29581,#7943,.T.) ;
#34790=EDGE_CURVE('',#29582,#29581,#24769,.T.) ;
#34791=EDGE_CURVE('',#29582,#29583,#7944,.T.) ;
#34792=EDGE_CURVE('',#29584,#29583,#24770,.T.) ;
#34793=EDGE_CURVE('',#29584,#29578,#7945,.T.) ;
#34794=EDGE_CURVE('',#29585,#29586,#7946,.T.) ;
#34795=EDGE_CURVE('',#29586,#29587,#7947,.T.) ;
#34796=EDGE_CURVE('',#29588,#29587,#24771,.T.) ;
#34797=EDGE_CURVE('',#29588,#29589,#7948,.T.) ;
#34798=EDGE_CURVE('',#29589,#29590,#7949,.T.) ;
#34799=EDGE_CURVE('',#29590,#29591,#7950,.T.) ;
#34800=EDGE_CURVE('',#29592,#29591,#24772,.T.) ;
#34801=EDGE_CURVE('',#29592,#29593,#7951,.T.) ;
#34802=EDGE_CURVE('',#29593,#29594,#7952,.T.) ;
#34803=EDGE_CURVE('',#29594,#29595,#7953,.T.) ;
#34804=EDGE_CURVE('',#29595,#29585,#7954,.T.) ;
#34805=EDGE_CURVE('',#29596,#29597,#24773,.T.) ;
#34806=EDGE_CURVE('',#29596,#29598,#7955,.T.) ;
#34807=EDGE_CURVE('',#29599,#29598,#24774,.T.) ;
#34808=EDGE_CURVE('',#29599,#29600,#7956,.T.) ;
#34809=EDGE_CURVE('',#29601,#29600,#24775,.T.) ;
#34810=EDGE_CURVE('',#29601,#29602,#7957,.T.) ;
#34811=EDGE_CURVE('',#29603,#29602,#24776,.T.) ;
#34812=EDGE_CURVE('',#29603,#29597,#7958,.T.) ;
#34813=EDGE_CURVE('',#29604,#29605,#24777,.T.) ;
#34814=EDGE_CURVE('',#29604,#29606,#7959,.T.) ;
#34815=EDGE_CURVE('',#29607,#29606,#24778,.T.) ;
#34816=EDGE_CURVE('',#29607,#29608,#7960,.T.) ;
#34817=EDGE_CURVE('',#29609,#29608,#24779,.T.) ;
#34818=EDGE_CURVE('',#29609,#29610,#7961,.T.) ;
#34819=EDGE_CURVE('',#29611,#29610,#24780,.T.) ;
#34820=EDGE_CURVE('',#29611,#29605,#7962,.T.) ;
#34821=EDGE_CURVE('',#29612,#29613,#24781,.T.) ;
#34822=EDGE_CURVE('',#29612,#29614,#7963,.T.) ;
#34823=EDGE_CURVE('',#29615,#29614,#24782,.T.) ;
#34824=EDGE_CURVE('',#29615,#29616,#7964,.T.) ;
#34825=EDGE_CURVE('',#29617,#29616,#24783,.T.) ;
#34826=EDGE_CURVE('',#29617,#29618,#7965,.T.) ;
#34827=EDGE_CURVE('',#29619,#29618,#24784,.T.) ;
#34828=EDGE_CURVE('',#29619,#29613,#7966,.T.) ;
#34829=EDGE_CURVE('',#29620,#29621,#24785,.T.) ;
#34830=EDGE_CURVE('',#29620,#29622,#7967,.T.) ;
#34831=EDGE_CURVE('',#29623,#29622,#24786,.T.) ;
#34832=EDGE_CURVE('',#29623,#29624,#7968,.T.) ;
#34833=EDGE_CURVE('',#29625,#29624,#24787,.T.) ;
#34834=EDGE_CURVE('',#29625,#29626,#7969,.T.) ;
#34835=EDGE_CURVE('',#29627,#29626,#24788,.T.) ;
#34836=EDGE_CURVE('',#29627,#29621,#7970,.T.) ;
#34837=EDGE_CURVE('',#29628,#29629,#7971,.T.) ;
#34838=EDGE_CURVE('',#29629,#29630,#7972,.T.) ;
#34839=EDGE_CURVE('',#29631,#29630,#24789,.T.) ;
#34840=EDGE_CURVE('',#29631,#29632,#7973,.T.) ;
#34841=EDGE_CURVE('',#29632,#29633,#7974,.T.) ;
#34842=EDGE_CURVE('',#29633,#29634,#7975,.T.) ;
#34843=EDGE_CURVE('',#29635,#29634,#24790,.T.) ;
#34844=EDGE_CURVE('',#29635,#29636,#7976,.T.) ;
#34845=EDGE_CURVE('',#29636,#29637,#7977,.T.) ;
#34846=EDGE_CURVE('',#29637,#29638,#7978,.T.) ;
#34847=EDGE_CURVE('',#29638,#29628,#7979,.T.) ;
#34848=EDGE_CURVE('',#29639,#29640,#24791,.T.) ;
#34849=EDGE_CURVE('',#29639,#29641,#7980,.T.) ;
#34850=EDGE_CURVE('',#29642,#29641,#24792,.T.) ;
#34851=EDGE_CURVE('',#29642,#29643,#7981,.T.) ;
#34852=EDGE_CURVE('',#29644,#29643,#24793,.T.) ;
#34853=EDGE_CURVE('',#29644,#29645,#7982,.T.) ;
#34854=EDGE_CURVE('',#29646,#29645,#24794,.T.) ;
#34855=EDGE_CURVE('',#29646,#29640,#7983,.T.) ;
#34856=EDGE_CURVE('',#29647,#29648,#24795,.T.) ;
#34857=EDGE_CURVE('',#29647,#29649,#7984,.T.) ;
#34858=EDGE_CURVE('',#29650,#29649,#24796,.T.) ;
#34859=EDGE_CURVE('',#29650,#29651,#7985,.T.) ;
#34860=EDGE_CURVE('',#29652,#29651,#24797,.T.) ;
#34861=EDGE_CURVE('',#29652,#29653,#7986,.T.) ;
#34862=EDGE_CURVE('',#29654,#29653,#24798,.T.) ;
#34863=EDGE_CURVE('',#29654,#29648,#7987,.T.) ;
#34864=EDGE_CURVE('',#29655,#29656,#24799,.T.) ;
#34865=EDGE_CURVE('',#29655,#29657,#7988,.T.) ;
#34866=EDGE_CURVE('',#29658,#29657,#24800,.T.) ;
#34867=EDGE_CURVE('',#29658,#29659,#7989,.T.) ;
#34868=EDGE_CURVE('',#29660,#29659,#24801,.T.) ;
#34869=EDGE_CURVE('',#29660,#29661,#7990,.T.) ;
#34870=EDGE_CURVE('',#29662,#29661,#24802,.T.) ;
#34871=EDGE_CURVE('',#29662,#29656,#7991,.T.) ;
#34872=EDGE_CURVE('',#29663,#29664,#24803,.T.) ;
#34873=EDGE_CURVE('',#29663,#29665,#7992,.T.) ;
#34874=EDGE_CURVE('',#29666,#29665,#24804,.T.) ;
#34875=EDGE_CURVE('',#29666,#29667,#7993,.T.) ;
#34876=EDGE_CURVE('',#29668,#29667,#24805,.T.) ;
#34877=EDGE_CURVE('',#29668,#29669,#7994,.T.) ;
#34878=EDGE_CURVE('',#29670,#29669,#24806,.T.) ;
#34879=EDGE_CURVE('',#29670,#29664,#7995,.T.) ;
#34880=EDGE_CURVE('',#29671,#29672,#24807,.T.) ;
#34881=EDGE_CURVE('',#29671,#29673,#7996,.T.) ;
#34882=EDGE_CURVE('',#29674,#29673,#24808,.T.) ;
#34883=EDGE_CURVE('',#29674,#29675,#7997,.T.) ;
#34884=EDGE_CURVE('',#29676,#29675,#24809,.T.) ;
#34885=EDGE_CURVE('',#29676,#29677,#7998,.T.) ;
#34886=EDGE_CURVE('',#29678,#29677,#24810,.T.) ;
#34887=EDGE_CURVE('',#29678,#29672,#7999,.T.) ;
#34888=EDGE_CURVE('',#29679,#29680,#24811,.T.) ;
#34889=EDGE_CURVE('',#29679,#29681,#8000,.T.) ;
#34890=EDGE_CURVE('',#29682,#29681,#24812,.T.) ;
#34891=EDGE_CURVE('',#29682,#29683,#8001,.T.) ;
#34892=EDGE_CURVE('',#29684,#29683,#24813,.T.) ;
#34893=EDGE_CURVE('',#29684,#29685,#8002,.T.) ;
#34894=EDGE_CURVE('',#29686,#29685,#24814,.T.) ;
#34895=EDGE_CURVE('',#29686,#29680,#8003,.T.) ;
#34896=EDGE_CURVE('',#29687,#29688,#24815,.T.) ;
#34897=EDGE_CURVE('',#29687,#29689,#8004,.T.) ;
#34898=EDGE_CURVE('',#29690,#29689,#24816,.T.) ;
#34899=EDGE_CURVE('',#29690,#29691,#8005,.T.) ;
#34900=EDGE_CURVE('',#29692,#29691,#24817,.T.) ;
#34901=EDGE_CURVE('',#29692,#29693,#8006,.T.) ;
#34902=EDGE_CURVE('',#29694,#29693,#24818,.T.) ;
#34903=EDGE_CURVE('',#29694,#29688,#8007,.T.) ;
#34904=EDGE_CURVE('',#29695,#29696,#24819,.T.) ;
#34905=EDGE_CURVE('',#29695,#29697,#8008,.T.) ;
#34906=EDGE_CURVE('',#29698,#29697,#8009,.T.) ;
#34907=EDGE_CURVE('',#29699,#29698,#8010,.T.) ;
#34908=EDGE_CURVE('',#29699,#29700,#8011,.T.) ;
#34909=EDGE_CURVE('',#29700,#29701,#8012,.T.) ;
#34910=EDGE_CURVE('',#29701,#29702,#8013,.T.) ;
#34911=EDGE_CURVE('',#29703,#29702,#24820,.T.) ;
#34912=EDGE_CURVE('',#29703,#29704,#8014,.T.) ;
#34913=EDGE_CURVE('',#29704,#29705,#8015,.T.) ;
#34914=EDGE_CURVE('',#29705,#29696,#8016,.T.) ;
#34915=EDGE_CURVE('',#29706,#29707,#24821,.T.) ;
#34916=EDGE_CURVE('',#29706,#29708,#8017,.T.) ;
#34917=EDGE_CURVE('',#29709,#29708,#24822,.T.) ;
#34918=EDGE_CURVE('',#29709,#29710,#8018,.T.) ;
#34919=EDGE_CURVE('',#29711,#29710,#24823,.T.) ;
#34920=EDGE_CURVE('',#29711,#29712,#8019,.T.) ;
#34921=EDGE_CURVE('',#29713,#29712,#24824,.T.) ;
#34922=EDGE_CURVE('',#29713,#29707,#8020,.T.) ;
#34923=EDGE_CURVE('',#29714,#29715,#24825,.T.) ;
#34924=EDGE_CURVE('',#29714,#29716,#8021,.T.) ;
#34925=EDGE_CURVE('',#29717,#29716,#24826,.T.) ;
#34926=EDGE_CURVE('',#29717,#29718,#8022,.T.) ;
#34927=EDGE_CURVE('',#29719,#29718,#24827,.T.) ;
#34928=EDGE_CURVE('',#29719,#29720,#8023,.T.) ;
#34929=EDGE_CURVE('',#29721,#29720,#24828,.T.) ;
#34930=EDGE_CURVE('',#29721,#29715,#8024,.T.) ;
#34931=EDGE_CURVE('',#29722,#29723,#24829,.T.) ;
#34932=EDGE_CURVE('',#29722,#29724,#8025,.T.) ;
#34933=EDGE_CURVE('',#29725,#29724,#24830,.T.) ;
#34934=EDGE_CURVE('',#29725,#29726,#8026,.T.) ;
#34935=EDGE_CURVE('',#29727,#29726,#24831,.T.) ;
#34936=EDGE_CURVE('',#29727,#29728,#8027,.T.) ;
#34937=EDGE_CURVE('',#29729,#29728,#24832,.T.) ;
#34938=EDGE_CURVE('',#29729,#29723,#8028,.T.) ;
#34939=EDGE_CURVE('',#29730,#29731,#24833,.T.) ;
#34940=EDGE_CURVE('',#29730,#29732,#8029,.T.) ;
#34941=EDGE_CURVE('',#29733,#29732,#24834,.T.) ;
#34942=EDGE_CURVE('',#29733,#29734,#8030,.T.) ;
#34943=EDGE_CURVE('',#29735,#29734,#24835,.T.) ;
#34944=EDGE_CURVE('',#29735,#29736,#8031,.T.) ;
#34945=EDGE_CURVE('',#29737,#29736,#24836,.T.) ;
#34946=EDGE_CURVE('',#29737,#29731,#8032,.T.) ;
#34947=EDGE_CURVE('',#29738,#29739,#24837,.T.) ;
#34948=EDGE_CURVE('',#29738,#29740,#8033,.T.) ;
#34949=EDGE_CURVE('',#29741,#29740,#24838,.T.) ;
#34950=EDGE_CURVE('',#29741,#29742,#8034,.T.) ;
#34951=EDGE_CURVE('',#29743,#29742,#24839,.T.) ;
#34952=EDGE_CURVE('',#29743,#29744,#8035,.T.) ;
#34953=EDGE_CURVE('',#29745,#29744,#24840,.T.) ;
#34954=EDGE_CURVE('',#29745,#29739,#8036,.T.) ;
#34955=EDGE_CURVE('',#29746,#29747,#24841,.T.) ;
#34956=EDGE_CURVE('',#29746,#29748,#8037,.T.) ;
#34957=EDGE_CURVE('',#29749,#29748,#24842,.T.) ;
#34958=EDGE_CURVE('',#29749,#29750,#8038,.T.) ;
#34959=EDGE_CURVE('',#29751,#29750,#24843,.T.) ;
#34960=EDGE_CURVE('',#29751,#29752,#8039,.T.) ;
#34961=EDGE_CURVE('',#29753,#29752,#24844,.T.) ;
#34962=EDGE_CURVE('',#29753,#29747,#8040,.T.) ;
#34963=EDGE_CURVE('',#29754,#29755,#24845,.T.) ;
#34964=EDGE_CURVE('',#29754,#29756,#8041,.T.) ;
#34965=EDGE_CURVE('',#29757,#29756,#24846,.T.) ;
#34966=EDGE_CURVE('',#29757,#29758,#8042,.T.) ;
#34967=EDGE_CURVE('',#29759,#29758,#24847,.T.) ;
#34968=EDGE_CURVE('',#29759,#29760,#8043,.T.) ;
#34969=EDGE_CURVE('',#29761,#29760,#24848,.T.) ;
#34970=EDGE_CURVE('',#29761,#29755,#8044,.T.) ;
#34971=EDGE_CURVE('',#29762,#29763,#24849,.T.) ;
#34972=EDGE_CURVE('',#29762,#29764,#8045,.T.) ;
#34973=EDGE_CURVE('',#29765,#29764,#8046,.T.) ;
#34974=EDGE_CURVE('',#29765,#29766,#8047,.T.) ;
#34975=EDGE_CURVE('',#29766,#29767,#8048,.T.) ;
#34976=EDGE_CURVE('',#29767,#29768,#8049,.T.) ;
#34977=EDGE_CURVE('',#29769,#29768,#24850,.T.) ;
#34978=EDGE_CURVE('',#29769,#29770,#8050,.T.) ;
#34979=EDGE_CURVE('',#29770,#29771,#8051,.T.) ;
#34980=EDGE_CURVE('',#29771,#29763,#8052,.T.) ;
#34981=EDGE_CURVE('',#29772,#29773,#8053,.T.) ;
#34982=EDGE_CURVE('',#29773,#29774,#8054,.T.) ;
#34983=EDGE_CURVE('',#29775,#29774,#24851,.T.) ;
#34984=EDGE_CURVE('',#29775,#29776,#8055,.T.) ;
#34985=EDGE_CURVE('',#29776,#29777,#8056,.T.) ;
#34986=EDGE_CURVE('',#29777,#29778,#8057,.T.) ;
#34987=EDGE_CURVE('',#29779,#29778,#24852,.T.) ;
#34988=EDGE_CURVE('',#29779,#29780,#8058,.T.) ;
#34989=EDGE_CURVE('',#29781,#29780,#8059,.T.) ;
#34990=EDGE_CURVE('',#29772,#29781,#8060,.T.) ;
#34991=EDGE_CURVE('',#29782,#29783,#8061,.T.) ;
#34992=EDGE_CURVE('',#29783,#29784,#8062,.T.) ;
#34993=EDGE_CURVE('',#29784,#29785,#8063,.T.) ;
#34994=EDGE_CURVE('',#29785,#29782,#8064,.T.) ;
#34995=EDGE_CURVE('',#29786,#29787,#8065,.T.) ;
#34996=EDGE_CURVE('',#29787,#29788,#8066,.T.) ;
#34997=EDGE_CURVE('',#29788,#29789,#8067,.T.) ;
#34998=EDGE_CURVE('',#29789,#29786,#8068,.T.) ;
#34999=EDGE_CURVE('',#29790,#29791,#8069,.T.) ;
#35000=EDGE_CURVE('',#29791,#29792,#8070,.T.) ;
#35001=EDGE_CURVE('',#29792,#29793,#8071,.T.) ;
#35002=EDGE_CURVE('',#29793,#29790,#8072,.T.) ;
#35003=EDGE_CURVE('',#29794,#29795,#8073,.T.) ;
#35004=EDGE_CURVE('',#29795,#29796,#8074,.T.) ;
#35005=EDGE_CURVE('',#29796,#29797,#8075,.T.) ;
#35006=EDGE_CURVE('',#29797,#29794,#8076,.T.) ;
#35007=EDGE_CURVE('',#29798,#29799,#8077,.T.) ;
#35008=EDGE_CURVE('',#29799,#29800,#8078,.T.) ;
#35009=EDGE_CURVE('',#29800,#29801,#8079,.T.) ;
#35010=EDGE_CURVE('',#29801,#29798,#8080,.T.) ;
#35011=EDGE_CURVE('',#29788,#29802,#24853,.T.) ;
#35012=EDGE_CURVE('',#29803,#29802,#8081,.T.) ;
#35013=EDGE_CURVE('',#29803,#29789,#24854,.T.) ;
#35014=EDGE_CURVE('',#29698,#29772,#24855,.T.) ;
#35015=EDGE_CURVE('',#29772,#29765,#8082,.T.) ;
#35016=EDGE_CURVE('',#29628,#29765,#24856,.T.) ;
#35017=EDGE_CURVE('',#29628,#29698,#8083,.T.) ;
#35018=EDGE_CURVE('',#29764,#29629,#24857,.T.) ;
#35019=EDGE_CURVE('',#29697,#29773,#24858,.T.) ;
#35020=EDGE_CURVE('',#29804,#29805,#8084,.T.) ;
#35021=EDGE_CURVE('',#29805,#29806,#8085,.T.) ;
#35022=EDGE_CURVE('',#29806,#29807,#8086,.T.) ;
#35023=EDGE_CURVE('',#29807,#29804,#8087,.T.) ;
#35024=EDGE_CURVE('',#29808,#29809,#8088,.T.) ;
#35025=EDGE_CURVE('',#29809,#29810,#8089,.T.) ;
#35026=EDGE_CURVE('',#29810,#29811,#8090,.T.) ;
#35027=EDGE_CURVE('',#29811,#29808,#8091,.T.) ;
#35028=EDGE_CURVE('',#29812,#29813,#8092,.T.) ;
#35029=EDGE_CURVE('',#29813,#29814,#8093,.T.) ;
#35030=EDGE_CURVE('',#29814,#29815,#8094,.T.) ;
#35031=EDGE_CURVE('',#29815,#29812,#8095,.T.) ;
#35032=EDGE_CURVE('',#29816,#29817,#8096,.T.) ;
#35033=EDGE_CURVE('',#29817,#29818,#8097,.T.) ;
#35034=EDGE_CURVE('',#29818,#29819,#8098,.T.) ;
#35035=EDGE_CURVE('',#29819,#29816,#8099,.T.) ;
#35036=EDGE_CURVE('',#29820,#29821,#8100,.T.) ;
#35037=EDGE_CURVE('',#29821,#29822,#8101,.T.) ;
#35038=EDGE_CURVE('',#29822,#29823,#8102,.T.) ;
#35039=EDGE_CURVE('',#29823,#29820,#8103,.T.) ;
#35040=EDGE_CURVE('',#29824,#29825,#8104,.T.) ;
#35041=EDGE_CURVE('',#29825,#29826,#8105,.T.) ;
#35042=EDGE_CURVE('',#29826,#29827,#8106,.T.) ;
#35043=EDGE_CURVE('',#29827,#29824,#8107,.T.) ;
#35044=EDGE_CURVE('',#29802,#29828,#8108,.T.) ;
#35045=EDGE_CURVE('',#29828,#29829,#8109,.T.) ;
#35046=EDGE_CURVE('',#29829,#29803,#8110,.T.) ;
#35047=EDGE_CURVE('',#29638,#29699,#8111,.T.) ;
#35048=EDGE_CURVE('',#29830,#29831,#8112,.T.) ;
#35049=EDGE_CURVE('',#29831,#29832,#8113,.T.) ;
#35050=EDGE_CURVE('',#29832,#29833,#8114,.T.) ;
#35051=EDGE_CURVE('',#29833,#29830,#8115,.T.) ;
#35052=EDGE_CURVE('',#29834,#29835,#8116,.T.) ;
#35053=EDGE_CURVE('',#29835,#29836,#8117,.T.) ;
#35054=EDGE_CURVE('',#29836,#29837,#8118,.T.) ;
#35055=EDGE_CURVE('',#29837,#29834,#8119,.T.) ;
#35056=EDGE_CURVE('',#29838,#29839,#8120,.T.) ;
#35057=EDGE_CURVE('',#29839,#29840,#8121,.T.) ;
#35058=EDGE_CURVE('',#29840,#29841,#8122,.T.) ;
#35059=EDGE_CURVE('',#29841,#29838,#8123,.T.) ;
#35060=EDGE_CURVE('',#29530,#29515,#8124,.T.) ;
#35061=EDGE_CURVE('',#29531,#29514,#8125,.T.) ;
#35062=EDGE_CURVE('',#29518,#29533,#8126,.T.) ;
#35063=EDGE_CURVE('',#29532,#29519,#8127,.T.) ;
#35064=EDGE_CURVE('',#29532,#29781,#24859,.T.) ;
#35065=EDGE_CURVE('',#29781,#29766,#8128,.T.) ;
#35066=EDGE_CURVE('',#29519,#29766,#24860,.T.) ;
#35067=EDGE_CURVE('',#29772,#29531,#24861,.T.) ;
#35068=EDGE_CURVE('',#29765,#29514,#24862,.T.) ;
#35069=EDGE_CURVE('',#29842,#29843,#8129,.T.) ;
#35070=EDGE_CURVE('',#29842,#29783,#24863,.T.) ;
#35071=EDGE_CURVE('',#29782,#29843,#24864,.T.) ;
#35072=EDGE_CURVE('',#29781,#29585,#24865,.T.) ;
#35073=EDGE_CURVE('',#29585,#29545,#8130,.T.) ;
#35074=EDGE_CURVE('',#29766,#29545,#24866,.T.) ;
#35075=EDGE_CURVE('',#29544,#29767,#24867,.T.) ;
#35076=EDGE_CURVE('',#29780,#29586,#24868,.T.) ;
#35077=EDGE_CURVE('',#29844,#29845,#8131,.T.) ;
#35078=EDGE_CURVE('',#29845,#29846,#8132,.T.) ;
#35079=EDGE_CURVE('',#29846,#29847,#8133,.T.) ;
#35080=EDGE_CURVE('',#29847,#29844,#8134,.T.) ;
#35081=EDGE_CURVE('',#29848,#29849,#8135,.T.) ;
#35082=EDGE_CURVE('',#29849,#29850,#8136,.T.) ;
#35083=EDGE_CURVE('',#29850,#29851,#8137,.T.) ;
#35084=EDGE_CURVE('',#29851,#29848,#8138,.T.) ;
#35085=EDGE_CURVE('',#29852,#29853,#8139,.T.) ;
#35086=EDGE_CURVE('',#29853,#29854,#8140,.T.) ;
#35087=EDGE_CURVE('',#29854,#29855,#8141,.T.) ;
#35088=EDGE_CURVE('',#29855,#29852,#8142,.T.) ;
#35089=EDGE_CURVE('',#29856,#29857,#8143,.T.) ;
#35090=EDGE_CURVE('',#29857,#29858,#8144,.T.) ;
#35091=EDGE_CURVE('',#29858,#29859,#8145,.T.) ;
#35092=EDGE_CURVE('',#29859,#29856,#8146,.T.) ;
#35093=EDGE_CURVE('',#29860,#29861,#8147,.T.) ;
#35094=EDGE_CURVE('',#29861,#29862,#8148,.T.) ;
#35095=EDGE_CURVE('',#29862,#29863,#8149,.T.) ;
#35096=EDGE_CURVE('',#29863,#29860,#8150,.T.) ;
#35097=EDGE_CURVE('',#29864,#29865,#8151,.T.) ;
#35098=EDGE_CURVE('',#29865,#29866,#8152,.T.) ;
#35099=EDGE_CURVE('',#29866,#29867,#8153,.T.) ;
#35100=EDGE_CURVE('',#29867,#29864,#8154,.T.) ;
#35101=EDGE_CURVE('',#29595,#29546,#8155,.T.) ;
#35102=EDGE_CURVE('',#29868,#29869,#8156,.T.) ;
#35103=EDGE_CURVE('',#29869,#29842,#8157,.T.) ;
#35104=EDGE_CURVE('',#29843,#29868,#8158,.T.) ;
#35105=EDGE_CURVE('',#29870,#29871,#8159,.T.) ;
#35106=EDGE_CURVE('',#29871,#29872,#8160,.T.) ;
#35107=EDGE_CURVE('',#29872,#29873,#8161,.T.) ;
#35108=EDGE_CURVE('',#29873,#29870,#8162,.T.) ;
#35109=EDGE_CURVE('',#29874,#29875,#8163,.T.) ;
#35110=EDGE_CURVE('',#29875,#29876,#8164,.T.) ;
#35111=EDGE_CURVE('',#29876,#29877,#8165,.T.) ;
#35112=EDGE_CURVE('',#29877,#29874,#8166,.T.) ;
#35113=EDGE_CURVE('',#29878,#29879,#8167,.T.) ;
#35114=EDGE_CURVE('',#29879,#29880,#8168,.T.) ;
#35115=EDGE_CURVE('',#29880,#29881,#8169,.T.) ;
#35116=EDGE_CURVE('',#29881,#29878,#8170,.T.) ;
#35117=EDGE_CURVE('',#29882,#29883,#8171,.T.) ;
#35118=EDGE_CURVE('',#29883,#29884,#8172,.T.) ;
#35119=EDGE_CURVE('',#29884,#29885,#8173,.T.) ;
#35120=EDGE_CURVE('',#29885,#29882,#8174,.T.) ;
#35121=EDGE_CURVE('',#29886,#29887,#8175,.T.) ;
#35122=EDGE_CURVE('',#29887,#29888,#8176,.T.) ;
#35123=EDGE_CURVE('',#29888,#29889,#8177,.T.) ;
#35124=EDGE_CURVE('',#29889,#29886,#8178,.T.) ;
#35125=EDGE_CURVE('',#29890,#29891,#8179,.T.) ;
#35126=EDGE_CURVE('',#29891,#29892,#8180,.T.) ;
#35127=EDGE_CURVE('',#29892,#29893,#8181,.T.) ;
#35128=EDGE_CURVE('',#29893,#29890,#8182,.T.) ;
#35129=EDGE_CURVE('',#29894,#29895,#8183,.T.) ;
#35130=EDGE_CURVE('',#29895,#29896,#8184,.T.) ;
#35131=EDGE_CURVE('',#29896,#29897,#8185,.T.) ;
#35132=EDGE_CURVE('',#29897,#29894,#8186,.T.) ;
#35133=EDGE_CURVE('',#29898,#29899,#8187,.T.) ;
#35134=EDGE_CURVE('',#29899,#29900,#8188,.T.) ;
#35135=EDGE_CURVE('',#29900,#29901,#8189,.T.) ;
#35136=EDGE_CURVE('',#29901,#29898,#8190,.T.) ;
#35137=EDGE_CURVE('',#29902,#29903,#8191,.T.) ;
#35138=EDGE_CURVE('',#29903,#29904,#8192,.T.) ;
#35139=EDGE_CURVE('',#29904,#29905,#8193,.T.) ;
#35140=EDGE_CURVE('',#29905,#29902,#8194,.T.) ;
#35141=EDGE_CURVE('',#29906,#29907,#8195,.T.) ;
#35142=EDGE_CURVE('',#29907,#29908,#8196,.T.) ;
#35143=EDGE_CURVE('',#29908,#29909,#8197,.T.) ;
#35144=EDGE_CURVE('',#29909,#29906,#8198,.T.) ;
#35145=EDGE_CURVE('',#29910,#29911,#8199,.T.) ;
#35146=EDGE_CURVE('',#29911,#29912,#8200,.T.) ;
#35147=EDGE_CURVE('',#29912,#29913,#8201,.T.) ;
#35148=EDGE_CURVE('',#29913,#29910,#8202,.T.) ;
#35149=EDGE_CURVE('',#29914,#29915,#8203,.T.) ;
#35150=EDGE_CURVE('',#29915,#29916,#8204,.T.) ;
#35151=EDGE_CURVE('',#29916,#29917,#8205,.T.) ;
#35152=EDGE_CURVE('',#29917,#29914,#8206,.T.) ;
#35153=EDGE_CURVE('',#29918,#29919,#8207,.T.) ;
#35154=EDGE_CURVE('',#29919,#29920,#8208,.T.) ;
#35155=EDGE_CURVE('',#29920,#29921,#8209,.T.) ;
#35156=EDGE_CURVE('',#29921,#29918,#8210,.T.) ;
#35157=EDGE_CURVE('',#29922,#29923,#8211,.T.) ;
#35158=EDGE_CURVE('',#29923,#29924,#8212,.T.) ;
#35159=EDGE_CURVE('',#29924,#29925,#8213,.T.) ;
#35160=EDGE_CURVE('',#29925,#29922,#8214,.T.) ;
#35161=EDGE_CURVE('',#29926,#29927,#8215,.T.) ;
#35162=EDGE_CURVE('',#29927,#29928,#8216,.T.) ;
#35163=EDGE_CURVE('',#29928,#29929,#8217,.T.) ;
#35164=EDGE_CURVE('',#29929,#29926,#8218,.T.) ;
#35165=EDGE_CURVE('',#29930,#29931,#8219,.T.) ;
#35166=EDGE_CURVE('',#29931,#29932,#8220,.T.) ;
#35167=EDGE_CURVE('',#29932,#29933,#8221,.T.) ;
#35168=EDGE_CURVE('',#29933,#29930,#8222,.T.) ;
#35169=EDGE_CURVE('',#29934,#29935,#8223,.T.) ;
#35170=EDGE_CURVE('',#29935,#29936,#8224,.T.) ;
#35171=EDGE_CURVE('',#29936,#29937,#8225,.T.) ;
#35172=EDGE_CURVE('',#29937,#29934,#8226,.T.) ;
#35173=EDGE_CURVE('',#29938,#29939,#8227,.T.) ;
#35174=EDGE_CURVE('',#29939,#29940,#8228,.T.) ;
#35175=EDGE_CURVE('',#29940,#29941,#8229,.T.) ;
#35176=EDGE_CURVE('',#29941,#29938,#8230,.T.) ;
#35177=EDGE_CURVE('',#29942,#29943,#8231,.T.) ;
#35178=EDGE_CURVE('',#29943,#29944,#8232,.T.) ;
#35179=EDGE_CURVE('',#29944,#29945,#8233,.T.) ;
#35180=EDGE_CURVE('',#29945,#29942,#8234,.T.) ;
#35181=EDGE_CURVE('',#29946,#29947,#8235,.T.) ;
#35182=EDGE_CURVE('',#29947,#29948,#8236,.T.) ;
#35183=EDGE_CURVE('',#29948,#29949,#8237,.T.) ;
#35184=EDGE_CURVE('',#29949,#29946,#8238,.T.) ;
#35185=EDGE_CURVE('',#29950,#29951,#8239,.T.) ;
#35186=EDGE_CURVE('',#29951,#29952,#8240,.T.) ;
#35187=EDGE_CURVE('',#29952,#29953,#8241,.T.) ;
#35188=EDGE_CURVE('',#29953,#29950,#8242,.T.) ;
#35189=EDGE_CURVE('',#29954,#29955,#8243,.T.) ;
#35190=EDGE_CURVE('',#29955,#29956,#8244,.T.) ;
#35191=EDGE_CURVE('',#29956,#29957,#8245,.T.) ;
#35192=EDGE_CURVE('',#29957,#29954,#8246,.T.) ;
#35193=EDGE_CURVE('',#29958,#29959,#8247,.T.) ;
#35194=EDGE_CURVE('',#29959,#29960,#8248,.T.) ;
#35195=EDGE_CURVE('',#29960,#29961,#8249,.T.) ;
#35196=EDGE_CURVE('',#29961,#29958,#8250,.T.) ;
#35197=EDGE_CURVE('',#29962,#29963,#8251,.T.) ;
#35198=EDGE_CURVE('',#29963,#29964,#8252,.T.) ;
#35199=EDGE_CURVE('',#29964,#29965,#8253,.T.) ;
#35200=EDGE_CURVE('',#29965,#29962,#8254,.T.) ;
#35201=EDGE_CURVE('',#29966,#29967,#8255,.T.) ;
#35202=EDGE_CURVE('',#29967,#29968,#8256,.T.) ;
#35203=EDGE_CURVE('',#29968,#29969,#8257,.T.) ;
#35204=EDGE_CURVE('',#29969,#29966,#8258,.T.) ;
#35205=EDGE_CURVE('',#29970,#29971,#8259,.T.) ;
#35206=EDGE_CURVE('',#29971,#29972,#8260,.T.) ;
#35207=EDGE_CURVE('',#29972,#29973,#8261,.T.) ;
#35208=EDGE_CURVE('',#29973,#29970,#8262,.T.) ;
#35209=EDGE_CURVE('',#29974,#29975,#8263,.T.) ;
#35210=EDGE_CURVE('',#29975,#29976,#8264,.T.) ;
#35211=EDGE_CURVE('',#29976,#29977,#8265,.T.) ;
#35212=EDGE_CURVE('',#29977,#29974,#8266,.T.) ;
#35213=EDGE_CURVE('',#29978,#29979,#8267,.T.) ;
#35214=EDGE_CURVE('',#29979,#29980,#8268,.T.) ;
#35215=EDGE_CURVE('',#29980,#29981,#8269,.T.) ;
#35216=EDGE_CURVE('',#29981,#29978,#8270,.T.) ;
#35217=EDGE_CURVE('',#29982,#29983,#8271,.T.) ;
#35218=EDGE_CURVE('',#29983,#29984,#8272,.T.) ;
#35219=EDGE_CURVE('',#29984,#29985,#8273,.T.) ;
#35220=EDGE_CURVE('',#29985,#29982,#8274,.T.) ;
#35221=EDGE_CURVE('',#29986,#29987,#8275,.T.) ;
#35222=EDGE_CURVE('',#29987,#29988,#8276,.T.) ;
#35223=EDGE_CURVE('',#29988,#29989,#8277,.T.) ;
#35224=EDGE_CURVE('',#29989,#29986,#8278,.T.) ;
#35225=EDGE_CURVE('',#29990,#29991,#8279,.T.) ;
#35226=EDGE_CURVE('',#29991,#29992,#8280,.T.) ;
#35227=EDGE_CURVE('',#29992,#29993,#8281,.T.) ;
#35228=EDGE_CURVE('',#29993,#29990,#8282,.T.) ;
#35229=EDGE_CURVE('',#29994,#29995,#8283,.T.) ;
#35230=EDGE_CURVE('',#29995,#29996,#8284,.T.) ;
#35231=EDGE_CURVE('',#29996,#29997,#8285,.T.) ;
#35232=EDGE_CURVE('',#29997,#29994,#8286,.T.) ;
#35233=EDGE_CURVE('',#29998,#29999,#8287,.T.) ;
#35234=EDGE_CURVE('',#29999,#30000,#8288,.T.) ;
#35235=EDGE_CURVE('',#30000,#30001,#8289,.T.) ;
#35236=EDGE_CURVE('',#30001,#29998,#8290,.T.) ;
#35237=EDGE_CURVE('',#30002,#30003,#8291,.T.) ;
#35238=EDGE_CURVE('',#30003,#30004,#8292,.T.) ;
#35239=EDGE_CURVE('',#30004,#30005,#8293,.T.) ;
#35240=EDGE_CURVE('',#30005,#30002,#8294,.T.) ;
#35241=EDGE_CURVE('',#30006,#30007,#8295,.T.) ;
#35242=EDGE_CURVE('',#30007,#30008,#8296,.T.) ;
#35243=EDGE_CURVE('',#30008,#30009,#8297,.T.) ;
#35244=EDGE_CURVE('',#30009,#30006,#8298,.T.) ;
#35245=EDGE_CURVE('',#30010,#30011,#8299,.T.) ;
#35246=EDGE_CURVE('',#30011,#30012,#8300,.T.) ;
#35247=EDGE_CURVE('',#30012,#30013,#8301,.T.) ;
#35248=EDGE_CURVE('',#30013,#30010,#8302,.T.) ;
#35249=EDGE_CURVE('',#30014,#30015,#8303,.T.) ;
#35250=EDGE_CURVE('',#30015,#30016,#8304,.T.) ;
#35251=EDGE_CURVE('',#30016,#30017,#8305,.T.) ;
#35252=EDGE_CURVE('',#30017,#30014,#8306,.T.) ;
#35253=EDGE_CURVE('',#30018,#30019,#8307,.T.) ;
#35254=EDGE_CURVE('',#30019,#30020,#8308,.T.) ;
#35255=EDGE_CURVE('',#30020,#30021,#8309,.T.) ;
#35256=EDGE_CURVE('',#30021,#30018,#8310,.T.) ;
#35257=EDGE_CURVE('',#30022,#30023,#8311,.T.) ;
#35258=EDGE_CURVE('',#30023,#30024,#8312,.T.) ;
#35259=EDGE_CURVE('',#30024,#30025,#8313,.T.) ;
#35260=EDGE_CURVE('',#30025,#30022,#8314,.T.) ;
#35261=EDGE_CURVE('',#30026,#30027,#8315,.T.) ;
#35262=EDGE_CURVE('',#30027,#30028,#8316,.T.) ;
#35263=EDGE_CURVE('',#30028,#30029,#8317,.T.) ;
#35264=EDGE_CURVE('',#30029,#30026,#8318,.T.) ;
#35265=EDGE_CURVE('',#30030,#30031,#8319,.T.) ;
#35266=EDGE_CURVE('',#30031,#30032,#8320,.T.) ;
#35267=EDGE_CURVE('',#30032,#30033,#8321,.T.) ;
#35268=EDGE_CURVE('',#30033,#30030,#8322,.T.) ;
#35269=EDGE_CURVE('',#30034,#30035,#8323,.T.) ;
#35270=EDGE_CURVE('',#30035,#30036,#8324,.T.) ;
#35271=EDGE_CURVE('',#30036,#30037,#8325,.T.) ;
#35272=EDGE_CURVE('',#30037,#30034,#8326,.T.) ;
#35273=EDGE_CURVE('',#30038,#30039,#8327,.T.) ;
#35274=EDGE_CURVE('',#30039,#30040,#8328,.T.) ;
#35275=EDGE_CURVE('',#30040,#30041,#8329,.T.) ;
#35276=EDGE_CURVE('',#30041,#30038,#8330,.T.) ;
#35277=EDGE_CURVE('',#30042,#30043,#8331,.T.) ;
#35278=EDGE_CURVE('',#30043,#30044,#8332,.T.) ;
#35279=EDGE_CURVE('',#30044,#30045,#8333,.T.) ;
#35280=EDGE_CURVE('',#30045,#30042,#8334,.T.) ;
#35281=EDGE_CURVE('',#30046,#30047,#8335,.T.) ;
#35282=EDGE_CURVE('',#30047,#30048,#8336,.T.) ;
#35283=EDGE_CURVE('',#30048,#30049,#8337,.T.) ;
#35284=EDGE_CURVE('',#30049,#30046,#8338,.T.) ;
#35285=EDGE_CURVE('',#30050,#30051,#8339,.T.) ;
#35286=EDGE_CURVE('',#30051,#30052,#8340,.T.) ;
#35287=EDGE_CURVE('',#30052,#30053,#8341,.T.) ;
#35288=EDGE_CURVE('',#30053,#30050,#8342,.T.) ;
#35289=EDGE_CURVE('',#30054,#30055,#8343,.T.) ;
#35290=EDGE_CURVE('',#30055,#30056,#8344,.T.) ;
#35291=EDGE_CURVE('',#30056,#30057,#8345,.T.) ;
#35292=EDGE_CURVE('',#30057,#30054,#8346,.T.) ;
#35293=EDGE_CURVE('',#30058,#30059,#8347,.T.) ;
#35294=EDGE_CURVE('',#30059,#30060,#8348,.T.) ;
#35295=EDGE_CURVE('',#30060,#30061,#8349,.T.) ;
#35296=EDGE_CURVE('',#30061,#30058,#8350,.T.) ;
#35297=EDGE_CURVE('',#29547,#29865,#24869,.T.) ;
#35298=EDGE_CURVE('',#29866,#29546,#4840,.T.) ;
#35299=EDGE_CURVE('',#29867,#29595,#4841,.T.) ;
#35300=EDGE_CURVE('',#29547,#29863,#24870,.T.) ;
#35301=EDGE_CURVE('',#29863,#29865,#24871,.T.) ;
#35302=EDGE_CURVE('',#29864,#29594,#24872,.T.) ;
#35303=EDGE_CURVE('',#29860,#29864,#24873,.T.) ;
#35304=EDGE_CURVE('',#29548,#29862,#24874,.T.) ;
#35305=EDGE_CURVE('',#29860,#29594,#24875,.T.) ;
#35306=EDGE_CURVE('',#29548,#29859,#24876,.T.) ;
#35307=EDGE_CURVE('',#29859,#29862,#24877,.T.) ;
#35308=EDGE_CURVE('',#29861,#29593,#24878,.T.) ;
#35309=EDGE_CURVE('',#29856,#29861,#24879,.T.) ;
#35310=EDGE_CURVE('',#29549,#29858,#24880,.T.) ;
#35311=EDGE_CURVE('',#29856,#29593,#24881,.T.) ;
#35312=EDGE_CURVE('',#29855,#29858,#24882,.T.) ;
#35313=EDGE_CURVE('',#29550,#29855,#24883,.T.) ;
#35314=EDGE_CURVE('',#29857,#29592,#24884,.T.) ;
#35315=EDGE_CURVE('',#29852,#29857,#24885,.T.) ;
#35316=EDGE_CURVE('',#29551,#29854,#24886,.T.) ;
#35317=EDGE_CURVE('',#29852,#29591,#24887,.T.) ;
#35318=EDGE_CURVE('',#29551,#29851,#24888,.T.) ;
#35319=EDGE_CURVE('',#29851,#29854,#24889,.T.) ;
#35320=EDGE_CURVE('',#29853,#29590,#24890,.T.) ;
#35321=EDGE_CURVE('',#29848,#29853,#24891,.T.) ;
#35322=EDGE_CURVE('',#29552,#29850,#24892,.T.) ;
#35323=EDGE_CURVE('',#29848,#29590,#24893,.T.) ;
#35324=EDGE_CURVE('',#29552,#29847,#24894,.T.) ;
#35325=EDGE_CURVE('',#29847,#29850,#24895,.T.) ;
#35326=EDGE_CURVE('',#29849,#29589,#24896,.T.) ;
#35327=EDGE_CURVE('',#29844,#29849,#24897,.T.) ;
#35328=EDGE_CURVE('',#29543,#29846,#24898,.T.) ;
#35329=EDGE_CURVE('',#29638,#29824,#4842,.T.) ;
#35330=EDGE_CURVE('',#29825,#29637,#24899,.T.) ;
#35331=EDGE_CURVE('',#29844,#29589,#24900,.T.) ;
#35332=EDGE_CURVE('',#29868,#29846,#24901,.T.) ;
#35333=EDGE_CURVE('',#29542,#29868,#24902,.T.) ;
#35334=EDGE_CURVE('',#29825,#29807,#24903,.T.) ;
#35335=EDGE_CURVE('',#29807,#29637,#24904,.T.) ;
#35336=EDGE_CURVE('',#29699,#29827,#4843,.T.) ;
#35337=EDGE_CURVE('',#29845,#29588,#24905,.T.) ;
#35338=EDGE_CURVE('',#29869,#29845,#24906,.T.) ;
#35339=EDGE_CURVE('',#29544,#29843,#24907,.T.) ;
#35340=EDGE_CURVE('',#29804,#29636,#24908,.T.) ;
#35341=EDGE_CURVE('',#29826,#29806,#24909,.T.) ;
#35342=EDGE_CURVE('',#29700,#29826,#24910,.T.) ;
#35343=EDGE_CURVE('',#29869,#29587,#24911,.T.) ;
#35344=EDGE_CURVE('',#29767,#29782,#24912,.T.) ;
#35345=EDGE_CURVE('',#29804,#29810,#24913,.T.) ;
#35346=EDGE_CURVE('',#29810,#29636,#24914,.T.) ;
#35347=EDGE_CURVE('',#29700,#29806,#24915,.T.) ;
#35348=EDGE_CURVE('',#29842,#29586,#24916,.T.) ;
#35349=EDGE_CURVE('',#29768,#29785,#24917,.T.) ;
#35350=EDGE_CURVE('',#29811,#29635,#24918,.T.) ;
#35351=EDGE_CURVE('',#29805,#29809,#24919,.T.) ;
#35352=EDGE_CURVE('',#29701,#29805,#24920,.T.) ;
#35353=EDGE_CURVE('',#29783,#29780,#24921,.T.) ;
#35354=EDGE_CURVE('',#29797,#29785,#24922,.T.) ;
#35355=EDGE_CURVE('',#29769,#29797,#24923,.T.) ;
#35356=EDGE_CURVE('',#29814,#29634,#24924,.T.) ;
#35357=EDGE_CURVE('',#29811,#29814,#24925,.T.) ;
#35358=EDGE_CURVE('',#29701,#29809,#24926,.T.) ;
#35359=EDGE_CURVE('',#29784,#29779,#24927,.T.) ;
#35360=EDGE_CURVE('',#29794,#29784,#24928,.T.) ;
#35361=EDGE_CURVE('',#29770,#29796,#24929,.T.) ;
#35362=EDGE_CURVE('',#29815,#29633,#24930,.T.) ;
#35363=EDGE_CURVE('',#29808,#29813,#24931,.T.) ;
#35364=EDGE_CURVE('',#29702,#29808,#24932,.T.) ;
#35365=EDGE_CURVE('',#29794,#29778,#24933,.T.) ;
#35366=EDGE_CURVE('',#29770,#29793,#24934,.T.) ;
#35367=EDGE_CURVE('',#29793,#29796,#24935,.T.) ;
#35368=EDGE_CURVE('',#29815,#29818,#24936,.T.) ;
#35369=EDGE_CURVE('',#29818,#29633,#24937,.T.) ;
#35370=EDGE_CURVE('',#29703,#29813,#24938,.T.) ;
#35371=EDGE_CURVE('',#29795,#29777,#24939,.T.) ;
#35372=EDGE_CURVE('',#29790,#29795,#24940,.T.) ;
#35373=EDGE_CURVE('',#29771,#29792,#24941,.T.) ;
#35374=EDGE_CURVE('',#29819,#29632,#24942,.T.) ;
#35375=EDGE_CURVE('',#29812,#29817,#24943,.T.) ;
#35376=EDGE_CURVE('',#29704,#29812,#24944,.T.) ;
#35377=EDGE_CURVE('',#29790,#29777,#24945,.T.) ;
#35378=EDGE_CURVE('',#29771,#29801,#24946,.T.) ;
#35379=EDGE_CURVE('',#29801,#29792,#24947,.T.) ;
#35380=EDGE_CURVE('',#29629,#29803,#24948,.T.) ;
#35381=EDGE_CURVE('',#29789,#29764,#24949,.T.) ;
#35382=EDGE_CURVE('',#29819,#29822,#24950,.T.) ;
#35383=EDGE_CURVE('',#29822,#29632,#24951,.T.) ;
#35384=EDGE_CURVE('',#29704,#29817,#24952,.T.) ;
#35385=EDGE_CURVE('',#29791,#29776,#24953,.T.) ;
#35386=EDGE_CURVE('',#29798,#29791,#24954,.T.) ;
#35387=EDGE_CURVE('',#29763,#29800,#24955,.T.) ;
#35388=EDGE_CURVE('',#29786,#29762,#24956,.T.) ;
#35389=EDGE_CURVE('',#29630,#29829,#24957,.T.) ;
#35390=EDGE_CURVE('',#29823,#29631,#24958,.T.) ;
#35391=EDGE_CURVE('',#29816,#29821,#24959,.T.) ;
#35392=EDGE_CURVE('',#29705,#29816,#24960,.T.) ;
#35393=EDGE_CURVE('',#29798,#29776,#24961,.T.) ;
#35394=EDGE_CURVE('',#29786,#29800,#24962,.T.) ;
#35395=EDGE_CURVE('',#29823,#29829,#24963,.T.) ;
#35396=EDGE_CURVE('',#29705,#29821,#24964,.T.) ;
#35397=EDGE_CURVE('',#29799,#29775,#24965,.T.) ;
#35398=EDGE_CURVE('',#29787,#29799,#24966,.T.) ;
#35399=EDGE_CURVE('',#29820,#29828,#24967,.T.) ;
#35400=EDGE_CURVE('',#29696,#29820,#24968,.T.) ;
#35401=EDGE_CURVE('',#29787,#29774,#24969,.T.) ;
#35402=EDGE_CURVE('',#29695,#29828,#24970,.T.) ;
#35403=EDGE_CURVE('',#29788,#29773,#24971,.T.) ;
#35404=EDGE_CURVE('',#29697,#29802,#24972,.T.) ;
#35405=EDGE_CURVE('',#29562,#30044,#24973,.T.) ;
#35406=EDGE_CURVE('',#30045,#29568,#24974,.T.) ;
#35407=EDGE_CURVE('',#30031,#30044,#24975,.T.) ;
#35408=EDGE_CURVE('',#29561,#30031,#24976,.T.) ;
#35409=EDGE_CURVE('',#30038,#29567,#24977,.T.) ;
#35410=EDGE_CURVE('',#30045,#30038,#24978,.T.) ;
#35411=EDGE_CURVE('',#30032,#30043,#24979,.T.) ;
#35412=EDGE_CURVE('',#29563,#30030,#24980,.T.) ;
#35413=EDGE_CURVE('',#29565,#30034,#24981,.T.) ;
#35414=EDGE_CURVE('',#30035,#29564,#24982,.T.) ;
#35415=EDGE_CURVE('',#30039,#29566,#24983,.T.) ;
#35416=EDGE_CURVE('',#30042,#30041,#24984,.T.) ;
#35417=EDGE_CURVE('',#29608,#30042,#24985,.T.) ;
#35418=EDGE_CURVE('',#30043,#29607,#24986,.T.) ;
#35419=EDGE_CURVE('',#30032,#29606,#24987,.T.) ;
#35420=EDGE_CURVE('',#30035,#30030,#24988,.T.) ;
#35421=EDGE_CURVE('',#30039,#30034,#24989,.T.) ;
#35422=EDGE_CURVE('',#29609,#30041,#24990,.T.) ;
#35423=EDGE_CURVE('',#30033,#29604,#24991,.T.) ;
#35424=EDGE_CURVE('',#30036,#30033,#24992,.T.) ;
#35425=EDGE_CURVE('',#30040,#30037,#24993,.T.) ;
#35426=EDGE_CURVE('',#29610,#30040,#24994,.T.) ;
#35427=EDGE_CURVE('',#30036,#29605,#24995,.T.) ;
#35428=EDGE_CURVE('',#29611,#30037,#24996,.T.) ;
#35429=EDGE_CURVE('',#29570,#30016,#24997,.T.) ;
#35430=EDGE_CURVE('',#30017,#29576,#24998,.T.) ;
#35431=EDGE_CURVE('',#30019,#30016,#24999,.T.) ;
#35432=EDGE_CURVE('',#29569,#30019,#25000,.T.) ;
#35433=EDGE_CURVE('',#30026,#29575,#25001,.T.) ;
#35434=EDGE_CURVE('',#30017,#30026,#25002,.T.) ;
#35435=EDGE_CURVE('',#30020,#30015,#25003,.T.) ;
#35436=EDGE_CURVE('',#29571,#30018,#25004,.T.) ;
#35437=EDGE_CURVE('',#29573,#30022,#25005,.T.) ;
#35438=EDGE_CURVE('',#30023,#29572,#25006,.T.) ;
#35439=EDGE_CURVE('',#30027,#29574,#25007,.T.) ;
#35440=EDGE_CURVE('',#30014,#30029,#25008,.T.) ;
#35441=EDGE_CURVE('',#29616,#30014,#25009,.T.) ;
#35442=EDGE_CURVE('',#30015,#29615,#25010,.T.) ;
#35443=EDGE_CURVE('',#30020,#29614,#25011,.T.) ;
#35444=EDGE_CURVE('',#30023,#30018,#25012,.T.) ;
#35445=EDGE_CURVE('',#30027,#30022,#25013,.T.) ;
#35446=EDGE_CURVE('',#29617,#30029,#25014,.T.) ;
#35447=EDGE_CURVE('',#30021,#29612,#25015,.T.) ;
#35448=EDGE_CURVE('',#30024,#30021,#25016,.T.) ;
#35449=EDGE_CURVE('',#30028,#30025,#25017,.T.) ;
#35450=EDGE_CURVE('',#29618,#30028,#25018,.T.) ;
#35451=EDGE_CURVE('',#30024,#29613,#25019,.T.) ;
#35452=EDGE_CURVE('',#29619,#30025,#25020,.T.) ;
#35453=EDGE_CURVE('',#29554,#30000,#25021,.T.) ;
#35454=EDGE_CURVE('',#30001,#29560,#25022,.T.) ;
#35455=EDGE_CURVE('',#30011,#30000,#25023,.T.) ;
#35456=EDGE_CURVE('',#29553,#30011,#25024,.T.) ;
#35457=EDGE_CURVE('',#30002,#29559,#25025,.T.) ;
#35458=EDGE_CURVE('',#30001,#30002,#25026,.T.) ;
#35459=EDGE_CURVE('',#30012,#29999,#25027,.T.) ;
#35460=EDGE_CURVE('',#29555,#30010,#25028,.T.) ;
#35461=EDGE_CURVE('',#29557,#30006,#25029,.T.) ;
#35462=EDGE_CURVE('',#30007,#29556,#25030,.T.) ;
#35463=EDGE_CURVE('',#30003,#29558,#25031,.T.) ;
#35464=EDGE_CURVE('',#29998,#30005,#25032,.T.) ;
#35465=EDGE_CURVE('',#29600,#29998,#25033,.T.) ;
#35466=EDGE_CURVE('',#29999,#29599,#25034,.T.) ;
#35467=EDGE_CURVE('',#30012,#29598,#25035,.T.) ;
#35468=EDGE_CURVE('',#30007,#30010,#25036,.T.) ;
#35469=EDGE_CURVE('',#30003,#30006,#25037,.T.) ;
#35470=EDGE_CURVE('',#29601,#30005,#25038,.T.) ;
#35471=EDGE_CURVE('',#30013,#29596,#25039,.T.) ;
#35472=EDGE_CURVE('',#30008,#30013,#25040,.T.) ;
#35473=EDGE_CURVE('',#30004,#30009,#25041,.T.) ;
#35474=EDGE_CURVE('',#29602,#30004,#25042,.T.) ;
#35475=EDGE_CURVE('',#30008,#29597,#25043,.T.) ;
#35476=EDGE_CURVE('',#29603,#30009,#25044,.T.) ;
#35477=EDGE_CURVE('',#29578,#29984,#25045,.T.) ;
#35478=EDGE_CURVE('',#29985,#29584,#25046,.T.) ;
#35479=EDGE_CURVE('',#29987,#29984,#25047,.T.) ;
#35480=EDGE_CURVE('',#29577,#29987,#25048,.T.) ;
#35481=EDGE_CURVE('',#29994,#29583,#25049,.T.) ;
#35482=EDGE_CURVE('',#29985,#29994,#25050,.T.) ;
#35483=EDGE_CURVE('',#29988,#29983,#25051,.T.) ;
#35484=EDGE_CURVE('',#29579,#29986,#25052,.T.) ;
#35485=EDGE_CURVE('',#29581,#29990,#25053,.T.) ;
#35486=EDGE_CURVE('',#29991,#29580,#25054,.T.) ;
#35487=EDGE_CURVE('',#29995,#29582,#25055,.T.) ;
#35488=EDGE_CURVE('',#29982,#29997,#25056,.T.) ;
#35489=EDGE_CURVE('',#29624,#29982,#25057,.T.) ;
#35490=EDGE_CURVE('',#29983,#29623,#25058,.T.) ;
#35491=EDGE_CURVE('',#29988,#29622,#25059,.T.) ;
#35492=EDGE_CURVE('',#29991,#29986,#25060,.T.) ;
#35493=EDGE_CURVE('',#29995,#29990,#25061,.T.) ;
#35494=EDGE_CURVE('',#29625,#29997,#25062,.T.) ;
#35495=EDGE_CURVE('',#29989,#29620,#25063,.T.) ;
#35496=EDGE_CURVE('',#29992,#29989,#25064,.T.) ;
#35497=EDGE_CURVE('',#29996,#29993,#25065,.T.) ;
#35498=EDGE_CURVE('',#29626,#29996,#25066,.T.) ;
#35499=EDGE_CURVE('',#29992,#29621,#25067,.T.) ;
#35500=EDGE_CURVE('',#29627,#29993,#25068,.T.) ;
#35501=EDGE_CURVE('',#29524,#30050,#25069,.T.) ;
#35502=EDGE_CURVE('',#30051,#29523,#25070,.T.) ;
#35503=EDGE_CURVE('',#30049,#29522,#25071,.T.) ;
#35504=EDGE_CURVE('',#30051,#30049,#25072,.T.) ;
#35505=EDGE_CURVE('',#30054,#30050,#25073,.T.) ;
#35506=EDGE_CURVE('',#29525,#30054,#25074,.T.) ;
#35507=EDGE_CURVE('',#30046,#29520,#25075,.T.) ;
#35508=EDGE_CURVE('',#30052,#30048,#25076,.T.) ;
#35509=EDGE_CURVE('',#30053,#29541,#25077,.T.) ;
#35510=EDGE_CURVE('',#29535,#30052,#25078,.T.) ;
#35511=EDGE_CURVE('',#30055,#30053,#25079,.T.) ;
#35512=EDGE_CURVE('',#29526,#30057,#25080,.T.) ;
#35513=EDGE_CURVE('',#29521,#30060,#25081,.T.) ;
#35514=EDGE_CURVE('',#30061,#29527,#25082,.T.) ;
#35515=EDGE_CURVE('',#30046,#30060,#25083,.T.) ;
#35516=EDGE_CURVE('',#29534,#30048,#25084,.T.) ;
#35517=EDGE_CURVE('',#30055,#29540,#25085,.T.) ;
#35518=EDGE_CURVE('',#30061,#30057,#25086,.T.) ;
#35519=EDGE_CURVE('',#30047,#30059,#25087,.T.) ;
#35520=EDGE_CURVE('',#29536,#30047,#25088,.T.) ;
#35521=EDGE_CURVE('',#30056,#29539,#25089,.T.) ;
#35522=EDGE_CURVE('',#30058,#30056,#25090,.T.) ;
#35523=EDGE_CURVE('',#29537,#30059,#25091,.T.) ;
#35524=EDGE_CURVE('',#30058,#29538,#25092,.T.) ;
#35525=EDGE_CURVE('',#29664,#29880,#25093,.T.) ;
#35526=EDGE_CURVE('',#29881,#29670,#25094,.T.) ;
#35527=EDGE_CURVE('',#29883,#29880,#25095,.T.) ;
#35528=EDGE_CURVE('',#29663,#29883,#25096,.T.) ;
#35529=EDGE_CURVE('',#29874,#29669,#25097,.T.) ;
#35530=EDGE_CURVE('',#29881,#29874,#25098,.T.) ;
#35531=EDGE_CURVE('',#29884,#29879,#25099,.T.) ;
#35532=EDGE_CURVE('',#29665,#29882,#25100,.T.) ;
#35533=EDGE_CURVE('',#29667,#29870,#25101,.T.) ;
#35534=EDGE_CURVE('',#29871,#29666,#25102,.T.) ;
#35535=EDGE_CURVE('',#29875,#29668,#25103,.T.) ;
#35536=EDGE_CURVE('',#29878,#29877,#25104,.T.) ;
#35537=EDGE_CURVE('',#29734,#29878,#25105,.T.) ;
#35538=EDGE_CURVE('',#29879,#29733,#25106,.T.) ;
#35539=EDGE_CURVE('',#29884,#29732,#25107,.T.) ;
#35540=EDGE_CURVE('',#29871,#29882,#25108,.T.) ;
#35541=EDGE_CURVE('',#29875,#29870,#25109,.T.) ;
#35542=EDGE_CURVE('',#29735,#29877,#25110,.T.) ;
#35543=EDGE_CURVE('',#29885,#29730,#25111,.T.) ;
#35544=EDGE_CURVE('',#29872,#29885,#25112,.T.) ;
#35545=EDGE_CURVE('',#29876,#29873,#25113,.T.) ;
#35546=EDGE_CURVE('',#29736,#29876,#25114,.T.) ;
#35547=EDGE_CURVE('',#29872,#29731,#25115,.T.) ;
#35548=EDGE_CURVE('',#29737,#29873,#25116,.T.) ;
#35549=EDGE_CURVE('',#29672,#29896,#25117,.T.) ;
#35550=EDGE_CURVE('',#29897,#29678,#25118,.T.) ;
#35551=EDGE_CURVE('',#29899,#29896,#25119,.T.) ;
#35552=EDGE_CURVE('',#29671,#29899,#25120,.T.) ;
#35553=EDGE_CURVE('',#29890,#29677,#25121,.T.) ;
#35554=EDGE_CURVE('',#29897,#29890,#25122,.T.) ;
#35555=EDGE_CURVE('',#29900,#29895,#25123,.T.) ;
#35556=EDGE_CURVE('',#29673,#29898,#25124,.T.) ;
#35557=EDGE_CURVE('',#29675,#29886,#25125,.T.) ;
#35558=EDGE_CURVE('',#29887,#29674,#25126,.T.) ;
#35559=EDGE_CURVE('',#29891,#29676,#25127,.T.) ;
#35560=EDGE_CURVE('',#29894,#29893,#25128,.T.) ;
#35561=EDGE_CURVE('',#29742,#29894,#25129,.T.) ;
#35562=EDGE_CURVE('',#29895,#29741,#25130,.T.) ;
#35563=EDGE_CURVE('',#29900,#29740,#25131,.T.) ;
#35564=EDGE_CURVE('',#29887,#29898,#25132,.T.) ;
#35565=EDGE_CURVE('',#29891,#29886,#25133,.T.) ;
#35566=EDGE_CURVE('',#29743,#29893,#25134,.T.) ;
#35567=EDGE_CURVE('',#29901,#29738,#25135,.T.) ;
#35568=EDGE_CURVE('',#29888,#29901,#25136,.T.) ;
#35569=EDGE_CURVE('',#29892,#29889,#25137,.T.) ;
#35570=EDGE_CURVE('',#29744,#29892,#25138,.T.) ;
#35571=EDGE_CURVE('',#29888,#29739,#25139,.T.) ;
#35572=EDGE_CURVE('',#29745,#29889,#25140,.T.) ;
#35573=EDGE_CURVE('',#29656,#29912,#25141,.T.) ;
#35574=EDGE_CURVE('',#29913,#29662,#25142,.T.) ;
#35575=EDGE_CURVE('',#29915,#29912,#25143,.T.) ;
#35576=EDGE_CURVE('',#29655,#29915,#25144,.T.) ;
#35577=EDGE_CURVE('',#29906,#29661,#25145,.T.) ;
#35578=EDGE_CURVE('',#29913,#29906,#25146,.T.) ;
#35579=EDGE_CURVE('',#29916,#29911,#25147,.T.) ;
#35580=EDGE_CURVE('',#29657,#29914,#25148,.T.) ;
#35581=EDGE_CURVE('',#29659,#29902,#25149,.T.) ;
#35582=EDGE_CURVE('',#29903,#29658,#25150,.T.) ;
#35583=EDGE_CURVE('',#29907,#29660,#25151,.T.) ;
#35584=EDGE_CURVE('',#29910,#29909,#25152,.T.) ;
#35585=EDGE_CURVE('',#29726,#29910,#25153,.T.) ;
#35586=EDGE_CURVE('',#29911,#29725,#25154,.T.) ;
#35587=EDGE_CURVE('',#29916,#29724,#25155,.T.) ;
#35588=EDGE_CURVE('',#29903,#29914,#25156,.T.) ;
#35589=EDGE_CURVE('',#29907,#29902,#25157,.T.) ;
#35590=EDGE_CURVE('',#29727,#29909,#25158,.T.) ;
#35591=EDGE_CURVE('',#29917,#29722,#25159,.T.) ;
#35592=EDGE_CURVE('',#29904,#29917,#25160,.T.) ;
#35593=EDGE_CURVE('',#29908,#29905,#25161,.T.) ;
#35594=EDGE_CURVE('',#29728,#29908,#25162,.T.) ;
#35595=EDGE_CURVE('',#29904,#29723,#25163,.T.) ;
#35596=EDGE_CURVE('',#29729,#29905,#25164,.T.) ;
#35597=EDGE_CURVE('',#29680,#29928,#25165,.T.) ;
#35598=EDGE_CURVE('',#29929,#29686,#25166,.T.) ;
#35599=EDGE_CURVE('',#29931,#29928,#25167,.T.) ;
#35600=EDGE_CURVE('',#29679,#29931,#25168,.T.) ;
#35601=EDGE_CURVE('',#29922,#29685,#25169,.T.) ;
#35602=EDGE_CURVE('',#29929,#29922,#25170,.T.) ;
#35603=EDGE_CURVE('',#29932,#29927,#25171,.T.) ;
#35604=EDGE_CURVE('',#29681,#29930,#25172,.T.) ;
#35605=EDGE_CURVE('',#29683,#29918,#25173,.T.) ;
#35606=EDGE_CURVE('',#29919,#29682,#25174,.T.) ;
#35607=EDGE_CURVE('',#29923,#29684,#25175,.T.) ;
#35608=EDGE_CURVE('',#29926,#29925,#25176,.T.) ;
#35609=EDGE_CURVE('',#29750,#29926,#25177,.T.) ;
#35610=EDGE_CURVE('',#29927,#29749,#25178,.T.) ;
#35611=EDGE_CURVE('',#29932,#29748,#25179,.T.) ;
#35612=EDGE_CURVE('',#29919,#29930,#25180,.T.) ;
#35613=EDGE_CURVE('',#29923,#29918,#25181,.T.) ;
#35614=EDGE_CURVE('',#29751,#29925,#25182,.T.) ;
#35615=EDGE_CURVE('',#29933,#29746,#25183,.T.) ;
#35616=EDGE_CURVE('',#29920,#29933,#25184,.T.) ;
#35617=EDGE_CURVE('',#29924,#29921,#25185,.T.) ;
#35618=EDGE_CURVE('',#29752,#29924,#25186,.T.) ;
#35619=EDGE_CURVE('',#29920,#29747,#25187,.T.) ;
#35620=EDGE_CURVE('',#29753,#29921,#25188,.T.) ;
#35621=EDGE_CURVE('',#29648,#29944,#25189,.T.) ;
#35622=EDGE_CURVE('',#29945,#29654,#25190,.T.) ;
#35623=EDGE_CURVE('',#29947,#29944,#25191,.T.) ;
#35624=EDGE_CURVE('',#29647,#29947,#25192,.T.) ;
#35625=EDGE_CURVE('',#29938,#29653,#25193,.T.) ;
#35626=EDGE_CURVE('',#29945,#29938,#25194,.T.) ;
#35627=EDGE_CURVE('',#29948,#29943,#25195,.T.) ;
#35628=EDGE_CURVE('',#29649,#29946,#25196,.T.) ;
#35629=EDGE_CURVE('',#29651,#29934,#25197,.T.) ;
#35630=EDGE_CURVE('',#29935,#29650,#25198,.T.) ;
#35631=EDGE_CURVE('',#29939,#29652,#25199,.T.) ;
#35632=EDGE_CURVE('',#29942,#29941,#25200,.T.) ;
#35633=EDGE_CURVE('',#29718,#29942,#25201,.T.) ;
#35634=EDGE_CURVE('',#29943,#29717,#25202,.T.) ;
#35635=EDGE_CURVE('',#29948,#29716,#25203,.T.) ;
#35636=EDGE_CURVE('',#29935,#29946,#25204,.T.) ;
#35637=EDGE_CURVE('',#29939,#29934,#25205,.T.) ;
#35638=EDGE_CURVE('',#29719,#29941,#25206,.T.) ;
#35639=EDGE_CURVE('',#29949,#29714,#25207,.T.) ;
#35640=EDGE_CURVE('',#29936,#29949,#25208,.T.) ;
#35641=EDGE_CURVE('',#29940,#29937,#25209,.T.) ;
#35642=EDGE_CURVE('',#29720,#29940,#25210,.T.) ;
#35643=EDGE_CURVE('',#29936,#29715,#25211,.T.) ;
#35644=EDGE_CURVE('',#29721,#29937,#25212,.T.) ;
#35645=EDGE_CURVE('',#29688,#29952,#25213,.T.) ;
#35646=EDGE_CURVE('',#29953,#29694,#25214,.T.) ;
#35647=EDGE_CURVE('',#29955,#29952,#25215,.T.) ;
#35648=EDGE_CURVE('',#29687,#29955,#25216,.T.) ;
#35649=EDGE_CURVE('',#29962,#29693,#25217,.T.) ;
#35650=EDGE_CURVE('',#29953,#29962,#25218,.T.) ;
#35651=EDGE_CURVE('',#29956,#29951,#25219,.T.) ;
#35652=EDGE_CURVE('',#29689,#29954,#25220,.T.) ;
#35653=EDGE_CURVE('',#29691,#29958,#25221,.T.) ;
#35654=EDGE_CURVE('',#29959,#29690,#25222,.T.) ;
#35655=EDGE_CURVE('',#29963,#29692,#25223,.T.) ;
#35656=EDGE_CURVE('',#29950,#29965,#25224,.T.) ;
#35657=EDGE_CURVE('',#29758,#29950,#25225,.T.) ;
#35658=EDGE_CURVE('',#29951,#29757,#25226,.T.) ;
#35659=EDGE_CURVE('',#29956,#29756,#25227,.T.) ;
#35660=EDGE_CURVE('',#29959,#29954,#25228,.T.) ;
#35661=EDGE_CURVE('',#29963,#29958,#25229,.T.) ;
#35662=EDGE_CURVE('',#29759,#29965,#25230,.T.) ;
#35663=EDGE_CURVE('',#29957,#29754,#25231,.T.) ;
#35664=EDGE_CURVE('',#29960,#29957,#25232,.T.) ;
#35665=EDGE_CURVE('',#29964,#29961,#25233,.T.) ;
#35666=EDGE_CURVE('',#29760,#29964,#25234,.T.) ;
#35667=EDGE_CURVE('',#29960,#29755,#25235,.T.) ;
#35668=EDGE_CURVE('',#29761,#29961,#25236,.T.) ;
#35669=EDGE_CURVE('',#29640,#29980,#25237,.T.) ;
#35670=EDGE_CURVE('',#29981,#29646,#25238,.T.) ;
#35671=EDGE_CURVE('',#29967,#29980,#25239,.T.) ;
#35672=EDGE_CURVE('',#29639,#29967,#25240,.T.) ;
#35673=EDGE_CURVE('',#29974,#29645,#25241,.T.) ;
#35674=EDGE_CURVE('',#29981,#29974,#25242,.T.) ;
#35675=EDGE_CURVE('',#29968,#29979,#25243,.T.) ;
#35676=EDGE_CURVE('',#29641,#29966,#25244,.T.) ;
#35677=EDGE_CURVE('',#29643,#29970,#25245,.T.) ;
#35678=EDGE_CURVE('',#29971,#29642,#25246,.T.) ;
#35679=EDGE_CURVE('',#29975,#29644,#25247,.T.) ;
#35680=EDGE_CURVE('',#29978,#29977,#25248,.T.) ;
#35681=EDGE_CURVE('',#29710,#29978,#25249,.T.) ;
#35682=EDGE_CURVE('',#29979,#29709,#25250,.T.) ;
#35683=EDGE_CURVE('',#29968,#29708,#25251,.T.) ;
#35684=EDGE_CURVE('',#29971,#29966,#25252,.T.) ;
#35685=EDGE_CURVE('',#29975,#29970,#25253,.T.) ;
#35686=EDGE_CURVE('',#29711,#29977,#25254,.T.) ;
#35687=EDGE_CURVE('',#29969,#29706,#25255,.T.) ;
#35688=EDGE_CURVE('',#29972,#29969,#25256,.T.) ;
#35689=EDGE_CURVE('',#29976,#29973,#25257,.T.) ;
#35690=EDGE_CURVE('',#29712,#29976,#25258,.T.) ;
#35691=EDGE_CURVE('',#29972,#29707,#25259,.T.) ;
#35692=EDGE_CURVE('',#29713,#29973,#25260,.T.) ;
#35693=EDGE_CURVE('',#29530,#29840,#4844,.T.) ;
#35694=EDGE_CURVE('',#29841,#29529,#25261,.T.) ;
#35695=EDGE_CURVE('',#29528,#29832,#25262,.T.) ;
#35696=EDGE_CURVE('',#29833,#29533,#4845,.T.) ;
#35697=EDGE_CURVE('',#29529,#29836,#25263,.T.) ;
#35698=EDGE_CURVE('',#29837,#29528,#25264,.T.) ;
#35699=EDGE_CURVE('',#29841,#29836,#25265,.T.) ;
#35700=EDGE_CURVE('',#29515,#29839,#4846,.T.) ;
#35701=EDGE_CURVE('',#29830,#29518,#4847,.T.) ;
#35702=EDGE_CURVE('',#29837,#29832,#25266,.T.) ;
#35703=EDGE_CURVE('',#29838,#29835,#25267,.T.) ;
#35704=EDGE_CURVE('',#29516,#29838,#25268,.T.) ;
#35705=EDGE_CURVE('',#29831,#29517,#25269,.T.) ;
#35706=EDGE_CURVE('',#29834,#29831,#25270,.T.) ;
#35707=EDGE_CURVE('',#29516,#29835,#25271,.T.) ;
#35708=EDGE_CURVE('',#29834,#29517,#25272,.T.) ;
#44066=ORIENTED_EDGE('',*,*,#34692,.F.) ;
#44067=ORIENTED_EDGE('',*,*,#34693,.F.) ;
#44068=ORIENTED_EDGE('',*,*,#34694,.T.) ;
#44069=ORIENTED_EDGE('',*,*,#34695,.F.) ;
#44070=ORIENTED_EDGE('',*,*,#34694,.F.) ;
#44071=ORIENTED_EDGE('',*,*,#34696,.F.) ;
#44072=ORIENTED_EDGE('',*,*,#34697,.T.) ;
#44073=ORIENTED_EDGE('',*,*,#34698,.F.) ;
#44074=ORIENTED_EDGE('',*,*,#34699,.F.) ;
#44075=ORIENTED_EDGE('',*,*,#34697,.F.) ;
#44076=ORIENTED_EDGE('',*,*,#34700,.F.) ;
#44077=ORIENTED_EDGE('',*,*,#34701,.F.) ;
#44078=ORIENTED_EDGE('',*,*,#34702,.T.) ;
#44079=ORIENTED_EDGE('',*,*,#34703,.F.) ;
#44080=ORIENTED_EDGE('',*,*,#34704,.F.) ;
#44081=ORIENTED_EDGE('',*,*,#34702,.F.) ;
#44082=ORIENTED_EDGE('',*,*,#34705,.F.) ;
#44083=ORIENTED_EDGE('',*,*,#34706,.T.) ;
#44084=ORIENTED_EDGE('',*,*,#34707,.F.) ;
#44085=ORIENTED_EDGE('',*,*,#34706,.F.) ;
#44086=ORIENTED_EDGE('',*,*,#34708,.F.) ;
#44087=ORIENTED_EDGE('',*,*,#34709,.F.) ;
#44088=ORIENTED_EDGE('',*,*,#34710,.T.) ;
#44089=ORIENTED_EDGE('',*,*,#34711,.F.) ;
#44090=ORIENTED_EDGE('',*,*,#34712,.F.) ;
#44091=ORIENTED_EDGE('',*,*,#34710,.F.) ;
#44092=ORIENTED_EDGE('',*,*,#34713,.F.) ;
#44093=ORIENTED_EDGE('',*,*,#34714,.T.) ;
#44094=ORIENTED_EDGE('',*,*,#34715,.F.) ;
#44095=ORIENTED_EDGE('',*,*,#34714,.F.) ;
#44096=ORIENTED_EDGE('',*,*,#34708,.T.) ;
#44097=ORIENTED_EDGE('',*,*,#34709,.T.) ;
#44098=ORIENTED_EDGE('',*,*,#34716,.T.) ;
#44099=ORIENTED_EDGE('',*,*,#34717,.T.) ;
#44100=ORIENTED_EDGE('',*,*,#34716,.F.) ;
#44101=ORIENTED_EDGE('',*,*,#34715,.T.) ;
#44102=ORIENTED_EDGE('',*,*,#34718,.T.) ;
#44103=ORIENTED_EDGE('',*,*,#34711,.T.) ;
#44104=ORIENTED_EDGE('',*,*,#34712,.T.) ;
#44105=ORIENTED_EDGE('',*,*,#34718,.F.) ;
#44106=ORIENTED_EDGE('',*,*,#34700,.T.) ;
#44107=ORIENTED_EDGE('',*,*,#34701,.T.) ;
#44108=ORIENTED_EDGE('',*,*,#34719,.T.) ;
#44109=ORIENTED_EDGE('',*,*,#34720,.T.) ;
#44110=ORIENTED_EDGE('',*,*,#34719,.F.) ;
#44111=ORIENTED_EDGE('',*,*,#34707,.T.) ;
#44112=ORIENTED_EDGE('',*,*,#34721,.T.) ;
#44113=ORIENTED_EDGE('',*,*,#34703,.T.) ;
#44114=ORIENTED_EDGE('',*,*,#34704,.T.) ;
#44115=ORIENTED_EDGE('',*,*,#34721,.F.) ;
#44116=ORIENTED_EDGE('',*,*,#34692,.T.) ;
#44117=ORIENTED_EDGE('',*,*,#34693,.T.) ;
#44118=ORIENTED_EDGE('',*,*,#34722,.T.) ;
#44119=ORIENTED_EDGE('',*,*,#34698,.T.) ;
#44120=ORIENTED_EDGE('',*,*,#34699,.T.) ;
#44121=ORIENTED_EDGE('',*,*,#34722,.F.) ;
#44122=ORIENTED_EDGE('',*,*,#34723,.T.) ;
#44123=ORIENTED_EDGE('',*,*,#34724,.T.) ;
#44124=ORIENTED_EDGE('',*,*,#34725,.T.) ;
#44125=ORIENTED_EDGE('',*,*,#34726,.T.) ;
#44126=ORIENTED_EDGE('',*,*,#34727,.F.) ;
#44127=ORIENTED_EDGE('',*,*,#34728,.F.) ;
#44128=ORIENTED_EDGE('',*,*,#34729,.F.) ;
#44129=ORIENTED_EDGE('',*,*,#34730,.T.) ;
#44130=ORIENTED_EDGE('',*,*,#34731,.F.) ;
#44131=ORIENTED_EDGE('',*,*,#34732,.T.) ;
#44132=ORIENTED_EDGE('',*,*,#34733,.F.) ;
#44133=ORIENTED_EDGE('',*,*,#34734,.T.) ;
#44134=ORIENTED_EDGE('',*,*,#34735,.F.) ;
#44135=ORIENTED_EDGE('',*,*,#34736,.T.) ;
#44136=ORIENTED_EDGE('',*,*,#34696,.T.) ;
#44137=ORIENTED_EDGE('',*,*,#34737,.T.) ;
#44138=ORIENTED_EDGE('',*,*,#34738,.T.) ;
#44139=ORIENTED_EDGE('',*,*,#34739,.F.) ;
#44140=ORIENTED_EDGE('',*,*,#34740,.F.) ;
#44141=ORIENTED_EDGE('',*,*,#34741,.T.) ;
#44142=ORIENTED_EDGE('',*,*,#34742,.T.) ;
#44143=ORIENTED_EDGE('',*,*,#34743,.F.) ;
#44144=ORIENTED_EDGE('',*,*,#34744,.T.) ;
#44145=ORIENTED_EDGE('',*,*,#34745,.F.) ;
#44146=ORIENTED_EDGE('',*,*,#34746,.T.) ;
#44147=ORIENTED_EDGE('',*,*,#34747,.F.) ;
#44148=ORIENTED_EDGE('',*,*,#34748,.T.) ;
#44149=ORIENTED_EDGE('',*,*,#34749,.F.) ;
#44150=ORIENTED_EDGE('',*,*,#34750,.T.) ;
#44151=ORIENTED_EDGE('',*,*,#34695,.T.) ;
#44152=ORIENTED_EDGE('',*,*,#34751,.F.) ;
#44153=ORIENTED_EDGE('',*,*,#34752,.T.) ;
#44154=ORIENTED_EDGE('',*,*,#34753,.F.) ;
#44155=ORIENTED_EDGE('',*,*,#34754,.F.) ;
#44156=ORIENTED_EDGE('',*,*,#34755,.T.) ;
#44157=ORIENTED_EDGE('',*,*,#34756,.T.) ;
#44158=ORIENTED_EDGE('',*,*,#34757,.T.) ;
#44159=ORIENTED_EDGE('',*,*,#34758,.F.) ;
#44160=ORIENTED_EDGE('',*,*,#34759,.T.) ;
#44161=ORIENTED_EDGE('',*,*,#34760,.T.) ;
#44162=ORIENTED_EDGE('',*,*,#34761,.T.) ;
#44163=ORIENTED_EDGE('',*,*,#34762,.F.) ;
#44164=ORIENTED_EDGE('',*,*,#34763,.T.) ;
#44165=ORIENTED_EDGE('',*,*,#34764,.F.) ;
#44166=ORIENTED_EDGE('',*,*,#34765,.T.) ;
#44167=ORIENTED_EDGE('',*,*,#34766,.F.) ;
#44168=ORIENTED_EDGE('',*,*,#34767,.T.) ;
#44169=ORIENTED_EDGE('',*,*,#34768,.F.) ;
#44170=ORIENTED_EDGE('',*,*,#34769,.T.) ;
#44171=ORIENTED_EDGE('',*,*,#34770,.F.) ;
#44172=ORIENTED_EDGE('',*,*,#34771,.T.) ;
#44173=ORIENTED_EDGE('',*,*,#34772,.F.) ;
#44174=ORIENTED_EDGE('',*,*,#34773,.T.) ;
#44175=ORIENTED_EDGE('',*,*,#34774,.F.) ;
#44176=ORIENTED_EDGE('',*,*,#34775,.T.) ;
#44177=ORIENTED_EDGE('',*,*,#34776,.F.) ;
#44178=ORIENTED_EDGE('',*,*,#34777,.T.) ;
#44179=ORIENTED_EDGE('',*,*,#34778,.F.) ;
#44180=ORIENTED_EDGE('',*,*,#34779,.T.) ;
#44181=ORIENTED_EDGE('',*,*,#34780,.F.) ;
#44182=ORIENTED_EDGE('',*,*,#34781,.T.) ;
#44183=ORIENTED_EDGE('',*,*,#34782,.F.) ;
#44184=ORIENTED_EDGE('',*,*,#34783,.T.) ;
#44185=ORIENTED_EDGE('',*,*,#34784,.F.) ;
#44186=ORIENTED_EDGE('',*,*,#34785,.T.) ;
#44187=ORIENTED_EDGE('',*,*,#34786,.F.) ;
#44188=ORIENTED_EDGE('',*,*,#34787,.T.) ;
#44189=ORIENTED_EDGE('',*,*,#34788,.F.) ;
#44190=ORIENTED_EDGE('',*,*,#34789,.T.) ;
#44191=ORIENTED_EDGE('',*,*,#34790,.F.) ;
#44192=ORIENTED_EDGE('',*,*,#34791,.T.) ;
#44193=ORIENTED_EDGE('',*,*,#34792,.F.) ;
#44194=ORIENTED_EDGE('',*,*,#34793,.T.) ;
#44195=ORIENTED_EDGE('',*,*,#34794,.T.) ;
#44196=ORIENTED_EDGE('',*,*,#34795,.T.) ;
#44197=ORIENTED_EDGE('',*,*,#34796,.F.) ;
#44198=ORIENTED_EDGE('',*,*,#34797,.T.) ;
#44199=ORIENTED_EDGE('',*,*,#34798,.T.) ;
#44200=ORIENTED_EDGE('',*,*,#34799,.T.) ;
#44201=ORIENTED_EDGE('',*,*,#34800,.F.) ;
#44202=ORIENTED_EDGE('',*,*,#34801,.T.) ;
#44203=ORIENTED_EDGE('',*,*,#34802,.T.) ;
#44204=ORIENTED_EDGE('',*,*,#34803,.T.) ;
#44205=ORIENTED_EDGE('',*,*,#34804,.T.) ;
#44206=ORIENTED_EDGE('',*,*,#34805,.F.) ;
#44207=ORIENTED_EDGE('',*,*,#34806,.T.) ;
#44208=ORIENTED_EDGE('',*,*,#34807,.F.) ;
#44209=ORIENTED_EDGE('',*,*,#34808,.T.) ;
#44210=ORIENTED_EDGE('',*,*,#34809,.F.) ;
#44211=ORIENTED_EDGE('',*,*,#34810,.T.) ;
#44212=ORIENTED_EDGE('',*,*,#34811,.F.) ;
#44213=ORIENTED_EDGE('',*,*,#34812,.T.) ;
#44214=ORIENTED_EDGE('',*,*,#34813,.F.) ;
#44215=ORIENTED_EDGE('',*,*,#34814,.T.) ;
#44216=ORIENTED_EDGE('',*,*,#34815,.F.) ;
#44217=ORIENTED_EDGE('',*,*,#34816,.T.) ;
#44218=ORIENTED_EDGE('',*,*,#34817,.F.) ;
#44219=ORIENTED_EDGE('',*,*,#34818,.T.) ;
#44220=ORIENTED_EDGE('',*,*,#34819,.F.) ;
#44221=ORIENTED_EDGE('',*,*,#34820,.T.) ;
#44222=ORIENTED_EDGE('',*,*,#34821,.F.) ;
#44223=ORIENTED_EDGE('',*,*,#34822,.T.) ;
#44224=ORIENTED_EDGE('',*,*,#34823,.F.) ;
#44225=ORIENTED_EDGE('',*,*,#34824,.T.) ;
#44226=ORIENTED_EDGE('',*,*,#34825,.F.) ;
#44227=ORIENTED_EDGE('',*,*,#34826,.T.) ;
#44228=ORIENTED_EDGE('',*,*,#34827,.F.) ;
#44229=ORIENTED_EDGE('',*,*,#34828,.T.) ;
#44230=ORIENTED_EDGE('',*,*,#34829,.F.) ;
#44231=ORIENTED_EDGE('',*,*,#34830,.T.) ;
#44232=ORIENTED_EDGE('',*,*,#34831,.F.) ;
#44233=ORIENTED_EDGE('',*,*,#34832,.T.) ;
#44234=ORIENTED_EDGE('',*,*,#34833,.F.) ;
#44235=ORIENTED_EDGE('',*,*,#34834,.T.) ;
#44236=ORIENTED_EDGE('',*,*,#34835,.F.) ;
#44237=ORIENTED_EDGE('',*,*,#34836,.T.) ;
#44238=ORIENTED_EDGE('',*,*,#34837,.T.) ;
#44239=ORIENTED_EDGE('',*,*,#34838,.T.) ;
#44240=ORIENTED_EDGE('',*,*,#34839,.F.) ;
#44241=ORIENTED_EDGE('',*,*,#34840,.T.) ;
#44242=ORIENTED_EDGE('',*,*,#34841,.T.) ;
#44243=ORIENTED_EDGE('',*,*,#34842,.T.) ;
#44244=ORIENTED_EDGE('',*,*,#34843,.F.) ;
#44245=ORIENTED_EDGE('',*,*,#34844,.T.) ;
#44246=ORIENTED_EDGE('',*,*,#34845,.T.) ;
#44247=ORIENTED_EDGE('',*,*,#34846,.T.) ;
#44248=ORIENTED_EDGE('',*,*,#34847,.T.) ;
#44249=ORIENTED_EDGE('',*,*,#34848,.F.) ;
#44250=ORIENTED_EDGE('',*,*,#34849,.T.) ;
#44251=ORIENTED_EDGE('',*,*,#34850,.F.) ;
#44252=ORIENTED_EDGE('',*,*,#34851,.T.) ;
#44253=ORIENTED_EDGE('',*,*,#34852,.F.) ;
#44254=ORIENTED_EDGE('',*,*,#34853,.T.) ;
#44255=ORIENTED_EDGE('',*,*,#34854,.F.) ;
#44256=ORIENTED_EDGE('',*,*,#34855,.T.) ;
#44257=ORIENTED_EDGE('',*,*,#34856,.F.) ;
#44258=ORIENTED_EDGE('',*,*,#34857,.T.) ;
#44259=ORIENTED_EDGE('',*,*,#34858,.F.) ;
#44260=ORIENTED_EDGE('',*,*,#34859,.T.) ;
#44261=ORIENTED_EDGE('',*,*,#34860,.F.) ;
#44262=ORIENTED_EDGE('',*,*,#34861,.T.) ;
#44263=ORIENTED_EDGE('',*,*,#34862,.F.) ;
#44264=ORIENTED_EDGE('',*,*,#34863,.T.) ;
#44265=ORIENTED_EDGE('',*,*,#34864,.F.) ;
#44266=ORIENTED_EDGE('',*,*,#34865,.T.) ;
#44267=ORIENTED_EDGE('',*,*,#34866,.F.) ;
#44268=ORIENTED_EDGE('',*,*,#34867,.T.) ;
#44269=ORIENTED_EDGE('',*,*,#34868,.F.) ;
#44270=ORIENTED_EDGE('',*,*,#34869,.T.) ;
#44271=ORIENTED_EDGE('',*,*,#34870,.F.) ;
#44272=ORIENTED_EDGE('',*,*,#34871,.T.) ;
#44273=ORIENTED_EDGE('',*,*,#34872,.F.) ;
#44274=ORIENTED_EDGE('',*,*,#34873,.T.) ;
#44275=ORIENTED_EDGE('',*,*,#34874,.F.) ;
#44276=ORIENTED_EDGE('',*,*,#34875,.T.) ;
#44277=ORIENTED_EDGE('',*,*,#34876,.F.) ;
#44278=ORIENTED_EDGE('',*,*,#34877,.T.) ;
#44279=ORIENTED_EDGE('',*,*,#34878,.F.) ;
#44280=ORIENTED_EDGE('',*,*,#34879,.T.) ;
#44281=ORIENTED_EDGE('',*,*,#34880,.F.) ;
#44282=ORIENTED_EDGE('',*,*,#34881,.T.) ;
#44283=ORIENTED_EDGE('',*,*,#34882,.F.) ;
#44284=ORIENTED_EDGE('',*,*,#34883,.T.) ;
#44285=ORIENTED_EDGE('',*,*,#34884,.F.) ;
#44286=ORIENTED_EDGE('',*,*,#34885,.T.) ;
#44287=ORIENTED_EDGE('',*,*,#34886,.F.) ;
#44288=ORIENTED_EDGE('',*,*,#34887,.T.) ;
#44289=ORIENTED_EDGE('',*,*,#34888,.F.) ;
#44290=ORIENTED_EDGE('',*,*,#34889,.T.) ;
#44291=ORIENTED_EDGE('',*,*,#34890,.F.) ;
#44292=ORIENTED_EDGE('',*,*,#34891,.T.) ;
#44293=ORIENTED_EDGE('',*,*,#34892,.F.) ;
#44294=ORIENTED_EDGE('',*,*,#34893,.T.) ;
#44295=ORIENTED_EDGE('',*,*,#34894,.F.) ;
#44296=ORIENTED_EDGE('',*,*,#34895,.T.) ;
#44297=ORIENTED_EDGE('',*,*,#34896,.F.) ;
#44298=ORIENTED_EDGE('',*,*,#34897,.T.) ;
#44299=ORIENTED_EDGE('',*,*,#34898,.F.) ;
#44300=ORIENTED_EDGE('',*,*,#34899,.T.) ;
#44301=ORIENTED_EDGE('',*,*,#34900,.F.) ;
#44302=ORIENTED_EDGE('',*,*,#34901,.T.) ;
#44303=ORIENTED_EDGE('',*,*,#34902,.F.) ;
#44304=ORIENTED_EDGE('',*,*,#34903,.T.) ;
#44305=ORIENTED_EDGE('',*,*,#34904,.F.) ;
#44306=ORIENTED_EDGE('',*,*,#34905,.T.) ;
#44307=ORIENTED_EDGE('',*,*,#34906,.F.) ;
#44308=ORIENTED_EDGE('',*,*,#34907,.F.) ;
#44309=ORIENTED_EDGE('',*,*,#34908,.T.) ;
#44310=ORIENTED_EDGE('',*,*,#34909,.T.) ;
#44311=ORIENTED_EDGE('',*,*,#34910,.T.) ;
#44312=ORIENTED_EDGE('',*,*,#34911,.F.) ;
#44313=ORIENTED_EDGE('',*,*,#34912,.T.) ;
#44314=ORIENTED_EDGE('',*,*,#34913,.T.) ;
#44315=ORIENTED_EDGE('',*,*,#34914,.T.) ;
#44316=ORIENTED_EDGE('',*,*,#34915,.F.) ;
#44317=ORIENTED_EDGE('',*,*,#34916,.T.) ;
#44318=ORIENTED_EDGE('',*,*,#34917,.F.) ;
#44319=ORIENTED_EDGE('',*,*,#34918,.T.) ;
#44320=ORIENTED_EDGE('',*,*,#34919,.F.) ;
#44321=ORIENTED_EDGE('',*,*,#34920,.T.) ;
#44322=ORIENTED_EDGE('',*,*,#34921,.F.) ;
#44323=ORIENTED_EDGE('',*,*,#34922,.T.) ;
#44324=ORIENTED_EDGE('',*,*,#34923,.F.) ;
#44325=ORIENTED_EDGE('',*,*,#34924,.T.) ;
#44326=ORIENTED_EDGE('',*,*,#34925,.F.) ;
#44327=ORIENTED_EDGE('',*,*,#34926,.T.) ;
#44328=ORIENTED_EDGE('',*,*,#34927,.F.) ;
#44329=ORIENTED_EDGE('',*,*,#34928,.T.) ;
#44330=ORIENTED_EDGE('',*,*,#34929,.F.) ;
#44331=ORIENTED_EDGE('',*,*,#34930,.T.) ;
#44332=ORIENTED_EDGE('',*,*,#34931,.F.) ;
#44333=ORIENTED_EDGE('',*,*,#34932,.T.) ;
#44334=ORIENTED_EDGE('',*,*,#34933,.F.) ;
#44335=ORIENTED_EDGE('',*,*,#34934,.T.) ;
#44336=ORIENTED_EDGE('',*,*,#34935,.F.) ;
#44337=ORIENTED_EDGE('',*,*,#34936,.T.) ;
#44338=ORIENTED_EDGE('',*,*,#34937,.F.) ;
#44339=ORIENTED_EDGE('',*,*,#34938,.T.) ;
#44340=ORIENTED_EDGE('',*,*,#34939,.F.) ;
#44341=ORIENTED_EDGE('',*,*,#34940,.T.) ;
#44342=ORIENTED_EDGE('',*,*,#34941,.F.) ;
#44343=ORIENTED_EDGE('',*,*,#34942,.T.) ;
#44344=ORIENTED_EDGE('',*,*,#34943,.F.) ;
#44345=ORIENTED_EDGE('',*,*,#34944,.T.) ;
#44346=ORIENTED_EDGE('',*,*,#34945,.F.) ;
#44347=ORIENTED_EDGE('',*,*,#34946,.T.) ;
#44348=ORIENTED_EDGE('',*,*,#34947,.F.) ;
#44349=ORIENTED_EDGE('',*,*,#34948,.T.) ;
#44350=ORIENTED_EDGE('',*,*,#34949,.F.) ;
#44351=ORIENTED_EDGE('',*,*,#34950,.T.) ;
#44352=ORIENTED_EDGE('',*,*,#34951,.F.) ;
#44353=ORIENTED_EDGE('',*,*,#34952,.T.) ;
#44354=ORIENTED_EDGE('',*,*,#34953,.F.) ;
#44355=ORIENTED_EDGE('',*,*,#34954,.T.) ;
#44356=ORIENTED_EDGE('',*,*,#34955,.F.) ;
#44357=ORIENTED_EDGE('',*,*,#34956,.T.) ;
#44358=ORIENTED_EDGE('',*,*,#34957,.F.) ;
#44359=ORIENTED_EDGE('',*,*,#34958,.T.) ;
#44360=ORIENTED_EDGE('',*,*,#34959,.F.) ;
#44361=ORIENTED_EDGE('',*,*,#34960,.T.) ;
#44362=ORIENTED_EDGE('',*,*,#34961,.F.) ;
#44363=ORIENTED_EDGE('',*,*,#34962,.T.) ;
#44364=ORIENTED_EDGE('',*,*,#34963,.F.) ;
#44365=ORIENTED_EDGE('',*,*,#34964,.T.) ;
#44366=ORIENTED_EDGE('',*,*,#34965,.F.) ;
#44367=ORIENTED_EDGE('',*,*,#34966,.T.) ;
#44368=ORIENTED_EDGE('',*,*,#34967,.F.) ;
#44369=ORIENTED_EDGE('',*,*,#34968,.T.) ;
#44370=ORIENTED_EDGE('',*,*,#34969,.F.) ;
#44371=ORIENTED_EDGE('',*,*,#34970,.T.) ;
#44372=ORIENTED_EDGE('',*,*,#34971,.F.) ;
#44373=ORIENTED_EDGE('',*,*,#34972,.T.) ;
#44374=ORIENTED_EDGE('',*,*,#34973,.F.) ;
#44375=ORIENTED_EDGE('',*,*,#34974,.T.) ;
#44376=ORIENTED_EDGE('',*,*,#34975,.T.) ;
#44377=ORIENTED_EDGE('',*,*,#34976,.T.) ;
#44378=ORIENTED_EDGE('',*,*,#34977,.F.) ;
#44379=ORIENTED_EDGE('',*,*,#34978,.T.) ;
#44380=ORIENTED_EDGE('',*,*,#34979,.T.) ;
#44381=ORIENTED_EDGE('',*,*,#34980,.T.) ;
#44382=ORIENTED_EDGE('',*,*,#34717,.F.) ;
#44383=ORIENTED_EDGE('',*,*,#34720,.F.) ;
#44384=ORIENTED_EDGE('',*,*,#34981,.T.) ;
#44385=ORIENTED_EDGE('',*,*,#34982,.T.) ;
#44386=ORIENTED_EDGE('',*,*,#34983,.F.) ;
#44387=ORIENTED_EDGE('',*,*,#34984,.T.) ;
#44388=ORIENTED_EDGE('',*,*,#34985,.T.) ;
#44389=ORIENTED_EDGE('',*,*,#34986,.T.) ;
#44390=ORIENTED_EDGE('',*,*,#34987,.F.) ;
#44391=ORIENTED_EDGE('',*,*,#34988,.T.) ;
#44392=ORIENTED_EDGE('',*,*,#34989,.F.) ;
#44393=ORIENTED_EDGE('',*,*,#34990,.F.) ;
#44394=ORIENTED_EDGE('',*,*,#34713,.T.) ;
#44395=ORIENTED_EDGE('',*,*,#34705,.T.) ;
#44396=ORIENTED_EDGE('',*,*,#34991,.T.) ;
#44397=ORIENTED_EDGE('',*,*,#34992,.T.) ;
#44398=ORIENTED_EDGE('',*,*,#34993,.T.) ;
#44399=ORIENTED_EDGE('',*,*,#34994,.T.) ;
#44400=ORIENTED_EDGE('',*,*,#34995,.T.) ;
#44401=ORIENTED_EDGE('',*,*,#34996,.T.) ;
#44402=ORIENTED_EDGE('',*,*,#34997,.T.) ;
#44403=ORIENTED_EDGE('',*,*,#34998,.T.) ;
#44404=ORIENTED_EDGE('',*,*,#34999,.T.) ;
#44405=ORIENTED_EDGE('',*,*,#35000,.T.) ;
#44406=ORIENTED_EDGE('',*,*,#35001,.T.) ;
#44407=ORIENTED_EDGE('',*,*,#35002,.T.) ;
#44408=ORIENTED_EDGE('',*,*,#35003,.T.) ;
#44409=ORIENTED_EDGE('',*,*,#35004,.T.) ;
#44410=ORIENTED_EDGE('',*,*,#35005,.T.) ;
#44411=ORIENTED_EDGE('',*,*,#35006,.T.) ;
#44412=ORIENTED_EDGE('',*,*,#35007,.T.) ;
#44413=ORIENTED_EDGE('',*,*,#35008,.T.) ;
#44414=ORIENTED_EDGE('',*,*,#35009,.T.) ;
#44415=ORIENTED_EDGE('',*,*,#35010,.T.) ;
#44416=ORIENTED_EDGE('',*,*,#34997,.F.) ;
#44417=ORIENTED_EDGE('',*,*,#35011,.T.) ;
#44418=ORIENTED_EDGE('',*,*,#35012,.F.) ;
#44419=ORIENTED_EDGE('',*,*,#35013,.T.) ;
#44420=ORIENTED_EDGE('',*,*,#35014,.T.) ;
#44421=ORIENTED_EDGE('',*,*,#35015,.T.) ;
#44422=ORIENTED_EDGE('',*,*,#35016,.F.) ;
#44423=ORIENTED_EDGE('',*,*,#35017,.T.) ;
#44424=ORIENTED_EDGE('',*,*,#34973,.T.) ;
#44425=ORIENTED_EDGE('',*,*,#35018,.T.) ;
#44426=ORIENTED_EDGE('',*,*,#34837,.F.) ;
#44427=ORIENTED_EDGE('',*,*,#35016,.T.) ;
#44428=ORIENTED_EDGE('',*,*,#34906,.T.) ;
#44429=ORIENTED_EDGE('',*,*,#35019,.T.) ;
#44430=ORIENTED_EDGE('',*,*,#34981,.F.) ;
#44431=ORIENTED_EDGE('',*,*,#35014,.F.) ;
#44432=ORIENTED_EDGE('',*,*,#35020,.T.) ;
#44433=ORIENTED_EDGE('',*,*,#35021,.T.) ;
#44434=ORIENTED_EDGE('',*,*,#35022,.T.) ;
#44435=ORIENTED_EDGE('',*,*,#35023,.T.) ;
#44436=ORIENTED_EDGE('',*,*,#35024,.T.) ;
#44437=ORIENTED_EDGE('',*,*,#35025,.T.) ;
#44438=ORIENTED_EDGE('',*,*,#35026,.T.) ;
#44439=ORIENTED_EDGE('',*,*,#35027,.T.) ;
#44440=ORIENTED_EDGE('',*,*,#35028,.T.) ;
#44441=ORIENTED_EDGE('',*,*,#35029,.T.) ;
#44442=ORIENTED_EDGE('',*,*,#35030,.T.) ;
#44443=ORIENTED_EDGE('',*,*,#35031,.T.) ;
#44444=ORIENTED_EDGE('',*,*,#35032,.T.) ;
#44445=ORIENTED_EDGE('',*,*,#35033,.T.) ;
#44446=ORIENTED_EDGE('',*,*,#35034,.T.) ;
#44447=ORIENTED_EDGE('',*,*,#35035,.T.) ;
#44448=ORIENTED_EDGE('',*,*,#35036,.T.) ;
#44449=ORIENTED_EDGE('',*,*,#35037,.T.) ;
#44450=ORIENTED_EDGE('',*,*,#35038,.T.) ;
#44451=ORIENTED_EDGE('',*,*,#35039,.T.) ;
#44452=ORIENTED_EDGE('',*,*,#35040,.T.) ;
#44453=ORIENTED_EDGE('',*,*,#35041,.T.) ;
#44454=ORIENTED_EDGE('',*,*,#35042,.T.) ;
#44455=ORIENTED_EDGE('',*,*,#35043,.T.) ;
#44456=ORIENTED_EDGE('',*,*,#35012,.T.) ;
#44457=ORIENTED_EDGE('',*,*,#35044,.T.) ;
#44458=ORIENTED_EDGE('',*,*,#35045,.T.) ;
#44459=ORIENTED_EDGE('',*,*,#35046,.T.) ;
#44460=ORIENTED_EDGE('',*,*,#34847,.F.) ;
#44461=ORIENTED_EDGE('',*,*,#35047,.T.) ;
#44462=ORIENTED_EDGE('',*,*,#34907,.T.) ;
#44463=ORIENTED_EDGE('',*,*,#35017,.F.) ;
#44464=ORIENTED_EDGE('',*,*,#35048,.T.) ;
#44465=ORIENTED_EDGE('',*,*,#35049,.T.) ;
#44466=ORIENTED_EDGE('',*,*,#35050,.T.) ;
#44467=ORIENTED_EDGE('',*,*,#35051,.T.) ;
#44468=ORIENTED_EDGE('',*,*,#35052,.T.) ;
#44469=ORIENTED_EDGE('',*,*,#35053,.T.) ;
#44470=ORIENTED_EDGE('',*,*,#35054,.T.) ;
#44471=ORIENTED_EDGE('',*,*,#35055,.T.) ;
#44472=ORIENTED_EDGE('',*,*,#35056,.T.) ;
#44473=ORIENTED_EDGE('',*,*,#35057,.T.) ;
#44474=ORIENTED_EDGE('',*,*,#35058,.T.) ;
#44475=ORIENTED_EDGE('',*,*,#35059,.T.) ;
#44476=ORIENTED_EDGE('',*,*,#34739,.T.) ;
#44477=ORIENTED_EDGE('',*,*,#35060,.T.) ;
#44478=ORIENTED_EDGE('',*,*,#34723,.F.) ;
#44479=ORIENTED_EDGE('',*,*,#35061,.F.) ;
#44480=ORIENTED_EDGE('',*,*,#34727,.T.) ;
#44481=ORIENTED_EDGE('',*,*,#35062,.T.) ;
#44482=ORIENTED_EDGE('',*,*,#34741,.F.) ;
#44483=ORIENTED_EDGE('',*,*,#35063,.T.) ;
#44484=ORIENTED_EDGE('',*,*,#35063,.F.) ;
#44485=ORIENTED_EDGE('',*,*,#35064,.T.) ;
#44486=ORIENTED_EDGE('',*,*,#35065,.T.) ;
#44487=ORIENTED_EDGE('',*,*,#35066,.F.) ;
#44488=ORIENTED_EDGE('',*,*,#35067,.T.) ;
#44489=ORIENTED_EDGE('',*,*,#35061,.T.) ;
#44490=ORIENTED_EDGE('',*,*,#35068,.F.) ;
#44491=ORIENTED_EDGE('',*,*,#35015,.F.) ;
#44492=ORIENTED_EDGE('',*,*,#34974,.F.) ;
#44493=ORIENTED_EDGE('',*,*,#35068,.T.) ;
#44494=ORIENTED_EDGE('',*,*,#34728,.T.) ;
#44495=ORIENTED_EDGE('',*,*,#35066,.T.) ;
#44496=ORIENTED_EDGE('',*,*,#34990,.T.) ;
#44497=ORIENTED_EDGE('',*,*,#35064,.F.) ;
#44498=ORIENTED_EDGE('',*,*,#34740,.T.) ;
#44499=ORIENTED_EDGE('',*,*,#35067,.F.) ;
#44500=ORIENTED_EDGE('',*,*,#35069,.F.) ;
#44501=ORIENTED_EDGE('',*,*,#35070,.T.) ;
#44502=ORIENTED_EDGE('',*,*,#34991,.F.) ;
#44503=ORIENTED_EDGE('',*,*,#35071,.T.) ;
#44504=ORIENTED_EDGE('',*,*,#35072,.T.) ;
#44505=ORIENTED_EDGE('',*,*,#35073,.T.) ;
#44506=ORIENTED_EDGE('',*,*,#35074,.F.) ;
#44507=ORIENTED_EDGE('',*,*,#35065,.F.) ;
#44508=ORIENTED_EDGE('',*,*,#34753,.T.) ;
#44509=ORIENTED_EDGE('',*,*,#35075,.T.) ;
#44510=ORIENTED_EDGE('',*,*,#34975,.F.) ;
#44511=ORIENTED_EDGE('',*,*,#35074,.T.) ;
#44512=ORIENTED_EDGE('',*,*,#34989,.T.) ;
#44513=ORIENTED_EDGE('',*,*,#35076,.T.) ;
#44514=ORIENTED_EDGE('',*,*,#34794,.F.) ;
#44515=ORIENTED_EDGE('',*,*,#35072,.F.) ;
#44516=ORIENTED_EDGE('',*,*,#35077,.T.) ;
#44517=ORIENTED_EDGE('',*,*,#35078,.T.) ;
#44518=ORIENTED_EDGE('',*,*,#35079,.T.) ;
#44519=ORIENTED_EDGE('',*,*,#35080,.T.) ;
#44520=ORIENTED_EDGE('',*,*,#35081,.T.) ;
#44521=ORIENTED_EDGE('',*,*,#35082,.T.) ;
#44522=ORIENTED_EDGE('',*,*,#35083,.T.) ;
#44523=ORIENTED_EDGE('',*,*,#35084,.T.) ;
#44524=ORIENTED_EDGE('',*,*,#35085,.T.) ;
#44525=ORIENTED_EDGE('',*,*,#35086,.T.) ;
#44526=ORIENTED_EDGE('',*,*,#35087,.T.) ;
#44527=ORIENTED_EDGE('',*,*,#35088,.T.) ;
#44528=ORIENTED_EDGE('',*,*,#35089,.T.) ;
#44529=ORIENTED_EDGE('',*,*,#35090,.T.) ;
#44530=ORIENTED_EDGE('',*,*,#35091,.T.) ;
#44531=ORIENTED_EDGE('',*,*,#35092,.T.) ;
#44532=ORIENTED_EDGE('',*,*,#35093,.T.) ;
#44533=ORIENTED_EDGE('',*,*,#35094,.T.) ;
#44534=ORIENTED_EDGE('',*,*,#35095,.T.) ;
#44535=ORIENTED_EDGE('',*,*,#35096,.T.) ;
#44536=ORIENTED_EDGE('',*,*,#35097,.T.) ;
#44537=ORIENTED_EDGE('',*,*,#35098,.T.) ;
#44538=ORIENTED_EDGE('',*,*,#35099,.T.) ;
#44539=ORIENTED_EDGE('',*,*,#35100,.T.) ;
#44540=ORIENTED_EDGE('',*,*,#34804,.F.) ;
#44541=ORIENTED_EDGE('',*,*,#35101,.T.) ;
#44542=ORIENTED_EDGE('',*,*,#34754,.T.) ;
#44543=ORIENTED_EDGE('',*,*,#35073,.F.) ;
#44544=ORIENTED_EDGE('',*,*,#35102,.T.) ;
#44545=ORIENTED_EDGE('',*,*,#35103,.T.) ;
#44546=ORIENTED_EDGE('',*,*,#35069,.T.) ;
#44547=ORIENTED_EDGE('',*,*,#35104,.T.) ;
#44548=ORIENTED_EDGE('',*,*,#35105,.T.) ;
#44549=ORIENTED_EDGE('',*,*,#35106,.T.) ;
#44550=ORIENTED_EDGE('',*,*,#35107,.T.) ;
#44551=ORIENTED_EDGE('',*,*,#35108,.T.) ;
#44552=ORIENTED_EDGE('',*,*,#35109,.T.) ;
#44553=ORIENTED_EDGE('',*,*,#35110,.T.) ;
#44554=ORIENTED_EDGE('',*,*,#35111,.T.) ;
#44555=ORIENTED_EDGE('',*,*,#35112,.T.) ;
#44556=ORIENTED_EDGE('',*,*,#35113,.T.) ;
#44557=ORIENTED_EDGE('',*,*,#35114,.T.) ;
#44558=ORIENTED_EDGE('',*,*,#35115,.T.) ;
#44559=ORIENTED_EDGE('',*,*,#35116,.T.) ;
#44560=ORIENTED_EDGE('',*,*,#35117,.T.) ;
#44561=ORIENTED_EDGE('',*,*,#35118,.T.) ;
#44562=ORIENTED_EDGE('',*,*,#35119,.T.) ;
#44563=ORIENTED_EDGE('',*,*,#35120,.T.) ;
#44564=ORIENTED_EDGE('',*,*,#35121,.T.) ;
#44565=ORIENTED_EDGE('',*,*,#35122,.T.) ;
#44566=ORIENTED_EDGE('',*,*,#35123,.T.) ;
#44567=ORIENTED_EDGE('',*,*,#35124,.T.) ;
#44568=ORIENTED_EDGE('',*,*,#35125,.T.) ;
#44569=ORIENTED_EDGE('',*,*,#35126,.T.) ;
#44570=ORIENTED_EDGE('',*,*,#35127,.T.) ;
#44571=ORIENTED_EDGE('',*,*,#35128,.T.) ;
#44572=ORIENTED_EDGE('',*,*,#35129,.T.) ;
#44573=ORIENTED_EDGE('',*,*,#35130,.T.) ;
#44574=ORIENTED_EDGE('',*,*,#35131,.T.) ;
#44575=ORIENTED_EDGE('',*,*,#35132,.T.) ;
#44576=ORIENTED_EDGE('',*,*,#35133,.T.) ;
#44577=ORIENTED_EDGE('',*,*,#35134,.T.) ;
#44578=ORIENTED_EDGE('',*,*,#35135,.T.) ;
#44579=ORIENTED_EDGE('',*,*,#35136,.T.) ;
#44580=ORIENTED_EDGE('',*,*,#35137,.T.) ;
#44581=ORIENTED_EDGE('',*,*,#35138,.T.) ;
#44582=ORIENTED_EDGE('',*,*,#35139,.T.) ;
#44583=ORIENTED_EDGE('',*,*,#35140,.T.) ;
#44584=ORIENTED_EDGE('',*,*,#35141,.T.) ;
#44585=ORIENTED_EDGE('',*,*,#35142,.T.) ;
#44586=ORIENTED_EDGE('',*,*,#35143,.T.) ;
#44587=ORIENTED_EDGE('',*,*,#35144,.T.) ;
#44588=ORIENTED_EDGE('',*,*,#35145,.T.) ;
#44589=ORIENTED_EDGE('',*,*,#35146,.T.) ;
#44590=ORIENTED_EDGE('',*,*,#35147,.T.) ;
#44591=ORIENTED_EDGE('',*,*,#35148,.T.) ;
#44592=ORIENTED_EDGE('',*,*,#35149,.T.) ;
#44593=ORIENTED_EDGE('',*,*,#35150,.T.) ;
#44594=ORIENTED_EDGE('',*,*,#35151,.T.) ;
#44595=ORIENTED_EDGE('',*,*,#35152,.T.) ;
#44596=ORIENTED_EDGE('',*,*,#35153,.T.) ;
#44597=ORIENTED_EDGE('',*,*,#35154,.T.) ;
#44598=ORIENTED_EDGE('',*,*,#35155,.T.) ;
#44599=ORIENTED_EDGE('',*,*,#35156,.T.) ;
#44600=ORIENTED_EDGE('',*,*,#35157,.T.) ;
#44601=ORIENTED_EDGE('',*,*,#35158,.T.) ;
#44602=ORIENTED_EDGE('',*,*,#35159,.T.) ;
#44603=ORIENTED_EDGE('',*,*,#35160,.T.) ;
#44604=ORIENTED_EDGE('',*,*,#35161,.T.) ;
#44605=ORIENTED_EDGE('',*,*,#35162,.T.) ;
#44606=ORIENTED_EDGE('',*,*,#35163,.T.) ;
#44607=ORIENTED_EDGE('',*,*,#35164,.T.) ;
#44608=ORIENTED_EDGE('',*,*,#35165,.T.) ;
#44609=ORIENTED_EDGE('',*,*,#35166,.T.) ;
#44610=ORIENTED_EDGE('',*,*,#35167,.T.) ;
#44611=ORIENTED_EDGE('',*,*,#35168,.T.) ;
#44612=ORIENTED_EDGE('',*,*,#35169,.T.) ;
#44613=ORIENTED_EDGE('',*,*,#35170,.T.) ;
#44614=ORIENTED_EDGE('',*,*,#35171,.T.) ;
#44615=ORIENTED_EDGE('',*,*,#35172,.T.) ;
#44616=ORIENTED_EDGE('',*,*,#35173,.T.) ;
#44617=ORIENTED_EDGE('',*,*,#35174,.T.) ;
#44618=ORIENTED_EDGE('',*,*,#35175,.T.) ;
#44619=ORIENTED_EDGE('',*,*,#35176,.T.) ;
#44620=ORIENTED_EDGE('',*,*,#35177,.T.) ;
#44621=ORIENTED_EDGE('',*,*,#35178,.T.) ;
#44622=ORIENTED_EDGE('',*,*,#35179,.T.) ;
#44623=ORIENTED_EDGE('',*,*,#35180,.T.) ;
#44624=ORIENTED_EDGE('',*,*,#35181,.T.) ;
#44625=ORIENTED_EDGE('',*,*,#35182,.T.) ;
#44626=ORIENTED_EDGE('',*,*,#35183,.T.) ;
#44627=ORIENTED_EDGE('',*,*,#35184,.T.) ;
#44628=ORIENTED_EDGE('',*,*,#35185,.T.) ;
#44629=ORIENTED_EDGE('',*,*,#35186,.T.) ;
#44630=ORIENTED_EDGE('',*,*,#35187,.T.) ;
#44631=ORIENTED_EDGE('',*,*,#35188,.T.) ;
#44632=ORIENTED_EDGE('',*,*,#35189,.T.) ;
#44633=ORIENTED_EDGE('',*,*,#35190,.T.) ;
#44634=ORIENTED_EDGE('',*,*,#35191,.T.) ;
#44635=ORIENTED_EDGE('',*,*,#35192,.T.) ;
#44636=ORIENTED_EDGE('',*,*,#35193,.T.) ;
#44637=ORIENTED_EDGE('',*,*,#35194,.T.) ;
#44638=ORIENTED_EDGE('',*,*,#35195,.T.) ;
#44639=ORIENTED_EDGE('',*,*,#35196,.T.) ;
#44640=ORIENTED_EDGE('',*,*,#35197,.T.) ;
#44641=ORIENTED_EDGE('',*,*,#35198,.T.) ;
#44642=ORIENTED_EDGE('',*,*,#35199,.T.) ;
#44643=ORIENTED_EDGE('',*,*,#35200,.T.) ;
#44644=ORIENTED_EDGE('',*,*,#35201,.T.) ;
#44645=ORIENTED_EDGE('',*,*,#35202,.T.) ;
#44646=ORIENTED_EDGE('',*,*,#35203,.T.) ;
#44647=ORIENTED_EDGE('',*,*,#35204,.T.) ;
#44648=ORIENTED_EDGE('',*,*,#35205,.T.) ;
#44649=ORIENTED_EDGE('',*,*,#35206,.T.) ;
#44650=ORIENTED_EDGE('',*,*,#35207,.T.) ;
#44651=ORIENTED_EDGE('',*,*,#35208,.T.) ;
#44652=ORIENTED_EDGE('',*,*,#35209,.T.) ;
#44653=ORIENTED_EDGE('',*,*,#35210,.T.) ;
#44654=ORIENTED_EDGE('',*,*,#35211,.T.) ;
#44655=ORIENTED_EDGE('',*,*,#35212,.T.) ;
#44656=ORIENTED_EDGE('',*,*,#35213,.T.) ;
#44657=ORIENTED_EDGE('',*,*,#35214,.T.) ;
#44658=ORIENTED_EDGE('',*,*,#35215,.T.) ;
#44659=ORIENTED_EDGE('',*,*,#35216,.T.) ;
#44660=ORIENTED_EDGE('',*,*,#35217,.T.) ;
#44661=ORIENTED_EDGE('',*,*,#35218,.T.) ;
#44662=ORIENTED_EDGE('',*,*,#35219,.T.) ;
#44663=ORIENTED_EDGE('',*,*,#35220,.T.) ;
#44664=ORIENTED_EDGE('',*,*,#35221,.T.) ;
#44665=ORIENTED_EDGE('',*,*,#35222,.T.) ;
#44666=ORIENTED_EDGE('',*,*,#35223,.T.) ;
#44667=ORIENTED_EDGE('',*,*,#35224,.T.) ;
#44668=ORIENTED_EDGE('',*,*,#35225,.T.) ;
#44669=ORIENTED_EDGE('',*,*,#35226,.T.) ;
#44670=ORIENTED_EDGE('',*,*,#35227,.T.) ;
#44671=ORIENTED_EDGE('',*,*,#35228,.T.) ;
#44672=ORIENTED_EDGE('',*,*,#35229,.T.) ;
#44673=ORIENTED_EDGE('',*,*,#35230,.T.) ;
#44674=ORIENTED_EDGE('',*,*,#35231,.T.) ;
#44675=ORIENTED_EDGE('',*,*,#35232,.T.) ;
#44676=ORIENTED_EDGE('',*,*,#35233,.T.) ;
#44677=ORIENTED_EDGE('',*,*,#35234,.T.) ;
#44678=ORIENTED_EDGE('',*,*,#35235,.T.) ;
#44679=ORIENTED_EDGE('',*,*,#35236,.T.) ;
#44680=ORIENTED_EDGE('',*,*,#35237,.T.) ;
#44681=ORIENTED_EDGE('',*,*,#35238,.T.) ;
#44682=ORIENTED_EDGE('',*,*,#35239,.T.) ;
#44683=ORIENTED_EDGE('',*,*,#35240,.T.) ;
#44684=ORIENTED_EDGE('',*,*,#35241,.T.) ;
#44685=ORIENTED_EDGE('',*,*,#35242,.T.) ;
#44686=ORIENTED_EDGE('',*,*,#35243,.T.) ;
#44687=ORIENTED_EDGE('',*,*,#35244,.T.) ;
#44688=ORIENTED_EDGE('',*,*,#35245,.T.) ;
#44689=ORIENTED_EDGE('',*,*,#35246,.T.) ;
#44690=ORIENTED_EDGE('',*,*,#35247,.T.) ;
#44691=ORIENTED_EDGE('',*,*,#35248,.T.) ;
#44692=ORIENTED_EDGE('',*,*,#35249,.T.) ;
#44693=ORIENTED_EDGE('',*,*,#35250,.T.) ;
#44694=ORIENTED_EDGE('',*,*,#35251,.T.) ;
#44695=ORIENTED_EDGE('',*,*,#35252,.T.) ;
#44696=ORIENTED_EDGE('',*,*,#35253,.T.) ;
#44697=ORIENTED_EDGE('',*,*,#35254,.T.) ;
#44698=ORIENTED_EDGE('',*,*,#35255,.T.) ;
#44699=ORIENTED_EDGE('',*,*,#35256,.T.) ;
#44700=ORIENTED_EDGE('',*,*,#35257,.T.) ;
#44701=ORIENTED_EDGE('',*,*,#35258,.T.) ;
#44702=ORIENTED_EDGE('',*,*,#35259,.T.) ;
#44703=ORIENTED_EDGE('',*,*,#35260,.T.) ;
#44704=ORIENTED_EDGE('',*,*,#35261,.T.) ;
#44705=ORIENTED_EDGE('',*,*,#35262,.T.) ;
#44706=ORIENTED_EDGE('',*,*,#35263,.T.) ;
#44707=ORIENTED_EDGE('',*,*,#35264,.T.) ;
#44708=ORIENTED_EDGE('',*,*,#35265,.T.) ;
#44709=ORIENTED_EDGE('',*,*,#35266,.T.) ;
#44710=ORIENTED_EDGE('',*,*,#35267,.T.) ;
#44711=ORIENTED_EDGE('',*,*,#35268,.T.) ;
#44712=ORIENTED_EDGE('',*,*,#35269,.T.) ;
#44713=ORIENTED_EDGE('',*,*,#35270,.T.) ;
#44714=ORIENTED_EDGE('',*,*,#35271,.T.) ;
#44715=ORIENTED_EDGE('',*,*,#35272,.T.) ;
#44716=ORIENTED_EDGE('',*,*,#35273,.T.) ;
#44717=ORIENTED_EDGE('',*,*,#35274,.T.) ;
#44718=ORIENTED_EDGE('',*,*,#35275,.T.) ;
#44719=ORIENTED_EDGE('',*,*,#35276,.T.) ;
#44720=ORIENTED_EDGE('',*,*,#35277,.T.) ;
#44721=ORIENTED_EDGE('',*,*,#35278,.T.) ;
#44722=ORIENTED_EDGE('',*,*,#35279,.T.) ;
#44723=ORIENTED_EDGE('',*,*,#35280,.T.) ;
#44724=ORIENTED_EDGE('',*,*,#35281,.T.) ;
#44725=ORIENTED_EDGE('',*,*,#35282,.T.) ;
#44726=ORIENTED_EDGE('',*,*,#35283,.T.) ;
#44727=ORIENTED_EDGE('',*,*,#35284,.T.) ;
#44728=ORIENTED_EDGE('',*,*,#35285,.T.) ;
#44729=ORIENTED_EDGE('',*,*,#35286,.T.) ;
#44730=ORIENTED_EDGE('',*,*,#35287,.T.) ;
#44731=ORIENTED_EDGE('',*,*,#35288,.T.) ;
#44732=ORIENTED_EDGE('',*,*,#35289,.T.) ;
#44733=ORIENTED_EDGE('',*,*,#35290,.T.) ;
#44734=ORIENTED_EDGE('',*,*,#35291,.T.) ;
#44735=ORIENTED_EDGE('',*,*,#35292,.T.) ;
#44736=ORIENTED_EDGE('',*,*,#35293,.T.) ;
#44737=ORIENTED_EDGE('',*,*,#35294,.T.) ;
#44738=ORIENTED_EDGE('',*,*,#35295,.T.) ;
#44739=ORIENTED_EDGE('',*,*,#35296,.T.) ;
#44740=ORIENTED_EDGE('',*,*,#35297,.F.) ;
#44741=ORIENTED_EDGE('',*,*,#34755,.F.) ;
#44742=ORIENTED_EDGE('',*,*,#35298,.F.) ;
#44743=ORIENTED_EDGE('',*,*,#35098,.F.) ;
#44744=ORIENTED_EDGE('',*,*,#35298,.T.) ;
#44745=ORIENTED_EDGE('',*,*,#35101,.F.) ;
#44746=ORIENTED_EDGE('',*,*,#35299,.F.) ;
#44747=ORIENTED_EDGE('',*,*,#35099,.F.) ;
#44748=ORIENTED_EDGE('',*,*,#35300,.F.) ;
#44749=ORIENTED_EDGE('',*,*,#35297,.T.) ;
#44750=ORIENTED_EDGE('',*,*,#35301,.F.) ;
#44751=ORIENTED_EDGE('',*,*,#35299,.T.) ;
#44752=ORIENTED_EDGE('',*,*,#34803,.F.) ;
#44753=ORIENTED_EDGE('',*,*,#35302,.F.) ;
#44754=ORIENTED_EDGE('',*,*,#35100,.F.) ;
#44755=ORIENTED_EDGE('',*,*,#35301,.T.) ;
#44756=ORIENTED_EDGE('',*,*,#35097,.F.) ;
#44757=ORIENTED_EDGE('',*,*,#35303,.F.) ;
#44758=ORIENTED_EDGE('',*,*,#35096,.F.) ;
#44759=ORIENTED_EDGE('',*,*,#35300,.T.) ;
#44760=ORIENTED_EDGE('',*,*,#35095,.F.) ;
#44761=ORIENTED_EDGE('',*,*,#35304,.F.) ;
#44762=ORIENTED_EDGE('',*,*,#34756,.F.) ;
#44763=ORIENTED_EDGE('',*,*,#35303,.T.) ;
#44764=ORIENTED_EDGE('',*,*,#35302,.T.) ;
#44765=ORIENTED_EDGE('',*,*,#35305,.F.) ;
#44766=ORIENTED_EDGE('',*,*,#35306,.F.) ;
#44767=ORIENTED_EDGE('',*,*,#35304,.T.) ;
#44768=ORIENTED_EDGE('',*,*,#35307,.F.) ;
#44769=ORIENTED_EDGE('',*,*,#35305,.T.) ;
#44770=ORIENTED_EDGE('',*,*,#34802,.F.) ;
#44771=ORIENTED_EDGE('',*,*,#35308,.F.) ;
#44772=ORIENTED_EDGE('',*,*,#35093,.F.) ;
#44773=ORIENTED_EDGE('',*,*,#35307,.T.) ;
#44774=ORIENTED_EDGE('',*,*,#35094,.F.) ;
#44775=ORIENTED_EDGE('',*,*,#35309,.F.) ;
#44776=ORIENTED_EDGE('',*,*,#35092,.F.) ;
#44777=ORIENTED_EDGE('',*,*,#35306,.T.) ;
#44778=ORIENTED_EDGE('',*,*,#35091,.F.) ;
#44779=ORIENTED_EDGE('',*,*,#35310,.F.) ;
#44780=ORIENTED_EDGE('',*,*,#34757,.F.) ;
#44781=ORIENTED_EDGE('',*,*,#35309,.T.) ;
#44782=ORIENTED_EDGE('',*,*,#35308,.T.) ;
#44783=ORIENTED_EDGE('',*,*,#35311,.F.) ;
#44784=ORIENTED_EDGE('',*,*,#34758,.T.) ;
#44785=ORIENTED_EDGE('',*,*,#35310,.T.) ;
#44786=ORIENTED_EDGE('',*,*,#35312,.F.) ;
#44787=ORIENTED_EDGE('',*,*,#35313,.F.) ;
#44788=ORIENTED_EDGE('',*,*,#35311,.T.) ;
#44789=ORIENTED_EDGE('',*,*,#34801,.F.) ;
#44790=ORIENTED_EDGE('',*,*,#35314,.F.) ;
#44791=ORIENTED_EDGE('',*,*,#35089,.F.) ;
#44792=ORIENTED_EDGE('',*,*,#35312,.T.) ;
#44793=ORIENTED_EDGE('',*,*,#35090,.F.) ;
#44794=ORIENTED_EDGE('',*,*,#35315,.F.) ;
#44795=ORIENTED_EDGE('',*,*,#35088,.F.) ;
#44796=ORIENTED_EDGE('',*,*,#35313,.T.) ;
#44797=ORIENTED_EDGE('',*,*,#35087,.F.) ;
#44798=ORIENTED_EDGE('',*,*,#35316,.F.) ;
#44799=ORIENTED_EDGE('',*,*,#34759,.F.) ;
#44800=ORIENTED_EDGE('',*,*,#35314,.T.) ;
#44801=ORIENTED_EDGE('',*,*,#34800,.T.) ;
#44802=ORIENTED_EDGE('',*,*,#35317,.F.) ;
#44803=ORIENTED_EDGE('',*,*,#35315,.T.) ;
#44804=ORIENTED_EDGE('',*,*,#35318,.F.) ;
#44805=ORIENTED_EDGE('',*,*,#35316,.T.) ;
#44806=ORIENTED_EDGE('',*,*,#35319,.F.) ;
#44807=ORIENTED_EDGE('',*,*,#35317,.T.) ;
#44808=ORIENTED_EDGE('',*,*,#34799,.F.) ;
#44809=ORIENTED_EDGE('',*,*,#35320,.F.) ;
#44810=ORIENTED_EDGE('',*,*,#35085,.F.) ;
#44811=ORIENTED_EDGE('',*,*,#35319,.T.) ;
#44812=ORIENTED_EDGE('',*,*,#35086,.F.) ;
#44813=ORIENTED_EDGE('',*,*,#35321,.F.) ;
#44814=ORIENTED_EDGE('',*,*,#35084,.F.) ;
#44815=ORIENTED_EDGE('',*,*,#35318,.T.) ;
#44816=ORIENTED_EDGE('',*,*,#35083,.F.) ;
#44817=ORIENTED_EDGE('',*,*,#35322,.F.) ;
#44818=ORIENTED_EDGE('',*,*,#34760,.F.) ;
#44819=ORIENTED_EDGE('',*,*,#35321,.T.) ;
#44820=ORIENTED_EDGE('',*,*,#35320,.T.) ;
#44821=ORIENTED_EDGE('',*,*,#35323,.F.) ;
#44822=ORIENTED_EDGE('',*,*,#35324,.F.) ;
#44823=ORIENTED_EDGE('',*,*,#35322,.T.) ;
#44824=ORIENTED_EDGE('',*,*,#35325,.F.) ;
#44825=ORIENTED_EDGE('',*,*,#35323,.T.) ;
#44826=ORIENTED_EDGE('',*,*,#34798,.F.) ;
#44827=ORIENTED_EDGE('',*,*,#35326,.F.) ;
#44828=ORIENTED_EDGE('',*,*,#35081,.F.) ;
#44829=ORIENTED_EDGE('',*,*,#35325,.T.) ;
#44830=ORIENTED_EDGE('',*,*,#35082,.F.) ;
#44831=ORIENTED_EDGE('',*,*,#35327,.F.) ;
#44832=ORIENTED_EDGE('',*,*,#35080,.F.) ;
#44833=ORIENTED_EDGE('',*,*,#35324,.T.) ;
#44834=ORIENTED_EDGE('',*,*,#35079,.F.) ;
#44835=ORIENTED_EDGE('',*,*,#35328,.F.) ;
#44836=ORIENTED_EDGE('',*,*,#34761,.F.) ;
#44837=ORIENTED_EDGE('',*,*,#35329,.F.) ;
#44838=ORIENTED_EDGE('',*,*,#34846,.F.) ;
#44839=ORIENTED_EDGE('',*,*,#35330,.F.) ;
#44840=ORIENTED_EDGE('',*,*,#35040,.F.) ;
#44841=ORIENTED_EDGE('',*,*,#35327,.T.) ;
#44842=ORIENTED_EDGE('',*,*,#35326,.T.) ;
#44843=ORIENTED_EDGE('',*,*,#35331,.F.) ;
#44844=ORIENTED_EDGE('',*,*,#34751,.T.) ;
#44845=ORIENTED_EDGE('',*,*,#35328,.T.) ;
#44846=ORIENTED_EDGE('',*,*,#35332,.F.) ;
#44847=ORIENTED_EDGE('',*,*,#35333,.F.) ;
#44848=ORIENTED_EDGE('',*,*,#35334,.F.) ;
#44849=ORIENTED_EDGE('',*,*,#35330,.T.) ;
#44850=ORIENTED_EDGE('',*,*,#35335,.F.) ;
#44851=ORIENTED_EDGE('',*,*,#35329,.T.) ;
#44852=ORIENTED_EDGE('',*,*,#35043,.F.) ;
#44853=ORIENTED_EDGE('',*,*,#35336,.F.) ;
#44854=ORIENTED_EDGE('',*,*,#35047,.F.) ;
#44855=ORIENTED_EDGE('',*,*,#35331,.T.) ;
#44856=ORIENTED_EDGE('',*,*,#34797,.F.) ;
#44857=ORIENTED_EDGE('',*,*,#35337,.F.) ;
#44858=ORIENTED_EDGE('',*,*,#35077,.F.) ;
#44859=ORIENTED_EDGE('',*,*,#35332,.T.) ;
#44860=ORIENTED_EDGE('',*,*,#35078,.F.) ;
#44861=ORIENTED_EDGE('',*,*,#35338,.F.) ;
#44862=ORIENTED_EDGE('',*,*,#35102,.F.) ;
#44863=ORIENTED_EDGE('',*,*,#35333,.T.) ;
#44864=ORIENTED_EDGE('',*,*,#35104,.F.) ;
#44865=ORIENTED_EDGE('',*,*,#35339,.F.) ;
#44866=ORIENTED_EDGE('',*,*,#34752,.F.) ;
#44867=ORIENTED_EDGE('',*,*,#35335,.T.) ;
#44868=ORIENTED_EDGE('',*,*,#34845,.F.) ;
#44869=ORIENTED_EDGE('',*,*,#35340,.F.) ;
#44870=ORIENTED_EDGE('',*,*,#35023,.F.) ;
#44871=ORIENTED_EDGE('',*,*,#35334,.T.) ;
#44872=ORIENTED_EDGE('',*,*,#35022,.F.) ;
#44873=ORIENTED_EDGE('',*,*,#35341,.F.) ;
#44874=ORIENTED_EDGE('',*,*,#35041,.F.) ;
#44875=ORIENTED_EDGE('',*,*,#35336,.T.) ;
#44876=ORIENTED_EDGE('',*,*,#35042,.F.) ;
#44877=ORIENTED_EDGE('',*,*,#35342,.F.) ;
#44878=ORIENTED_EDGE('',*,*,#34908,.F.) ;
#44879=ORIENTED_EDGE('',*,*,#35337,.T.) ;
#44880=ORIENTED_EDGE('',*,*,#34796,.T.) ;
#44881=ORIENTED_EDGE('',*,*,#35343,.F.) ;
#44882=ORIENTED_EDGE('',*,*,#35338,.T.) ;
#44883=ORIENTED_EDGE('',*,*,#35339,.T.) ;
#44884=ORIENTED_EDGE('',*,*,#35071,.F.) ;
#44885=ORIENTED_EDGE('',*,*,#35344,.F.) ;
#44886=ORIENTED_EDGE('',*,*,#35075,.F.) ;
#44887=ORIENTED_EDGE('',*,*,#35345,.F.) ;
#44888=ORIENTED_EDGE('',*,*,#35340,.T.) ;
#44889=ORIENTED_EDGE('',*,*,#35346,.F.) ;
#44890=ORIENTED_EDGE('',*,*,#35342,.T.) ;
#44891=ORIENTED_EDGE('',*,*,#35341,.T.) ;
#44892=ORIENTED_EDGE('',*,*,#35347,.F.) ;
#44893=ORIENTED_EDGE('',*,*,#35343,.T.) ;
#44894=ORIENTED_EDGE('',*,*,#34795,.F.) ;
#44895=ORIENTED_EDGE('',*,*,#35348,.F.) ;
#44896=ORIENTED_EDGE('',*,*,#35103,.F.) ;
#44897=ORIENTED_EDGE('',*,*,#35344,.T.) ;
#44898=ORIENTED_EDGE('',*,*,#34994,.F.) ;
#44899=ORIENTED_EDGE('',*,*,#35349,.F.) ;
#44900=ORIENTED_EDGE('',*,*,#34976,.F.) ;
#44901=ORIENTED_EDGE('',*,*,#35346,.T.) ;
#44902=ORIENTED_EDGE('',*,*,#34844,.F.) ;
#44903=ORIENTED_EDGE('',*,*,#35350,.F.) ;
#44904=ORIENTED_EDGE('',*,*,#35026,.F.) ;
#44905=ORIENTED_EDGE('',*,*,#35345,.T.) ;
#44906=ORIENTED_EDGE('',*,*,#35025,.F.) ;
#44907=ORIENTED_EDGE('',*,*,#35351,.F.) ;
#44908=ORIENTED_EDGE('',*,*,#35020,.F.) ;
#44909=ORIENTED_EDGE('',*,*,#35347,.T.) ;
#44910=ORIENTED_EDGE('',*,*,#35021,.F.) ;
#44911=ORIENTED_EDGE('',*,*,#35352,.F.) ;
#44912=ORIENTED_EDGE('',*,*,#34909,.F.) ;
#44913=ORIENTED_EDGE('',*,*,#35348,.T.) ;
#44914=ORIENTED_EDGE('',*,*,#35076,.F.) ;
#44915=ORIENTED_EDGE('',*,*,#35353,.F.) ;
#44916=ORIENTED_EDGE('',*,*,#35070,.F.) ;
#44917=ORIENTED_EDGE('',*,*,#34977,.T.) ;
#44918=ORIENTED_EDGE('',*,*,#35349,.T.) ;
#44919=ORIENTED_EDGE('',*,*,#35354,.F.) ;
#44920=ORIENTED_EDGE('',*,*,#35355,.F.) ;
#44921=ORIENTED_EDGE('',*,*,#35350,.T.) ;
#44922=ORIENTED_EDGE('',*,*,#34843,.T.) ;
#44923=ORIENTED_EDGE('',*,*,#35356,.F.) ;
#44924=ORIENTED_EDGE('',*,*,#35357,.F.) ;
#44925=ORIENTED_EDGE('',*,*,#35352,.T.) ;
#44926=ORIENTED_EDGE('',*,*,#35351,.T.) ;
#44927=ORIENTED_EDGE('',*,*,#35358,.F.) ;
#44928=ORIENTED_EDGE('',*,*,#35353,.T.) ;
#44929=ORIENTED_EDGE('',*,*,#34988,.F.) ;
#44930=ORIENTED_EDGE('',*,*,#35359,.F.) ;
#44931=ORIENTED_EDGE('',*,*,#34992,.F.) ;
#44932=ORIENTED_EDGE('',*,*,#35354,.T.) ;
#44933=ORIENTED_EDGE('',*,*,#34993,.F.) ;
#44934=ORIENTED_EDGE('',*,*,#35360,.F.) ;
#44935=ORIENTED_EDGE('',*,*,#35006,.F.) ;
#44936=ORIENTED_EDGE('',*,*,#35355,.T.) ;
#44937=ORIENTED_EDGE('',*,*,#35005,.F.) ;
#44938=ORIENTED_EDGE('',*,*,#35361,.F.) ;
#44939=ORIENTED_EDGE('',*,*,#34978,.F.) ;
#44940=ORIENTED_EDGE('',*,*,#35356,.T.) ;
#44941=ORIENTED_EDGE('',*,*,#34842,.F.) ;
#44942=ORIENTED_EDGE('',*,*,#35362,.F.) ;
#44943=ORIENTED_EDGE('',*,*,#35030,.F.) ;
#44944=ORIENTED_EDGE('',*,*,#35357,.T.) ;
#44945=ORIENTED_EDGE('',*,*,#35029,.F.) ;
#44946=ORIENTED_EDGE('',*,*,#35363,.F.) ;
#44947=ORIENTED_EDGE('',*,*,#35027,.F.) ;
#44948=ORIENTED_EDGE('',*,*,#35358,.T.) ;
#44949=ORIENTED_EDGE('',*,*,#35024,.F.) ;
#44950=ORIENTED_EDGE('',*,*,#35364,.F.) ;
#44951=ORIENTED_EDGE('',*,*,#34910,.F.) ;
#44952=ORIENTED_EDGE('',*,*,#35359,.T.) ;
#44953=ORIENTED_EDGE('',*,*,#34987,.T.) ;
#44954=ORIENTED_EDGE('',*,*,#35365,.F.) ;
#44955=ORIENTED_EDGE('',*,*,#35360,.T.) ;
#44956=ORIENTED_EDGE('',*,*,#35366,.F.) ;
#44957=ORIENTED_EDGE('',*,*,#35361,.T.) ;
#44958=ORIENTED_EDGE('',*,*,#35367,.F.) ;
#44959=ORIENTED_EDGE('',*,*,#35368,.F.) ;
#44960=ORIENTED_EDGE('',*,*,#35362,.T.) ;
#44961=ORIENTED_EDGE('',*,*,#35369,.F.) ;
#44962=ORIENTED_EDGE('',*,*,#35364,.T.) ;
#44963=ORIENTED_EDGE('',*,*,#35363,.T.) ;
#44964=ORIENTED_EDGE('',*,*,#35370,.F.) ;
#44965=ORIENTED_EDGE('',*,*,#34911,.T.) ;
#44966=ORIENTED_EDGE('',*,*,#35365,.T.) ;
#44967=ORIENTED_EDGE('',*,*,#34986,.F.) ;
#44968=ORIENTED_EDGE('',*,*,#35371,.F.) ;
#44969=ORIENTED_EDGE('',*,*,#35003,.F.) ;
#44970=ORIENTED_EDGE('',*,*,#35367,.T.) ;
#44971=ORIENTED_EDGE('',*,*,#35004,.F.) ;
#44972=ORIENTED_EDGE('',*,*,#35372,.F.) ;
#44973=ORIENTED_EDGE('',*,*,#35002,.F.) ;
#44974=ORIENTED_EDGE('',*,*,#35366,.T.) ;
#44975=ORIENTED_EDGE('',*,*,#35001,.F.) ;
#44976=ORIENTED_EDGE('',*,*,#35373,.F.) ;
#44977=ORIENTED_EDGE('',*,*,#34979,.F.) ;
#44978=ORIENTED_EDGE('',*,*,#35369,.T.) ;
#44979=ORIENTED_EDGE('',*,*,#34841,.F.) ;
#44980=ORIENTED_EDGE('',*,*,#35374,.F.) ;
#44981=ORIENTED_EDGE('',*,*,#35034,.F.) ;
#44982=ORIENTED_EDGE('',*,*,#35368,.T.) ;
#44983=ORIENTED_EDGE('',*,*,#35033,.F.) ;
#44984=ORIENTED_EDGE('',*,*,#35375,.F.) ;
#44985=ORIENTED_EDGE('',*,*,#35031,.F.) ;
#44986=ORIENTED_EDGE('',*,*,#35370,.T.) ;
#44987=ORIENTED_EDGE('',*,*,#35028,.F.) ;
#44988=ORIENTED_EDGE('',*,*,#35376,.F.) ;
#44989=ORIENTED_EDGE('',*,*,#34912,.F.) ;
#44990=ORIENTED_EDGE('',*,*,#35372,.T.) ;
#44991=ORIENTED_EDGE('',*,*,#35371,.T.) ;
#44992=ORIENTED_EDGE('',*,*,#35377,.F.) ;
#44993=ORIENTED_EDGE('',*,*,#35378,.F.) ;
#44994=ORIENTED_EDGE('',*,*,#35373,.T.) ;
#44995=ORIENTED_EDGE('',*,*,#35379,.F.) ;
#44996=ORIENTED_EDGE('',*,*,#35380,.F.) ;
#44997=ORIENTED_EDGE('',*,*,#35018,.F.) ;
#44998=ORIENTED_EDGE('',*,*,#35381,.F.) ;
#44999=ORIENTED_EDGE('',*,*,#35013,.F.) ;
#45000=ORIENTED_EDGE('',*,*,#35382,.F.) ;
#45001=ORIENTED_EDGE('',*,*,#35374,.T.) ;
#45002=ORIENTED_EDGE('',*,*,#35383,.F.) ;
#45003=ORIENTED_EDGE('',*,*,#35376,.T.) ;
#45004=ORIENTED_EDGE('',*,*,#35375,.T.) ;
#45005=ORIENTED_EDGE('',*,*,#35384,.F.) ;
#45006=ORIENTED_EDGE('',*,*,#35377,.T.) ;
#45007=ORIENTED_EDGE('',*,*,#34985,.F.) ;
#45008=ORIENTED_EDGE('',*,*,#35385,.F.) ;
#45009=ORIENTED_EDGE('',*,*,#34999,.F.) ;
#45010=ORIENTED_EDGE('',*,*,#35379,.T.) ;
#45011=ORIENTED_EDGE('',*,*,#35000,.F.) ;
#45012=ORIENTED_EDGE('',*,*,#35386,.F.) ;
#45013=ORIENTED_EDGE('',*,*,#35010,.F.) ;
#45014=ORIENTED_EDGE('',*,*,#35378,.T.) ;
#45015=ORIENTED_EDGE('',*,*,#35009,.F.) ;
#45016=ORIENTED_EDGE('',*,*,#35387,.F.) ;
#45017=ORIENTED_EDGE('',*,*,#34980,.F.) ;
#45018=ORIENTED_EDGE('',*,*,#35381,.T.) ;
#45019=ORIENTED_EDGE('',*,*,#34972,.F.) ;
#45020=ORIENTED_EDGE('',*,*,#35388,.F.) ;
#45021=ORIENTED_EDGE('',*,*,#34998,.F.) ;
#45022=ORIENTED_EDGE('',*,*,#35380,.T.) ;
#45023=ORIENTED_EDGE('',*,*,#35046,.F.) ;
#45024=ORIENTED_EDGE('',*,*,#35389,.F.) ;
#45025=ORIENTED_EDGE('',*,*,#34838,.F.) ;
#45026=ORIENTED_EDGE('',*,*,#35383,.T.) ;
#45027=ORIENTED_EDGE('',*,*,#34840,.F.) ;
#45028=ORIENTED_EDGE('',*,*,#35390,.F.) ;
#45029=ORIENTED_EDGE('',*,*,#35038,.F.) ;
#45030=ORIENTED_EDGE('',*,*,#35382,.T.) ;
#45031=ORIENTED_EDGE('',*,*,#35037,.F.) ;
#45032=ORIENTED_EDGE('',*,*,#35391,.F.) ;
#45033=ORIENTED_EDGE('',*,*,#35035,.F.) ;
#45034=ORIENTED_EDGE('',*,*,#35384,.T.) ;
#45035=ORIENTED_EDGE('',*,*,#35032,.F.) ;
#45036=ORIENTED_EDGE('',*,*,#35392,.F.) ;
#45037=ORIENTED_EDGE('',*,*,#34913,.F.) ;
#45038=ORIENTED_EDGE('',*,*,#35386,.T.) ;
#45039=ORIENTED_EDGE('',*,*,#35385,.T.) ;
#45040=ORIENTED_EDGE('',*,*,#35393,.F.) ;
#45041=ORIENTED_EDGE('',*,*,#34971,.T.) ;
#45042=ORIENTED_EDGE('',*,*,#35387,.T.) ;
#45043=ORIENTED_EDGE('',*,*,#35394,.F.) ;
#45044=ORIENTED_EDGE('',*,*,#35388,.T.) ;
#45045=ORIENTED_EDGE('',*,*,#34839,.T.) ;
#45046=ORIENTED_EDGE('',*,*,#35389,.T.) ;
#45047=ORIENTED_EDGE('',*,*,#35395,.F.) ;
#45048=ORIENTED_EDGE('',*,*,#35390,.T.) ;
#45049=ORIENTED_EDGE('',*,*,#35392,.T.) ;
#45050=ORIENTED_EDGE('',*,*,#35391,.T.) ;
#45051=ORIENTED_EDGE('',*,*,#35396,.F.) ;
#45052=ORIENTED_EDGE('',*,*,#35393,.T.) ;
#45053=ORIENTED_EDGE('',*,*,#34984,.F.) ;
#45054=ORIENTED_EDGE('',*,*,#35397,.F.) ;
#45055=ORIENTED_EDGE('',*,*,#35007,.F.) ;
#45056=ORIENTED_EDGE('',*,*,#35394,.T.) ;
#45057=ORIENTED_EDGE('',*,*,#35008,.F.) ;
#45058=ORIENTED_EDGE('',*,*,#35398,.F.) ;
#45059=ORIENTED_EDGE('',*,*,#34995,.F.) ;
#45060=ORIENTED_EDGE('',*,*,#35395,.T.) ;
#45061=ORIENTED_EDGE('',*,*,#35045,.F.) ;
#45062=ORIENTED_EDGE('',*,*,#35399,.F.) ;
#45063=ORIENTED_EDGE('',*,*,#35039,.F.) ;
#45064=ORIENTED_EDGE('',*,*,#35396,.T.) ;
#45065=ORIENTED_EDGE('',*,*,#35036,.F.) ;
#45066=ORIENTED_EDGE('',*,*,#35400,.F.) ;
#45067=ORIENTED_EDGE('',*,*,#34914,.F.) ;
#45068=ORIENTED_EDGE('',*,*,#35397,.T.) ;
#45069=ORIENTED_EDGE('',*,*,#34983,.T.) ;
#45070=ORIENTED_EDGE('',*,*,#35401,.F.) ;
#45071=ORIENTED_EDGE('',*,*,#35398,.T.) ;
#45072=ORIENTED_EDGE('',*,*,#35400,.T.) ;
#45073=ORIENTED_EDGE('',*,*,#35399,.T.) ;
#45074=ORIENTED_EDGE('',*,*,#35402,.F.) ;
#45075=ORIENTED_EDGE('',*,*,#34904,.T.) ;
#45076=ORIENTED_EDGE('',*,*,#35401,.T.) ;
#45077=ORIENTED_EDGE('',*,*,#34982,.F.) ;
#45078=ORIENTED_EDGE('',*,*,#35403,.F.) ;
#45079=ORIENTED_EDGE('',*,*,#34996,.F.) ;
#45080=ORIENTED_EDGE('',*,*,#35402,.T.) ;
#45081=ORIENTED_EDGE('',*,*,#35044,.F.) ;
#45082=ORIENTED_EDGE('',*,*,#35404,.F.) ;
#45083=ORIENTED_EDGE('',*,*,#34905,.F.) ;
#45084=ORIENTED_EDGE('',*,*,#35403,.T.) ;
#45085=ORIENTED_EDGE('',*,*,#35019,.F.) ;
#45086=ORIENTED_EDGE('',*,*,#35404,.T.) ;
#45087=ORIENTED_EDGE('',*,*,#35011,.F.) ;
#45088=ORIENTED_EDGE('',*,*,#35405,.F.) ;
#45089=ORIENTED_EDGE('',*,*,#34777,.F.) ;
#45090=ORIENTED_EDGE('',*,*,#35406,.F.) ;
#45091=ORIENTED_EDGE('',*,*,#35279,.F.) ;
#45092=ORIENTED_EDGE('',*,*,#34770,.T.) ;
#45093=ORIENTED_EDGE('',*,*,#35405,.T.) ;
#45094=ORIENTED_EDGE('',*,*,#35407,.F.) ;
#45095=ORIENTED_EDGE('',*,*,#35408,.F.) ;
#45096=ORIENTED_EDGE('',*,*,#35406,.T.) ;
#45097=ORIENTED_EDGE('',*,*,#34776,.T.) ;
#45098=ORIENTED_EDGE('',*,*,#35409,.F.) ;
#45099=ORIENTED_EDGE('',*,*,#35410,.F.) ;
#45100=ORIENTED_EDGE('',*,*,#35407,.T.) ;
#45101=ORIENTED_EDGE('',*,*,#35278,.F.) ;
#45102=ORIENTED_EDGE('',*,*,#35411,.F.) ;
#45103=ORIENTED_EDGE('',*,*,#35266,.F.) ;
#45104=ORIENTED_EDGE('',*,*,#35408,.T.) ;
#45105=ORIENTED_EDGE('',*,*,#35265,.F.) ;
#45106=ORIENTED_EDGE('',*,*,#35412,.F.) ;
#45107=ORIENTED_EDGE('',*,*,#34771,.F.) ;
#45108=ORIENTED_EDGE('',*,*,#35413,.F.) ;
#45109=ORIENTED_EDGE('',*,*,#34773,.F.) ;
#45110=ORIENTED_EDGE('',*,*,#35414,.F.) ;
#45111=ORIENTED_EDGE('',*,*,#35269,.F.) ;
#45112=ORIENTED_EDGE('',*,*,#35409,.T.) ;
#45113=ORIENTED_EDGE('',*,*,#34775,.F.) ;
#45114=ORIENTED_EDGE('',*,*,#35415,.F.) ;
#45115=ORIENTED_EDGE('',*,*,#35273,.F.) ;
#45116=ORIENTED_EDGE('',*,*,#35410,.T.) ;
#45117=ORIENTED_EDGE('',*,*,#35276,.F.) ;
#45118=ORIENTED_EDGE('',*,*,#35416,.F.) ;
#45119=ORIENTED_EDGE('',*,*,#35280,.F.) ;
#45120=ORIENTED_EDGE('',*,*,#35417,.F.) ;
#45121=ORIENTED_EDGE('',*,*,#34816,.F.) ;
#45122=ORIENTED_EDGE('',*,*,#35418,.F.) ;
#45123=ORIENTED_EDGE('',*,*,#35277,.F.) ;
#45124=ORIENTED_EDGE('',*,*,#35418,.T.) ;
#45125=ORIENTED_EDGE('',*,*,#34815,.T.) ;
#45126=ORIENTED_EDGE('',*,*,#35419,.F.) ;
#45127=ORIENTED_EDGE('',*,*,#35411,.T.) ;
#45128=ORIENTED_EDGE('',*,*,#34772,.T.) ;
#45129=ORIENTED_EDGE('',*,*,#35412,.T.) ;
#45130=ORIENTED_EDGE('',*,*,#35420,.F.) ;
#45131=ORIENTED_EDGE('',*,*,#35414,.T.) ;
#45132=ORIENTED_EDGE('',*,*,#34774,.T.) ;
#45133=ORIENTED_EDGE('',*,*,#35413,.T.) ;
#45134=ORIENTED_EDGE('',*,*,#35421,.F.) ;
#45135=ORIENTED_EDGE('',*,*,#35415,.T.) ;
#45136=ORIENTED_EDGE('',*,*,#35417,.T.) ;
#45137=ORIENTED_EDGE('',*,*,#35416,.T.) ;
#45138=ORIENTED_EDGE('',*,*,#35422,.F.) ;
#45139=ORIENTED_EDGE('',*,*,#34817,.T.) ;
#45140=ORIENTED_EDGE('',*,*,#35419,.T.) ;
#45141=ORIENTED_EDGE('',*,*,#34814,.F.) ;
#45142=ORIENTED_EDGE('',*,*,#35423,.F.) ;
#45143=ORIENTED_EDGE('',*,*,#35267,.F.) ;
#45144=ORIENTED_EDGE('',*,*,#35420,.T.) ;
#45145=ORIENTED_EDGE('',*,*,#35268,.F.) ;
#45146=ORIENTED_EDGE('',*,*,#35424,.F.) ;
#45147=ORIENTED_EDGE('',*,*,#35270,.F.) ;
#45148=ORIENTED_EDGE('',*,*,#35421,.T.) ;
#45149=ORIENTED_EDGE('',*,*,#35272,.F.) ;
#45150=ORIENTED_EDGE('',*,*,#35425,.F.) ;
#45151=ORIENTED_EDGE('',*,*,#35274,.F.) ;
#45152=ORIENTED_EDGE('',*,*,#35422,.T.) ;
#45153=ORIENTED_EDGE('',*,*,#35275,.F.) ;
#45154=ORIENTED_EDGE('',*,*,#35426,.F.) ;
#45155=ORIENTED_EDGE('',*,*,#34818,.F.) ;
#45156=ORIENTED_EDGE('',*,*,#35423,.T.) ;
#45157=ORIENTED_EDGE('',*,*,#34813,.T.) ;
#45158=ORIENTED_EDGE('',*,*,#35427,.F.) ;
#45159=ORIENTED_EDGE('',*,*,#35424,.T.) ;
#45160=ORIENTED_EDGE('',*,*,#35426,.T.) ;
#45161=ORIENTED_EDGE('',*,*,#35425,.T.) ;
#45162=ORIENTED_EDGE('',*,*,#35428,.F.) ;
#45163=ORIENTED_EDGE('',*,*,#34819,.T.) ;
#45164=ORIENTED_EDGE('',*,*,#35427,.T.) ;
#45165=ORIENTED_EDGE('',*,*,#34820,.F.) ;
#45166=ORIENTED_EDGE('',*,*,#35428,.T.) ;
#45167=ORIENTED_EDGE('',*,*,#35271,.F.) ;
#45168=ORIENTED_EDGE('',*,*,#35429,.F.) ;
#45169=ORIENTED_EDGE('',*,*,#34785,.F.) ;
#45170=ORIENTED_EDGE('',*,*,#35430,.F.) ;
#45171=ORIENTED_EDGE('',*,*,#35251,.F.) ;
#45172=ORIENTED_EDGE('',*,*,#34778,.T.) ;
#45173=ORIENTED_EDGE('',*,*,#35429,.T.) ;
#45174=ORIENTED_EDGE('',*,*,#35431,.F.) ;
#45175=ORIENTED_EDGE('',*,*,#35432,.F.) ;
#45176=ORIENTED_EDGE('',*,*,#35430,.T.) ;
#45177=ORIENTED_EDGE('',*,*,#34784,.T.) ;
#45178=ORIENTED_EDGE('',*,*,#35433,.F.) ;
#45179=ORIENTED_EDGE('',*,*,#35434,.F.) ;
#45180=ORIENTED_EDGE('',*,*,#35431,.T.) ;
#45181=ORIENTED_EDGE('',*,*,#35250,.F.) ;
#45182=ORIENTED_EDGE('',*,*,#35435,.F.) ;
#45183=ORIENTED_EDGE('',*,*,#35254,.F.) ;
#45184=ORIENTED_EDGE('',*,*,#35432,.T.) ;
#45185=ORIENTED_EDGE('',*,*,#35253,.F.) ;
#45186=ORIENTED_EDGE('',*,*,#35436,.F.) ;
#45187=ORIENTED_EDGE('',*,*,#34779,.F.) ;
#45188=ORIENTED_EDGE('',*,*,#35437,.F.) ;
#45189=ORIENTED_EDGE('',*,*,#34781,.F.) ;
#45190=ORIENTED_EDGE('',*,*,#35438,.F.) ;
#45191=ORIENTED_EDGE('',*,*,#35257,.F.) ;
#45192=ORIENTED_EDGE('',*,*,#35433,.T.) ;
#45193=ORIENTED_EDGE('',*,*,#34783,.F.) ;
#45194=ORIENTED_EDGE('',*,*,#35439,.F.) ;
#45195=ORIENTED_EDGE('',*,*,#35261,.F.) ;
#45196=ORIENTED_EDGE('',*,*,#35434,.T.) ;
#45197=ORIENTED_EDGE('',*,*,#35264,.F.) ;
#45198=ORIENTED_EDGE('',*,*,#35440,.F.) ;
#45199=ORIENTED_EDGE('',*,*,#35252,.F.) ;
#45200=ORIENTED_EDGE('',*,*,#35441,.F.) ;
#45201=ORIENTED_EDGE('',*,*,#34824,.F.) ;
#45202=ORIENTED_EDGE('',*,*,#35442,.F.) ;
#45203=ORIENTED_EDGE('',*,*,#35249,.F.) ;
#45204=ORIENTED_EDGE('',*,*,#35442,.T.) ;
#45205=ORIENTED_EDGE('',*,*,#34823,.T.) ;
#45206=ORIENTED_EDGE('',*,*,#35443,.F.) ;
#45207=ORIENTED_EDGE('',*,*,#35435,.T.) ;
#45208=ORIENTED_EDGE('',*,*,#34780,.T.) ;
#45209=ORIENTED_EDGE('',*,*,#35436,.T.) ;
#45210=ORIENTED_EDGE('',*,*,#35444,.F.) ;
#45211=ORIENTED_EDGE('',*,*,#35438,.T.) ;
#45212=ORIENTED_EDGE('',*,*,#34782,.T.) ;
#45213=ORIENTED_EDGE('',*,*,#35437,.T.) ;
#45214=ORIENTED_EDGE('',*,*,#35445,.F.) ;
#45215=ORIENTED_EDGE('',*,*,#35439,.T.) ;
#45216=ORIENTED_EDGE('',*,*,#35441,.T.) ;
#45217=ORIENTED_EDGE('',*,*,#35440,.T.) ;
#45218=ORIENTED_EDGE('',*,*,#35446,.F.) ;
#45219=ORIENTED_EDGE('',*,*,#34825,.T.) ;
#45220=ORIENTED_EDGE('',*,*,#35443,.T.) ;
#45221=ORIENTED_EDGE('',*,*,#34822,.F.) ;
#45222=ORIENTED_EDGE('',*,*,#35447,.F.) ;
#45223=ORIENTED_EDGE('',*,*,#35255,.F.) ;
#45224=ORIENTED_EDGE('',*,*,#35444,.T.) ;
#45225=ORIENTED_EDGE('',*,*,#35256,.F.) ;
#45226=ORIENTED_EDGE('',*,*,#35448,.F.) ;
#45227=ORIENTED_EDGE('',*,*,#35258,.F.) ;
#45228=ORIENTED_EDGE('',*,*,#35445,.T.) ;
#45229=ORIENTED_EDGE('',*,*,#35260,.F.) ;
#45230=ORIENTED_EDGE('',*,*,#35449,.F.) ;
#45231=ORIENTED_EDGE('',*,*,#35262,.F.) ;
#45232=ORIENTED_EDGE('',*,*,#35446,.T.) ;
#45233=ORIENTED_EDGE('',*,*,#35263,.F.) ;
#45234=ORIENTED_EDGE('',*,*,#35450,.F.) ;
#45235=ORIENTED_EDGE('',*,*,#34826,.F.) ;
#45236=ORIENTED_EDGE('',*,*,#35447,.T.) ;
#45237=ORIENTED_EDGE('',*,*,#34821,.T.) ;
#45238=ORIENTED_EDGE('',*,*,#35451,.F.) ;
#45239=ORIENTED_EDGE('',*,*,#35448,.T.) ;
#45240=ORIENTED_EDGE('',*,*,#35450,.T.) ;
#45241=ORIENTED_EDGE('',*,*,#35449,.T.) ;
#45242=ORIENTED_EDGE('',*,*,#35452,.F.) ;
#45243=ORIENTED_EDGE('',*,*,#34827,.T.) ;
#45244=ORIENTED_EDGE('',*,*,#35451,.T.) ;
#45245=ORIENTED_EDGE('',*,*,#34828,.F.) ;
#45246=ORIENTED_EDGE('',*,*,#35452,.T.) ;
#45247=ORIENTED_EDGE('',*,*,#35259,.F.) ;
#45248=ORIENTED_EDGE('',*,*,#35453,.F.) ;
#45249=ORIENTED_EDGE('',*,*,#34769,.F.) ;
#45250=ORIENTED_EDGE('',*,*,#35454,.F.) ;
#45251=ORIENTED_EDGE('',*,*,#35235,.F.) ;
#45252=ORIENTED_EDGE('',*,*,#34762,.T.) ;
#45253=ORIENTED_EDGE('',*,*,#35453,.T.) ;
#45254=ORIENTED_EDGE('',*,*,#35455,.F.) ;
#45255=ORIENTED_EDGE('',*,*,#35456,.F.) ;
#45256=ORIENTED_EDGE('',*,*,#35454,.T.) ;
#45257=ORIENTED_EDGE('',*,*,#34768,.T.) ;
#45258=ORIENTED_EDGE('',*,*,#35457,.F.) ;
#45259=ORIENTED_EDGE('',*,*,#35458,.F.) ;
#45260=ORIENTED_EDGE('',*,*,#35455,.T.) ;
#45261=ORIENTED_EDGE('',*,*,#35234,.F.) ;
#45262=ORIENTED_EDGE('',*,*,#35459,.F.) ;
#45263=ORIENTED_EDGE('',*,*,#35246,.F.) ;
#45264=ORIENTED_EDGE('',*,*,#35456,.T.) ;
#45265=ORIENTED_EDGE('',*,*,#35245,.F.) ;
#45266=ORIENTED_EDGE('',*,*,#35460,.F.) ;
#45267=ORIENTED_EDGE('',*,*,#34763,.F.) ;
#45268=ORIENTED_EDGE('',*,*,#35461,.F.) ;
#45269=ORIENTED_EDGE('',*,*,#34765,.F.) ;
#45270=ORIENTED_EDGE('',*,*,#35462,.F.) ;
#45271=ORIENTED_EDGE('',*,*,#35241,.F.) ;
#45272=ORIENTED_EDGE('',*,*,#35457,.T.) ;
#45273=ORIENTED_EDGE('',*,*,#34767,.F.) ;
#45274=ORIENTED_EDGE('',*,*,#35463,.F.) ;
#45275=ORIENTED_EDGE('',*,*,#35237,.F.) ;
#45276=ORIENTED_EDGE('',*,*,#35458,.T.) ;
#45277=ORIENTED_EDGE('',*,*,#35240,.F.) ;
#45278=ORIENTED_EDGE('',*,*,#35464,.F.) ;
#45279=ORIENTED_EDGE('',*,*,#35236,.F.) ;
#45280=ORIENTED_EDGE('',*,*,#35465,.F.) ;
#45281=ORIENTED_EDGE('',*,*,#34808,.F.) ;
#45282=ORIENTED_EDGE('',*,*,#35466,.F.) ;
#45283=ORIENTED_EDGE('',*,*,#35233,.F.) ;
#45284=ORIENTED_EDGE('',*,*,#35466,.T.) ;
#45285=ORIENTED_EDGE('',*,*,#34807,.T.) ;
#45286=ORIENTED_EDGE('',*,*,#35467,.F.) ;
#45287=ORIENTED_EDGE('',*,*,#35459,.T.) ;
#45288=ORIENTED_EDGE('',*,*,#34764,.T.) ;
#45289=ORIENTED_EDGE('',*,*,#35460,.T.) ;
#45290=ORIENTED_EDGE('',*,*,#35468,.F.) ;
#45291=ORIENTED_EDGE('',*,*,#35462,.T.) ;
#45292=ORIENTED_EDGE('',*,*,#34766,.T.) ;
#45293=ORIENTED_EDGE('',*,*,#35461,.T.) ;
#45294=ORIENTED_EDGE('',*,*,#35469,.F.) ;
#45295=ORIENTED_EDGE('',*,*,#35463,.T.) ;
#45296=ORIENTED_EDGE('',*,*,#35465,.T.) ;
#45297=ORIENTED_EDGE('',*,*,#35464,.T.) ;
#45298=ORIENTED_EDGE('',*,*,#35470,.F.) ;
#45299=ORIENTED_EDGE('',*,*,#34809,.T.) ;
#45300=ORIENTED_EDGE('',*,*,#35467,.T.) ;
#45301=ORIENTED_EDGE('',*,*,#34806,.F.) ;
#45302=ORIENTED_EDGE('',*,*,#35471,.F.) ;
#45303=ORIENTED_EDGE('',*,*,#35247,.F.) ;
#45304=ORIENTED_EDGE('',*,*,#35468,.T.) ;
#45305=ORIENTED_EDGE('',*,*,#35248,.F.) ;
#45306=ORIENTED_EDGE('',*,*,#35472,.F.) ;
#45307=ORIENTED_EDGE('',*,*,#35242,.F.) ;
#45308=ORIENTED_EDGE('',*,*,#35469,.T.) ;
#45309=ORIENTED_EDGE('',*,*,#35244,.F.) ;
#45310=ORIENTED_EDGE('',*,*,#35473,.F.) ;
#45311=ORIENTED_EDGE('',*,*,#35238,.F.) ;
#45312=ORIENTED_EDGE('',*,*,#35470,.T.) ;
#45313=ORIENTED_EDGE('',*,*,#35239,.F.) ;
#45314=ORIENTED_EDGE('',*,*,#35474,.F.) ;
#45315=ORIENTED_EDGE('',*,*,#34810,.F.) ;
#45316=ORIENTED_EDGE('',*,*,#35471,.T.) ;
#45317=ORIENTED_EDGE('',*,*,#34805,.T.) ;
#45318=ORIENTED_EDGE('',*,*,#35475,.F.) ;
#45319=ORIENTED_EDGE('',*,*,#35472,.T.) ;
#45320=ORIENTED_EDGE('',*,*,#35474,.T.) ;
#45321=ORIENTED_EDGE('',*,*,#35473,.T.) ;
#45322=ORIENTED_EDGE('',*,*,#35476,.F.) ;
#45323=ORIENTED_EDGE('',*,*,#34811,.T.) ;
#45324=ORIENTED_EDGE('',*,*,#35475,.T.) ;
#45325=ORIENTED_EDGE('',*,*,#34812,.F.) ;
#45326=ORIENTED_EDGE('',*,*,#35476,.T.) ;
#45327=ORIENTED_EDGE('',*,*,#35243,.F.) ;
#45328=ORIENTED_EDGE('',*,*,#35477,.F.) ;
#45329=ORIENTED_EDGE('',*,*,#34793,.F.) ;
#45330=ORIENTED_EDGE('',*,*,#35478,.F.) ;
#45331=ORIENTED_EDGE('',*,*,#35219,.F.) ;
#45332=ORIENTED_EDGE('',*,*,#34786,.T.) ;
#45333=ORIENTED_EDGE('',*,*,#35477,.T.) ;
#45334=ORIENTED_EDGE('',*,*,#35479,.F.) ;
#45335=ORIENTED_EDGE('',*,*,#35480,.F.) ;
#45336=ORIENTED_EDGE('',*,*,#35478,.T.) ;
#45337=ORIENTED_EDGE('',*,*,#34792,.T.) ;
#45338=ORIENTED_EDGE('',*,*,#35481,.F.) ;
#45339=ORIENTED_EDGE('',*,*,#35482,.F.) ;
#45340=ORIENTED_EDGE('',*,*,#35479,.T.) ;
#45341=ORIENTED_EDGE('',*,*,#35218,.F.) ;
#45342=ORIENTED_EDGE('',*,*,#35483,.F.) ;
#45343=ORIENTED_EDGE('',*,*,#35222,.F.) ;
#45344=ORIENTED_EDGE('',*,*,#35480,.T.) ;
#45345=ORIENTED_EDGE('',*,*,#35221,.F.) ;
#45346=ORIENTED_EDGE('',*,*,#35484,.F.) ;
#45347=ORIENTED_EDGE('',*,*,#34787,.F.) ;
#45348=ORIENTED_EDGE('',*,*,#35485,.F.) ;
#45349=ORIENTED_EDGE('',*,*,#34789,.F.) ;
#45350=ORIENTED_EDGE('',*,*,#35486,.F.) ;
#45351=ORIENTED_EDGE('',*,*,#35225,.F.) ;
#45352=ORIENTED_EDGE('',*,*,#35481,.T.) ;
#45353=ORIENTED_EDGE('',*,*,#34791,.F.) ;
#45354=ORIENTED_EDGE('',*,*,#35487,.F.) ;
#45355=ORIENTED_EDGE('',*,*,#35229,.F.) ;
#45356=ORIENTED_EDGE('',*,*,#35482,.T.) ;
#45357=ORIENTED_EDGE('',*,*,#35232,.F.) ;
#45358=ORIENTED_EDGE('',*,*,#35488,.F.) ;
#45359=ORIENTED_EDGE('',*,*,#35220,.F.) ;
#45360=ORIENTED_EDGE('',*,*,#35489,.F.) ;
#45361=ORIENTED_EDGE('',*,*,#34832,.F.) ;
#45362=ORIENTED_EDGE('',*,*,#35490,.F.) ;
#45363=ORIENTED_EDGE('',*,*,#35217,.F.) ;
#45364=ORIENTED_EDGE('',*,*,#35490,.T.) ;
#45365=ORIENTED_EDGE('',*,*,#34831,.T.) ;
#45366=ORIENTED_EDGE('',*,*,#35491,.F.) ;
#45367=ORIENTED_EDGE('',*,*,#35483,.T.) ;
#45368=ORIENTED_EDGE('',*,*,#34788,.T.) ;
#45369=ORIENTED_EDGE('',*,*,#35484,.T.) ;
#45370=ORIENTED_EDGE('',*,*,#35492,.F.) ;
#45371=ORIENTED_EDGE('',*,*,#35486,.T.) ;
#45372=ORIENTED_EDGE('',*,*,#34790,.T.) ;
#45373=ORIENTED_EDGE('',*,*,#35485,.T.) ;
#45374=ORIENTED_EDGE('',*,*,#35493,.F.) ;
#45375=ORIENTED_EDGE('',*,*,#35487,.T.) ;
#45376=ORIENTED_EDGE('',*,*,#35489,.T.) ;
#45377=ORIENTED_EDGE('',*,*,#35488,.T.) ;
#45378=ORIENTED_EDGE('',*,*,#35494,.F.) ;
#45379=ORIENTED_EDGE('',*,*,#34833,.T.) ;
#45380=ORIENTED_EDGE('',*,*,#35491,.T.) ;
#45381=ORIENTED_EDGE('',*,*,#34830,.F.) ;
#45382=ORIENTED_EDGE('',*,*,#35495,.F.) ;
#45383=ORIENTED_EDGE('',*,*,#35223,.F.) ;
#45384=ORIENTED_EDGE('',*,*,#35492,.T.) ;
#45385=ORIENTED_EDGE('',*,*,#35224,.F.) ;
#45386=ORIENTED_EDGE('',*,*,#35496,.F.) ;
#45387=ORIENTED_EDGE('',*,*,#35226,.F.) ;
#45388=ORIENTED_EDGE('',*,*,#35493,.T.) ;
#45389=ORIENTED_EDGE('',*,*,#35228,.F.) ;
#45390=ORIENTED_EDGE('',*,*,#35497,.F.) ;
#45391=ORIENTED_EDGE('',*,*,#35230,.F.) ;
#45392=ORIENTED_EDGE('',*,*,#35494,.T.) ;
#45393=ORIENTED_EDGE('',*,*,#35231,.F.) ;
#45394=ORIENTED_EDGE('',*,*,#35498,.F.) ;
#45395=ORIENTED_EDGE('',*,*,#34834,.F.) ;
#45396=ORIENTED_EDGE('',*,*,#35495,.T.) ;
#45397=ORIENTED_EDGE('',*,*,#34829,.T.) ;
#45398=ORIENTED_EDGE('',*,*,#35499,.F.) ;
#45399=ORIENTED_EDGE('',*,*,#35496,.T.) ;
#45400=ORIENTED_EDGE('',*,*,#35498,.T.) ;
#45401=ORIENTED_EDGE('',*,*,#35497,.T.) ;
#45402=ORIENTED_EDGE('',*,*,#35500,.F.) ;
#45403=ORIENTED_EDGE('',*,*,#34835,.T.) ;
#45404=ORIENTED_EDGE('',*,*,#35499,.T.) ;
#45405=ORIENTED_EDGE('',*,*,#34836,.F.) ;
#45406=ORIENTED_EDGE('',*,*,#35500,.T.) ;
#45407=ORIENTED_EDGE('',*,*,#35227,.F.) ;
#45408=ORIENTED_EDGE('',*,*,#35501,.F.) ;
#45409=ORIENTED_EDGE('',*,*,#34732,.F.) ;
#45410=ORIENTED_EDGE('',*,*,#35502,.F.) ;
#45411=ORIENTED_EDGE('',*,*,#35285,.F.) ;
#45412=ORIENTED_EDGE('',*,*,#35502,.T.) ;
#45413=ORIENTED_EDGE('',*,*,#34731,.T.) ;
#45414=ORIENTED_EDGE('',*,*,#35503,.F.) ;
#45415=ORIENTED_EDGE('',*,*,#35504,.F.) ;
#45416=ORIENTED_EDGE('',*,*,#34733,.T.) ;
#45417=ORIENTED_EDGE('',*,*,#35501,.T.) ;
#45418=ORIENTED_EDGE('',*,*,#35505,.F.) ;
#45419=ORIENTED_EDGE('',*,*,#35506,.F.) ;
#45420=ORIENTED_EDGE('',*,*,#35503,.T.) ;
#45421=ORIENTED_EDGE('',*,*,#34730,.F.) ;
#45422=ORIENTED_EDGE('',*,*,#35507,.F.) ;
#45423=ORIENTED_EDGE('',*,*,#35284,.F.) ;
#45424=ORIENTED_EDGE('',*,*,#35504,.T.) ;
#45425=ORIENTED_EDGE('',*,*,#35283,.F.) ;
#45426=ORIENTED_EDGE('',*,*,#35508,.F.) ;
#45427=ORIENTED_EDGE('',*,*,#35286,.F.) ;
#45428=ORIENTED_EDGE('',*,*,#35509,.F.) ;
#45429=ORIENTED_EDGE('',*,*,#35287,.F.) ;
#45430=ORIENTED_EDGE('',*,*,#35510,.F.) ;
#45431=ORIENTED_EDGE('',*,*,#34750,.F.) ;
#45432=ORIENTED_EDGE('',*,*,#35505,.T.) ;
#45433=ORIENTED_EDGE('',*,*,#35288,.F.) ;
#45434=ORIENTED_EDGE('',*,*,#35511,.F.) ;
#45435=ORIENTED_EDGE('',*,*,#35289,.F.) ;
#45436=ORIENTED_EDGE('',*,*,#35506,.T.) ;
#45437=ORIENTED_EDGE('',*,*,#35292,.F.) ;
#45438=ORIENTED_EDGE('',*,*,#35512,.F.) ;
#45439=ORIENTED_EDGE('',*,*,#34734,.F.) ;
#45440=ORIENTED_EDGE('',*,*,#35513,.F.) ;
#45441=ORIENTED_EDGE('',*,*,#34736,.F.) ;
#45442=ORIENTED_EDGE('',*,*,#35514,.F.) ;
#45443=ORIENTED_EDGE('',*,*,#35295,.F.) ;
#45444=ORIENTED_EDGE('',*,*,#34729,.T.) ;
#45445=ORIENTED_EDGE('',*,*,#35513,.T.) ;
#45446=ORIENTED_EDGE('',*,*,#35515,.F.) ;
#45447=ORIENTED_EDGE('',*,*,#35507,.T.) ;
#45448=ORIENTED_EDGE('',*,*,#35510,.T.) ;
#45449=ORIENTED_EDGE('',*,*,#35508,.T.) ;
#45450=ORIENTED_EDGE('',*,*,#35516,.F.) ;
#45451=ORIENTED_EDGE('',*,*,#34743,.T.) ;
#45452=ORIENTED_EDGE('',*,*,#35509,.T.) ;
#45453=ORIENTED_EDGE('',*,*,#34749,.T.) ;
#45454=ORIENTED_EDGE('',*,*,#35517,.F.) ;
#45455=ORIENTED_EDGE('',*,*,#35511,.T.) ;
#45456=ORIENTED_EDGE('',*,*,#34735,.T.) ;
#45457=ORIENTED_EDGE('',*,*,#35512,.T.) ;
#45458=ORIENTED_EDGE('',*,*,#35518,.F.) ;
#45459=ORIENTED_EDGE('',*,*,#35514,.T.) ;
#45460=ORIENTED_EDGE('',*,*,#35515,.T.) ;
#45461=ORIENTED_EDGE('',*,*,#35294,.F.) ;
#45462=ORIENTED_EDGE('',*,*,#35519,.F.) ;
#45463=ORIENTED_EDGE('',*,*,#35281,.F.) ;
#45464=ORIENTED_EDGE('',*,*,#35516,.T.) ;
#45465=ORIENTED_EDGE('',*,*,#35282,.F.) ;
#45466=ORIENTED_EDGE('',*,*,#35520,.F.) ;
#45467=ORIENTED_EDGE('',*,*,#34744,.F.) ;
#45468=ORIENTED_EDGE('',*,*,#35517,.T.) ;
#45469=ORIENTED_EDGE('',*,*,#34748,.F.) ;
#45470=ORIENTED_EDGE('',*,*,#35521,.F.) ;
#45471=ORIENTED_EDGE('',*,*,#35290,.F.) ;
#45472=ORIENTED_EDGE('',*,*,#35518,.T.) ;
#45473=ORIENTED_EDGE('',*,*,#35291,.F.) ;
#45474=ORIENTED_EDGE('',*,*,#35522,.F.) ;
#45475=ORIENTED_EDGE('',*,*,#35296,.F.) ;
#45476=ORIENTED_EDGE('',*,*,#35520,.T.) ;
#45477=ORIENTED_EDGE('',*,*,#35519,.T.) ;
#45478=ORIENTED_EDGE('',*,*,#35523,.F.) ;
#45479=ORIENTED_EDGE('',*,*,#34745,.T.) ;
#45480=ORIENTED_EDGE('',*,*,#35521,.T.) ;
#45481=ORIENTED_EDGE('',*,*,#34747,.T.) ;
#45482=ORIENTED_EDGE('',*,*,#35524,.F.) ;
#45483=ORIENTED_EDGE('',*,*,#35522,.T.) ;
#45484=ORIENTED_EDGE('',*,*,#35523,.T.) ;
#45485=ORIENTED_EDGE('',*,*,#35293,.F.) ;
#45486=ORIENTED_EDGE('',*,*,#35524,.T.) ;
#45487=ORIENTED_EDGE('',*,*,#34746,.F.) ;
#45488=ORIENTED_EDGE('',*,*,#35525,.F.) ;
#45489=ORIENTED_EDGE('',*,*,#34879,.F.) ;
#45490=ORIENTED_EDGE('',*,*,#35526,.F.) ;
#45491=ORIENTED_EDGE('',*,*,#35115,.F.) ;
#45492=ORIENTED_EDGE('',*,*,#34872,.T.) ;
#45493=ORIENTED_EDGE('',*,*,#35525,.T.) ;
#45494=ORIENTED_EDGE('',*,*,#35527,.F.) ;
#45495=ORIENTED_EDGE('',*,*,#35528,.F.) ;
#45496=ORIENTED_EDGE('',*,*,#35526,.T.) ;
#45497=ORIENTED_EDGE('',*,*,#34878,.T.) ;
#45498=ORIENTED_EDGE('',*,*,#35529,.F.) ;
#45499=ORIENTED_EDGE('',*,*,#35530,.F.) ;
#45500=ORIENTED_EDGE('',*,*,#35527,.T.) ;
#45501=ORIENTED_EDGE('',*,*,#35114,.F.) ;
#45502=ORIENTED_EDGE('',*,*,#35531,.F.) ;
#45503=ORIENTED_EDGE('',*,*,#35118,.F.) ;
#45504=ORIENTED_EDGE('',*,*,#35528,.T.) ;
#45505=ORIENTED_EDGE('',*,*,#35117,.F.) ;
#45506=ORIENTED_EDGE('',*,*,#35532,.F.) ;
#45507=ORIENTED_EDGE('',*,*,#34873,.F.) ;
#45508=ORIENTED_EDGE('',*,*,#35533,.F.) ;
#45509=ORIENTED_EDGE('',*,*,#34875,.F.) ;
#45510=ORIENTED_EDGE('',*,*,#35534,.F.) ;
#45511=ORIENTED_EDGE('',*,*,#35105,.F.) ;
#45512=ORIENTED_EDGE('',*,*,#35529,.T.) ;
#45513=ORIENTED_EDGE('',*,*,#34877,.F.) ;
#45514=ORIENTED_EDGE('',*,*,#35535,.F.) ;
#45515=ORIENTED_EDGE('',*,*,#35109,.F.) ;
#45516=ORIENTED_EDGE('',*,*,#35530,.T.) ;
#45517=ORIENTED_EDGE('',*,*,#35112,.F.) ;
#45518=ORIENTED_EDGE('',*,*,#35536,.F.) ;
#45519=ORIENTED_EDGE('',*,*,#35116,.F.) ;
#45520=ORIENTED_EDGE('',*,*,#35537,.F.) ;
#45521=ORIENTED_EDGE('',*,*,#34942,.F.) ;
#45522=ORIENTED_EDGE('',*,*,#35538,.F.) ;
#45523=ORIENTED_EDGE('',*,*,#35113,.F.) ;
#45524=ORIENTED_EDGE('',*,*,#35538,.T.) ;
#45525=ORIENTED_EDGE('',*,*,#34941,.T.) ;
#45526=ORIENTED_EDGE('',*,*,#35539,.F.) ;
#45527=ORIENTED_EDGE('',*,*,#35531,.T.) ;
#45528=ORIENTED_EDGE('',*,*,#34874,.T.) ;
#45529=ORIENTED_EDGE('',*,*,#35532,.T.) ;
#45530=ORIENTED_EDGE('',*,*,#35540,.F.) ;
#45531=ORIENTED_EDGE('',*,*,#35534,.T.) ;
#45532=ORIENTED_EDGE('',*,*,#34876,.T.) ;
#45533=ORIENTED_EDGE('',*,*,#35533,.T.) ;
#45534=ORIENTED_EDGE('',*,*,#35541,.F.) ;
#45535=ORIENTED_EDGE('',*,*,#35535,.T.) ;
#45536=ORIENTED_EDGE('',*,*,#35537,.T.) ;
#45537=ORIENTED_EDGE('',*,*,#35536,.T.) ;
#45538=ORIENTED_EDGE('',*,*,#35542,.F.) ;
#45539=ORIENTED_EDGE('',*,*,#34943,.T.) ;
#45540=ORIENTED_EDGE('',*,*,#35539,.T.) ;
#45541=ORIENTED_EDGE('',*,*,#34940,.F.) ;
#45542=ORIENTED_EDGE('',*,*,#35543,.F.) ;
#45543=ORIENTED_EDGE('',*,*,#35119,.F.) ;
#45544=ORIENTED_EDGE('',*,*,#35540,.T.) ;
#45545=ORIENTED_EDGE('',*,*,#35120,.F.) ;
#45546=ORIENTED_EDGE('',*,*,#35544,.F.) ;
#45547=ORIENTED_EDGE('',*,*,#35106,.F.) ;
#45548=ORIENTED_EDGE('',*,*,#35541,.T.) ;
#45549=ORIENTED_EDGE('',*,*,#35108,.F.) ;
#45550=ORIENTED_EDGE('',*,*,#35545,.F.) ;
#45551=ORIENTED_EDGE('',*,*,#35110,.F.) ;
#45552=ORIENTED_EDGE('',*,*,#35542,.T.) ;
#45553=ORIENTED_EDGE('',*,*,#35111,.F.) ;
#45554=ORIENTED_EDGE('',*,*,#35546,.F.) ;
#45555=ORIENTED_EDGE('',*,*,#34944,.F.) ;
#45556=ORIENTED_EDGE('',*,*,#35543,.T.) ;
#45557=ORIENTED_EDGE('',*,*,#34939,.T.) ;
#45558=ORIENTED_EDGE('',*,*,#35547,.F.) ;
#45559=ORIENTED_EDGE('',*,*,#35544,.T.) ;
#45560=ORIENTED_EDGE('',*,*,#35546,.T.) ;
#45561=ORIENTED_EDGE('',*,*,#35545,.T.) ;
#45562=ORIENTED_EDGE('',*,*,#35548,.F.) ;
#45563=ORIENTED_EDGE('',*,*,#34945,.T.) ;
#45564=ORIENTED_EDGE('',*,*,#35547,.T.) ;
#45565=ORIENTED_EDGE('',*,*,#34946,.F.) ;
#45566=ORIENTED_EDGE('',*,*,#35548,.T.) ;
#45567=ORIENTED_EDGE('',*,*,#35107,.F.) ;
#45568=ORIENTED_EDGE('',*,*,#35549,.F.) ;
#45569=ORIENTED_EDGE('',*,*,#34887,.F.) ;
#45570=ORIENTED_EDGE('',*,*,#35550,.F.) ;
#45571=ORIENTED_EDGE('',*,*,#35131,.F.) ;
#45572=ORIENTED_EDGE('',*,*,#34880,.T.) ;
#45573=ORIENTED_EDGE('',*,*,#35549,.T.) ;
#45574=ORIENTED_EDGE('',*,*,#35551,.F.) ;
#45575=ORIENTED_EDGE('',*,*,#35552,.F.) ;
#45576=ORIENTED_EDGE('',*,*,#35550,.T.) ;
#45577=ORIENTED_EDGE('',*,*,#34886,.T.) ;
#45578=ORIENTED_EDGE('',*,*,#35553,.F.) ;
#45579=ORIENTED_EDGE('',*,*,#35554,.F.) ;
#45580=ORIENTED_EDGE('',*,*,#35551,.T.) ;
#45581=ORIENTED_EDGE('',*,*,#35130,.F.) ;
#45582=ORIENTED_EDGE('',*,*,#35555,.F.) ;
#45583=ORIENTED_EDGE('',*,*,#35134,.F.) ;
#45584=ORIENTED_EDGE('',*,*,#35552,.T.) ;
#45585=ORIENTED_EDGE('',*,*,#35133,.F.) ;
#45586=ORIENTED_EDGE('',*,*,#35556,.F.) ;
#45587=ORIENTED_EDGE('',*,*,#34881,.F.) ;
#45588=ORIENTED_EDGE('',*,*,#35557,.F.) ;
#45589=ORIENTED_EDGE('',*,*,#34883,.F.) ;
#45590=ORIENTED_EDGE('',*,*,#35558,.F.) ;
#45591=ORIENTED_EDGE('',*,*,#35121,.F.) ;
#45592=ORIENTED_EDGE('',*,*,#35553,.T.) ;
#45593=ORIENTED_EDGE('',*,*,#34885,.F.) ;
#45594=ORIENTED_EDGE('',*,*,#35559,.F.) ;
#45595=ORIENTED_EDGE('',*,*,#35125,.F.) ;
#45596=ORIENTED_EDGE('',*,*,#35554,.T.) ;
#45597=ORIENTED_EDGE('',*,*,#35128,.F.) ;
#45598=ORIENTED_EDGE('',*,*,#35560,.F.) ;
#45599=ORIENTED_EDGE('',*,*,#35132,.F.) ;
#45600=ORIENTED_EDGE('',*,*,#35561,.F.) ;
#45601=ORIENTED_EDGE('',*,*,#34950,.F.) ;
#45602=ORIENTED_EDGE('',*,*,#35562,.F.) ;
#45603=ORIENTED_EDGE('',*,*,#35129,.F.) ;
#45604=ORIENTED_EDGE('',*,*,#35562,.T.) ;
#45605=ORIENTED_EDGE('',*,*,#34949,.T.) ;
#45606=ORIENTED_EDGE('',*,*,#35563,.F.) ;
#45607=ORIENTED_EDGE('',*,*,#35555,.T.) ;
#45608=ORIENTED_EDGE('',*,*,#34882,.T.) ;
#45609=ORIENTED_EDGE('',*,*,#35556,.T.) ;
#45610=ORIENTED_EDGE('',*,*,#35564,.F.) ;
#45611=ORIENTED_EDGE('',*,*,#35558,.T.) ;
#45612=ORIENTED_EDGE('',*,*,#34884,.T.) ;
#45613=ORIENTED_EDGE('',*,*,#35557,.T.) ;
#45614=ORIENTED_EDGE('',*,*,#35565,.F.) ;
#45615=ORIENTED_EDGE('',*,*,#35559,.T.) ;
#45616=ORIENTED_EDGE('',*,*,#35561,.T.) ;
#45617=ORIENTED_EDGE('',*,*,#35560,.T.) ;
#45618=ORIENTED_EDGE('',*,*,#35566,.F.) ;
#45619=ORIENTED_EDGE('',*,*,#34951,.T.) ;
#45620=ORIENTED_EDGE('',*,*,#35563,.T.) ;
#45621=ORIENTED_EDGE('',*,*,#34948,.F.) ;
#45622=ORIENTED_EDGE('',*,*,#35567,.F.) ;
#45623=ORIENTED_EDGE('',*,*,#35135,.F.) ;
#45624=ORIENTED_EDGE('',*,*,#35564,.T.) ;
#45625=ORIENTED_EDGE('',*,*,#35136,.F.) ;
#45626=ORIENTED_EDGE('',*,*,#35568,.F.) ;
#45627=ORIENTED_EDGE('',*,*,#35122,.F.) ;
#45628=ORIENTED_EDGE('',*,*,#35565,.T.) ;
#45629=ORIENTED_EDGE('',*,*,#35124,.F.) ;
#45630=ORIENTED_EDGE('',*,*,#35569,.F.) ;
#45631=ORIENTED_EDGE('',*,*,#35126,.F.) ;
#45632=ORIENTED_EDGE('',*,*,#35566,.T.) ;
#45633=ORIENTED_EDGE('',*,*,#35127,.F.) ;
#45634=ORIENTED_EDGE('',*,*,#35570,.F.) ;
#45635=ORIENTED_EDGE('',*,*,#34952,.F.) ;
#45636=ORIENTED_EDGE('',*,*,#35567,.T.) ;
#45637=ORIENTED_EDGE('',*,*,#34947,.T.) ;
#45638=ORIENTED_EDGE('',*,*,#35571,.F.) ;
#45639=ORIENTED_EDGE('',*,*,#35568,.T.) ;
#45640=ORIENTED_EDGE('',*,*,#35570,.T.) ;
#45641=ORIENTED_EDGE('',*,*,#35569,.T.) ;
#45642=ORIENTED_EDGE('',*,*,#35572,.F.) ;
#45643=ORIENTED_EDGE('',*,*,#34953,.T.) ;
#45644=ORIENTED_EDGE('',*,*,#35571,.T.) ;
#45645=ORIENTED_EDGE('',*,*,#34954,.F.) ;
#45646=ORIENTED_EDGE('',*,*,#35572,.T.) ;
#45647=ORIENTED_EDGE('',*,*,#35123,.F.) ;
#45648=ORIENTED_EDGE('',*,*,#35573,.F.) ;
#45649=ORIENTED_EDGE('',*,*,#34871,.F.) ;
#45650=ORIENTED_EDGE('',*,*,#35574,.F.) ;
#45651=ORIENTED_EDGE('',*,*,#35147,.F.) ;
#45652=ORIENTED_EDGE('',*,*,#34864,.T.) ;
#45653=ORIENTED_EDGE('',*,*,#35573,.T.) ;
#45654=ORIENTED_EDGE('',*,*,#35575,.F.) ;
#45655=ORIENTED_EDGE('',*,*,#35576,.F.) ;
#45656=ORIENTED_EDGE('',*,*,#35574,.T.) ;
#45657=ORIENTED_EDGE('',*,*,#34870,.T.) ;
#45658=ORIENTED_EDGE('',*,*,#35577,.F.) ;
#45659=ORIENTED_EDGE('',*,*,#35578,.F.) ;
#45660=ORIENTED_EDGE('',*,*,#35575,.T.) ;
#45661=ORIENTED_EDGE('',*,*,#35146,.F.) ;
#45662=ORIENTED_EDGE('',*,*,#35579,.F.) ;
#45663=ORIENTED_EDGE('',*,*,#35150,.F.) ;
#45664=ORIENTED_EDGE('',*,*,#35576,.T.) ;
#45665=ORIENTED_EDGE('',*,*,#35149,.F.) ;
#45666=ORIENTED_EDGE('',*,*,#35580,.F.) ;
#45667=ORIENTED_EDGE('',*,*,#34865,.F.) ;
#45668=ORIENTED_EDGE('',*,*,#35581,.F.) ;
#45669=ORIENTED_EDGE('',*,*,#34867,.F.) ;
#45670=ORIENTED_EDGE('',*,*,#35582,.F.) ;
#45671=ORIENTED_EDGE('',*,*,#35137,.F.) ;
#45672=ORIENTED_EDGE('',*,*,#35577,.T.) ;
#45673=ORIENTED_EDGE('',*,*,#34869,.F.) ;
#45674=ORIENTED_EDGE('',*,*,#35583,.F.) ;
#45675=ORIENTED_EDGE('',*,*,#35141,.F.) ;
#45676=ORIENTED_EDGE('',*,*,#35578,.T.) ;
#45677=ORIENTED_EDGE('',*,*,#35144,.F.) ;
#45678=ORIENTED_EDGE('',*,*,#35584,.F.) ;
#45679=ORIENTED_EDGE('',*,*,#35148,.F.) ;
#45680=ORIENTED_EDGE('',*,*,#35585,.F.) ;
#45681=ORIENTED_EDGE('',*,*,#34934,.F.) ;
#45682=ORIENTED_EDGE('',*,*,#35586,.F.) ;
#45683=ORIENTED_EDGE('',*,*,#35145,.F.) ;
#45684=ORIENTED_EDGE('',*,*,#35586,.T.) ;
#45685=ORIENTED_EDGE('',*,*,#34933,.T.) ;
#45686=ORIENTED_EDGE('',*,*,#35587,.F.) ;
#45687=ORIENTED_EDGE('',*,*,#35579,.T.) ;
#45688=ORIENTED_EDGE('',*,*,#34866,.T.) ;
#45689=ORIENTED_EDGE('',*,*,#35580,.T.) ;
#45690=ORIENTED_EDGE('',*,*,#35588,.F.) ;
#45691=ORIENTED_EDGE('',*,*,#35582,.T.) ;
#45692=ORIENTED_EDGE('',*,*,#34868,.T.) ;
#45693=ORIENTED_EDGE('',*,*,#35581,.T.) ;
#45694=ORIENTED_EDGE('',*,*,#35589,.F.) ;
#45695=ORIENTED_EDGE('',*,*,#35583,.T.) ;
#45696=ORIENTED_EDGE('',*,*,#35585,.T.) ;
#45697=ORIENTED_EDGE('',*,*,#35584,.T.) ;
#45698=ORIENTED_EDGE('',*,*,#35590,.F.) ;
#45699=ORIENTED_EDGE('',*,*,#34935,.T.) ;
#45700=ORIENTED_EDGE('',*,*,#35587,.T.) ;
#45701=ORIENTED_EDGE('',*,*,#34932,.F.) ;
#45702=ORIENTED_EDGE('',*,*,#35591,.F.) ;
#45703=ORIENTED_EDGE('',*,*,#35151,.F.) ;
#45704=ORIENTED_EDGE('',*,*,#35588,.T.) ;
#45705=ORIENTED_EDGE('',*,*,#35152,.F.) ;
#45706=ORIENTED_EDGE('',*,*,#35592,.F.) ;
#45707=ORIENTED_EDGE('',*,*,#35138,.F.) ;
#45708=ORIENTED_EDGE('',*,*,#35589,.T.) ;
#45709=ORIENTED_EDGE('',*,*,#35140,.F.) ;
#45710=ORIENTED_EDGE('',*,*,#35593,.F.) ;
#45711=ORIENTED_EDGE('',*,*,#35142,.F.) ;
#45712=ORIENTED_EDGE('',*,*,#35590,.T.) ;
#45713=ORIENTED_EDGE('',*,*,#35143,.F.) ;
#45714=ORIENTED_EDGE('',*,*,#35594,.F.) ;
#45715=ORIENTED_EDGE('',*,*,#34936,.F.) ;
#45716=ORIENTED_EDGE('',*,*,#35591,.T.) ;
#45717=ORIENTED_EDGE('',*,*,#34931,.T.) ;
#45718=ORIENTED_EDGE('',*,*,#35595,.F.) ;
#45719=ORIENTED_EDGE('',*,*,#35592,.T.) ;
#45720=ORIENTED_EDGE('',*,*,#35594,.T.) ;
#45721=ORIENTED_EDGE('',*,*,#35593,.T.) ;
#45722=ORIENTED_EDGE('',*,*,#35596,.F.) ;
#45723=ORIENTED_EDGE('',*,*,#34937,.T.) ;
#45724=ORIENTED_EDGE('',*,*,#35595,.T.) ;
#45725=ORIENTED_EDGE('',*,*,#34938,.F.) ;
#45726=ORIENTED_EDGE('',*,*,#35596,.T.) ;
#45727=ORIENTED_EDGE('',*,*,#35139,.F.) ;
#45728=ORIENTED_EDGE('',*,*,#35597,.F.) ;
#45729=ORIENTED_EDGE('',*,*,#34895,.F.) ;
#45730=ORIENTED_EDGE('',*,*,#35598,.F.) ;
#45731=ORIENTED_EDGE('',*,*,#35163,.F.) ;
#45732=ORIENTED_EDGE('',*,*,#34888,.T.) ;
#45733=ORIENTED_EDGE('',*,*,#35597,.T.) ;
#45734=ORIENTED_EDGE('',*,*,#35599,.F.) ;
#45735=ORIENTED_EDGE('',*,*,#35600,.F.) ;
#45736=ORIENTED_EDGE('',*,*,#35598,.T.) ;
#45737=ORIENTED_EDGE('',*,*,#34894,.T.) ;
#45738=ORIENTED_EDGE('',*,*,#35601,.F.) ;
#45739=ORIENTED_EDGE('',*,*,#35602,.F.) ;
#45740=ORIENTED_EDGE('',*,*,#35599,.T.) ;
#45741=ORIENTED_EDGE('',*,*,#35162,.F.) ;
#45742=ORIENTED_EDGE('',*,*,#35603,.F.) ;
#45743=ORIENTED_EDGE('',*,*,#35166,.F.) ;
#45744=ORIENTED_EDGE('',*,*,#35600,.T.) ;
#45745=ORIENTED_EDGE('',*,*,#35165,.F.) ;
#45746=ORIENTED_EDGE('',*,*,#35604,.F.) ;
#45747=ORIENTED_EDGE('',*,*,#34889,.F.) ;
#45748=ORIENTED_EDGE('',*,*,#35605,.F.) ;
#45749=ORIENTED_EDGE('',*,*,#34891,.F.) ;
#45750=ORIENTED_EDGE('',*,*,#35606,.F.) ;
#45751=ORIENTED_EDGE('',*,*,#35153,.F.) ;
#45752=ORIENTED_EDGE('',*,*,#35601,.T.) ;
#45753=ORIENTED_EDGE('',*,*,#34893,.F.) ;
#45754=ORIENTED_EDGE('',*,*,#35607,.F.) ;
#45755=ORIENTED_EDGE('',*,*,#35157,.F.) ;
#45756=ORIENTED_EDGE('',*,*,#35602,.T.) ;
#45757=ORIENTED_EDGE('',*,*,#35160,.F.) ;
#45758=ORIENTED_EDGE('',*,*,#35608,.F.) ;
#45759=ORIENTED_EDGE('',*,*,#35164,.F.) ;
#45760=ORIENTED_EDGE('',*,*,#35609,.F.) ;
#45761=ORIENTED_EDGE('',*,*,#34958,.F.) ;
#45762=ORIENTED_EDGE('',*,*,#35610,.F.) ;
#45763=ORIENTED_EDGE('',*,*,#35161,.F.) ;
#45764=ORIENTED_EDGE('',*,*,#35610,.T.) ;
#45765=ORIENTED_EDGE('',*,*,#34957,.T.) ;
#45766=ORIENTED_EDGE('',*,*,#35611,.F.) ;
#45767=ORIENTED_EDGE('',*,*,#35603,.T.) ;
#45768=ORIENTED_EDGE('',*,*,#34890,.T.) ;
#45769=ORIENTED_EDGE('',*,*,#35604,.T.) ;
#45770=ORIENTED_EDGE('',*,*,#35612,.F.) ;
#45771=ORIENTED_EDGE('',*,*,#35606,.T.) ;
#45772=ORIENTED_EDGE('',*,*,#34892,.T.) ;
#45773=ORIENTED_EDGE('',*,*,#35605,.T.) ;
#45774=ORIENTED_EDGE('',*,*,#35613,.F.) ;
#45775=ORIENTED_EDGE('',*,*,#35607,.T.) ;
#45776=ORIENTED_EDGE('',*,*,#35609,.T.) ;
#45777=ORIENTED_EDGE('',*,*,#35608,.T.) ;
#45778=ORIENTED_EDGE('',*,*,#35614,.F.) ;
#45779=ORIENTED_EDGE('',*,*,#34959,.T.) ;
#45780=ORIENTED_EDGE('',*,*,#35611,.T.) ;
#45781=ORIENTED_EDGE('',*,*,#34956,.F.) ;
#45782=ORIENTED_EDGE('',*,*,#35615,.F.) ;
#45783=ORIENTED_EDGE('',*,*,#35167,.F.) ;
#45784=ORIENTED_EDGE('',*,*,#35612,.T.) ;
#45785=ORIENTED_EDGE('',*,*,#35168,.F.) ;
#45786=ORIENTED_EDGE('',*,*,#35616,.F.) ;
#45787=ORIENTED_EDGE('',*,*,#35154,.F.) ;
#45788=ORIENTED_EDGE('',*,*,#35613,.T.) ;
#45789=ORIENTED_EDGE('',*,*,#35156,.F.) ;
#45790=ORIENTED_EDGE('',*,*,#35617,.F.) ;
#45791=ORIENTED_EDGE('',*,*,#35158,.F.) ;
#45792=ORIENTED_EDGE('',*,*,#35614,.T.) ;
#45793=ORIENTED_EDGE('',*,*,#35159,.F.) ;
#45794=ORIENTED_EDGE('',*,*,#35618,.F.) ;
#45795=ORIENTED_EDGE('',*,*,#34960,.F.) ;
#45796=ORIENTED_EDGE('',*,*,#35615,.T.) ;
#45797=ORIENTED_EDGE('',*,*,#34955,.T.) ;
#45798=ORIENTED_EDGE('',*,*,#35619,.F.) ;
#45799=ORIENTED_EDGE('',*,*,#35616,.T.) ;
#45800=ORIENTED_EDGE('',*,*,#35618,.T.) ;
#45801=ORIENTED_EDGE('',*,*,#35617,.T.) ;
#45802=ORIENTED_EDGE('',*,*,#35620,.F.) ;
#45803=ORIENTED_EDGE('',*,*,#34961,.T.) ;
#45804=ORIENTED_EDGE('',*,*,#35619,.T.) ;
#45805=ORIENTED_EDGE('',*,*,#34962,.F.) ;
#45806=ORIENTED_EDGE('',*,*,#35620,.T.) ;
#45807=ORIENTED_EDGE('',*,*,#35155,.F.) ;
#45808=ORIENTED_EDGE('',*,*,#35621,.F.) ;
#45809=ORIENTED_EDGE('',*,*,#34863,.F.) ;
#45810=ORIENTED_EDGE('',*,*,#35622,.F.) ;
#45811=ORIENTED_EDGE('',*,*,#35179,.F.) ;
#45812=ORIENTED_EDGE('',*,*,#34856,.T.) ;
#45813=ORIENTED_EDGE('',*,*,#35621,.T.) ;
#45814=ORIENTED_EDGE('',*,*,#35623,.F.) ;
#45815=ORIENTED_EDGE('',*,*,#35624,.F.) ;
#45816=ORIENTED_EDGE('',*,*,#35622,.T.) ;
#45817=ORIENTED_EDGE('',*,*,#34862,.T.) ;
#45818=ORIENTED_EDGE('',*,*,#35625,.F.) ;
#45819=ORIENTED_EDGE('',*,*,#35626,.F.) ;
#45820=ORIENTED_EDGE('',*,*,#35623,.T.) ;
#45821=ORIENTED_EDGE('',*,*,#35178,.F.) ;
#45822=ORIENTED_EDGE('',*,*,#35627,.F.) ;
#45823=ORIENTED_EDGE('',*,*,#35182,.F.) ;
#45824=ORIENTED_EDGE('',*,*,#35624,.T.) ;
#45825=ORIENTED_EDGE('',*,*,#35181,.F.) ;
#45826=ORIENTED_EDGE('',*,*,#35628,.F.) ;
#45827=ORIENTED_EDGE('',*,*,#34857,.F.) ;
#45828=ORIENTED_EDGE('',*,*,#35629,.F.) ;
#45829=ORIENTED_EDGE('',*,*,#34859,.F.) ;
#45830=ORIENTED_EDGE('',*,*,#35630,.F.) ;
#45831=ORIENTED_EDGE('',*,*,#35169,.F.) ;
#45832=ORIENTED_EDGE('',*,*,#35625,.T.) ;
#45833=ORIENTED_EDGE('',*,*,#34861,.F.) ;
#45834=ORIENTED_EDGE('',*,*,#35631,.F.) ;
#45835=ORIENTED_EDGE('',*,*,#35173,.F.) ;
#45836=ORIENTED_EDGE('',*,*,#35626,.T.) ;
#45837=ORIENTED_EDGE('',*,*,#35176,.F.) ;
#45838=ORIENTED_EDGE('',*,*,#35632,.F.) ;
#45839=ORIENTED_EDGE('',*,*,#35180,.F.) ;
#45840=ORIENTED_EDGE('',*,*,#35633,.F.) ;
#45841=ORIENTED_EDGE('',*,*,#34926,.F.) ;
#45842=ORIENTED_EDGE('',*,*,#35634,.F.) ;
#45843=ORIENTED_EDGE('',*,*,#35177,.F.) ;
#45844=ORIENTED_EDGE('',*,*,#35634,.T.) ;
#45845=ORIENTED_EDGE('',*,*,#34925,.T.) ;
#45846=ORIENTED_EDGE('',*,*,#35635,.F.) ;
#45847=ORIENTED_EDGE('',*,*,#35627,.T.) ;
#45848=ORIENTED_EDGE('',*,*,#34858,.T.) ;
#45849=ORIENTED_EDGE('',*,*,#35628,.T.) ;
#45850=ORIENTED_EDGE('',*,*,#35636,.F.) ;
#45851=ORIENTED_EDGE('',*,*,#35630,.T.) ;
#45852=ORIENTED_EDGE('',*,*,#34860,.T.) ;
#45853=ORIENTED_EDGE('',*,*,#35629,.T.) ;
#45854=ORIENTED_EDGE('',*,*,#35637,.F.) ;
#45855=ORIENTED_EDGE('',*,*,#35631,.T.) ;
#45856=ORIENTED_EDGE('',*,*,#35633,.T.) ;
#45857=ORIENTED_EDGE('',*,*,#35632,.T.) ;
#45858=ORIENTED_EDGE('',*,*,#35638,.F.) ;
#45859=ORIENTED_EDGE('',*,*,#34927,.T.) ;
#45860=ORIENTED_EDGE('',*,*,#35635,.T.) ;
#45861=ORIENTED_EDGE('',*,*,#34924,.F.) ;
#45862=ORIENTED_EDGE('',*,*,#35639,.F.) ;
#45863=ORIENTED_EDGE('',*,*,#35183,.F.) ;
#45864=ORIENTED_EDGE('',*,*,#35636,.T.) ;
#45865=ORIENTED_EDGE('',*,*,#35184,.F.) ;
#45866=ORIENTED_EDGE('',*,*,#35640,.F.) ;
#45867=ORIENTED_EDGE('',*,*,#35170,.F.) ;
#45868=ORIENTED_EDGE('',*,*,#35637,.T.) ;
#45869=ORIENTED_EDGE('',*,*,#35172,.F.) ;
#45870=ORIENTED_EDGE('',*,*,#35641,.F.) ;
#45871=ORIENTED_EDGE('',*,*,#35174,.F.) ;
#45872=ORIENTED_EDGE('',*,*,#35638,.T.) ;
#45873=ORIENTED_EDGE('',*,*,#35175,.F.) ;
#45874=ORIENTED_EDGE('',*,*,#35642,.F.) ;
#45875=ORIENTED_EDGE('',*,*,#34928,.F.) ;
#45876=ORIENTED_EDGE('',*,*,#35639,.T.) ;
#45877=ORIENTED_EDGE('',*,*,#34923,.T.) ;
#45878=ORIENTED_EDGE('',*,*,#35643,.F.) ;
#45879=ORIENTED_EDGE('',*,*,#35640,.T.) ;
#45880=ORIENTED_EDGE('',*,*,#35642,.T.) ;
#45881=ORIENTED_EDGE('',*,*,#35641,.T.) ;
#45882=ORIENTED_EDGE('',*,*,#35644,.F.) ;
#45883=ORIENTED_EDGE('',*,*,#34929,.T.) ;
#45884=ORIENTED_EDGE('',*,*,#35643,.T.) ;
#45885=ORIENTED_EDGE('',*,*,#34930,.F.) ;
#45886=ORIENTED_EDGE('',*,*,#35644,.T.) ;
#45887=ORIENTED_EDGE('',*,*,#35171,.F.) ;
#45888=ORIENTED_EDGE('',*,*,#35645,.F.) ;
#45889=ORIENTED_EDGE('',*,*,#34903,.F.) ;
#45890=ORIENTED_EDGE('',*,*,#35646,.F.) ;
#45891=ORIENTED_EDGE('',*,*,#35187,.F.) ;
#45892=ORIENTED_EDGE('',*,*,#34896,.T.) ;
#45893=ORIENTED_EDGE('',*,*,#35645,.T.) ;
#45894=ORIENTED_EDGE('',*,*,#35647,.F.) ;
#45895=ORIENTED_EDGE('',*,*,#35648,.F.) ;
#45896=ORIENTED_EDGE('',*,*,#35646,.T.) ;
#45897=ORIENTED_EDGE('',*,*,#34902,.T.) ;
#45898=ORIENTED_EDGE('',*,*,#35649,.F.) ;
#45899=ORIENTED_EDGE('',*,*,#35650,.F.) ;
#45900=ORIENTED_EDGE('',*,*,#35647,.T.) ;
#45901=ORIENTED_EDGE('',*,*,#35186,.F.) ;
#45902=ORIENTED_EDGE('',*,*,#35651,.F.) ;
#45903=ORIENTED_EDGE('',*,*,#35190,.F.) ;
#45904=ORIENTED_EDGE('',*,*,#35648,.T.) ;
#45905=ORIENTED_EDGE('',*,*,#35189,.F.) ;
#45906=ORIENTED_EDGE('',*,*,#35652,.F.) ;
#45907=ORIENTED_EDGE('',*,*,#34897,.F.) ;
#45908=ORIENTED_EDGE('',*,*,#35653,.F.) ;
#45909=ORIENTED_EDGE('',*,*,#34899,.F.) ;
#45910=ORIENTED_EDGE('',*,*,#35654,.F.) ;
#45911=ORIENTED_EDGE('',*,*,#35193,.F.) ;
#45912=ORIENTED_EDGE('',*,*,#35649,.T.) ;
#45913=ORIENTED_EDGE('',*,*,#34901,.F.) ;
#45914=ORIENTED_EDGE('',*,*,#35655,.F.) ;
#45915=ORIENTED_EDGE('',*,*,#35197,.F.) ;
#45916=ORIENTED_EDGE('',*,*,#35650,.T.) ;
#45917=ORIENTED_EDGE('',*,*,#35200,.F.) ;
#45918=ORIENTED_EDGE('',*,*,#35656,.F.) ;
#45919=ORIENTED_EDGE('',*,*,#35188,.F.) ;
#45920=ORIENTED_EDGE('',*,*,#35657,.F.) ;
#45921=ORIENTED_EDGE('',*,*,#34966,.F.) ;
#45922=ORIENTED_EDGE('',*,*,#35658,.F.) ;
#45923=ORIENTED_EDGE('',*,*,#35185,.F.) ;
#45924=ORIENTED_EDGE('',*,*,#35658,.T.) ;
#45925=ORIENTED_EDGE('',*,*,#34965,.T.) ;
#45926=ORIENTED_EDGE('',*,*,#35659,.F.) ;
#45927=ORIENTED_EDGE('',*,*,#35651,.T.) ;
#45928=ORIENTED_EDGE('',*,*,#34898,.T.) ;
#45929=ORIENTED_EDGE('',*,*,#35652,.T.) ;
#45930=ORIENTED_EDGE('',*,*,#35660,.F.) ;
#45931=ORIENTED_EDGE('',*,*,#35654,.T.) ;
#45932=ORIENTED_EDGE('',*,*,#34900,.T.) ;
#45933=ORIENTED_EDGE('',*,*,#35653,.T.) ;
#45934=ORIENTED_EDGE('',*,*,#35661,.F.) ;
#45935=ORIENTED_EDGE('',*,*,#35655,.T.) ;
#45936=ORIENTED_EDGE('',*,*,#35657,.T.) ;
#45937=ORIENTED_EDGE('',*,*,#35656,.T.) ;
#45938=ORIENTED_EDGE('',*,*,#35662,.F.) ;
#45939=ORIENTED_EDGE('',*,*,#34967,.T.) ;
#45940=ORIENTED_EDGE('',*,*,#35659,.T.) ;
#45941=ORIENTED_EDGE('',*,*,#34964,.F.) ;
#45942=ORIENTED_EDGE('',*,*,#35663,.F.) ;
#45943=ORIENTED_EDGE('',*,*,#35191,.F.) ;
#45944=ORIENTED_EDGE('',*,*,#35660,.T.) ;
#45945=ORIENTED_EDGE('',*,*,#35192,.F.) ;
#45946=ORIENTED_EDGE('',*,*,#35664,.F.) ;
#45947=ORIENTED_EDGE('',*,*,#35194,.F.) ;
#45948=ORIENTED_EDGE('',*,*,#35661,.T.) ;
#45949=ORIENTED_EDGE('',*,*,#35196,.F.) ;
#45950=ORIENTED_EDGE('',*,*,#35665,.F.) ;
#45951=ORIENTED_EDGE('',*,*,#35198,.F.) ;
#45952=ORIENTED_EDGE('',*,*,#35662,.T.) ;
#45953=ORIENTED_EDGE('',*,*,#35199,.F.) ;
#45954=ORIENTED_EDGE('',*,*,#35666,.F.) ;
#45955=ORIENTED_EDGE('',*,*,#34968,.F.) ;
#45956=ORIENTED_EDGE('',*,*,#35663,.T.) ;
#45957=ORIENTED_EDGE('',*,*,#34963,.T.) ;
#45958=ORIENTED_EDGE('',*,*,#35667,.F.) ;
#45959=ORIENTED_EDGE('',*,*,#35664,.T.) ;
#45960=ORIENTED_EDGE('',*,*,#35666,.T.) ;
#45961=ORIENTED_EDGE('',*,*,#35665,.T.) ;
#45962=ORIENTED_EDGE('',*,*,#35668,.F.) ;
#45963=ORIENTED_EDGE('',*,*,#34969,.T.) ;
#45964=ORIENTED_EDGE('',*,*,#35667,.T.) ;
#45965=ORIENTED_EDGE('',*,*,#34970,.F.) ;
#45966=ORIENTED_EDGE('',*,*,#35668,.T.) ;
#45967=ORIENTED_EDGE('',*,*,#35195,.F.) ;
#45968=ORIENTED_EDGE('',*,*,#35669,.F.) ;
#45969=ORIENTED_EDGE('',*,*,#34855,.F.) ;
#45970=ORIENTED_EDGE('',*,*,#35670,.F.) ;
#45971=ORIENTED_EDGE('',*,*,#35215,.F.) ;
#45972=ORIENTED_EDGE('',*,*,#34848,.T.) ;
#45973=ORIENTED_EDGE('',*,*,#35669,.T.) ;
#45974=ORIENTED_EDGE('',*,*,#35671,.F.) ;
#45975=ORIENTED_EDGE('',*,*,#35672,.F.) ;
#45976=ORIENTED_EDGE('',*,*,#35670,.T.) ;
#45977=ORIENTED_EDGE('',*,*,#34854,.T.) ;
#45978=ORIENTED_EDGE('',*,*,#35673,.F.) ;
#45979=ORIENTED_EDGE('',*,*,#35674,.F.) ;
#45980=ORIENTED_EDGE('',*,*,#35671,.T.) ;
#45981=ORIENTED_EDGE('',*,*,#35214,.F.) ;
#45982=ORIENTED_EDGE('',*,*,#35675,.F.) ;
#45983=ORIENTED_EDGE('',*,*,#35202,.F.) ;
#45984=ORIENTED_EDGE('',*,*,#35672,.T.) ;
#45985=ORIENTED_EDGE('',*,*,#35201,.F.) ;
#45986=ORIENTED_EDGE('',*,*,#35676,.F.) ;
#45987=ORIENTED_EDGE('',*,*,#34849,.F.) ;
#45988=ORIENTED_EDGE('',*,*,#35677,.F.) ;
#45989=ORIENTED_EDGE('',*,*,#34851,.F.) ;
#45990=ORIENTED_EDGE('',*,*,#35678,.F.) ;
#45991=ORIENTED_EDGE('',*,*,#35205,.F.) ;
#45992=ORIENTED_EDGE('',*,*,#35673,.T.) ;
#45993=ORIENTED_EDGE('',*,*,#34853,.F.) ;
#45994=ORIENTED_EDGE('',*,*,#35679,.F.) ;
#45995=ORIENTED_EDGE('',*,*,#35209,.F.) ;
#45996=ORIENTED_EDGE('',*,*,#35674,.T.) ;
#45997=ORIENTED_EDGE('',*,*,#35212,.F.) ;
#45998=ORIENTED_EDGE('',*,*,#35680,.F.) ;
#45999=ORIENTED_EDGE('',*,*,#35216,.F.) ;
#46000=ORIENTED_EDGE('',*,*,#35681,.F.) ;
#46001=ORIENTED_EDGE('',*,*,#34918,.F.) ;
#46002=ORIENTED_EDGE('',*,*,#35682,.F.) ;
#46003=ORIENTED_EDGE('',*,*,#35213,.F.) ;
#46004=ORIENTED_EDGE('',*,*,#35682,.T.) ;
#46005=ORIENTED_EDGE('',*,*,#34917,.T.) ;
#46006=ORIENTED_EDGE('',*,*,#35683,.F.) ;
#46007=ORIENTED_EDGE('',*,*,#35675,.T.) ;
#46008=ORIENTED_EDGE('',*,*,#34850,.T.) ;
#46009=ORIENTED_EDGE('',*,*,#35676,.T.) ;
#46010=ORIENTED_EDGE('',*,*,#35684,.F.) ;
#46011=ORIENTED_EDGE('',*,*,#35678,.T.) ;
#46012=ORIENTED_EDGE('',*,*,#34852,.T.) ;
#46013=ORIENTED_EDGE('',*,*,#35677,.T.) ;
#46014=ORIENTED_EDGE('',*,*,#35685,.F.) ;
#46015=ORIENTED_EDGE('',*,*,#35679,.T.) ;
#46016=ORIENTED_EDGE('',*,*,#35681,.T.) ;
#46017=ORIENTED_EDGE('',*,*,#35680,.T.) ;
#46018=ORIENTED_EDGE('',*,*,#35686,.F.) ;
#46019=ORIENTED_EDGE('',*,*,#34919,.T.) ;
#46020=ORIENTED_EDGE('',*,*,#35683,.T.) ;
#46021=ORIENTED_EDGE('',*,*,#34916,.F.) ;
#46022=ORIENTED_EDGE('',*,*,#35687,.F.) ;
#46023=ORIENTED_EDGE('',*,*,#35203,.F.) ;
#46024=ORIENTED_EDGE('',*,*,#35684,.T.) ;
#46025=ORIENTED_EDGE('',*,*,#35204,.F.) ;
#46026=ORIENTED_EDGE('',*,*,#35688,.F.) ;
#46027=ORIENTED_EDGE('',*,*,#35206,.F.) ;
#46028=ORIENTED_EDGE('',*,*,#35685,.T.) ;
#46029=ORIENTED_EDGE('',*,*,#35208,.F.) ;
#46030=ORIENTED_EDGE('',*,*,#35689,.F.) ;
#46031=ORIENTED_EDGE('',*,*,#35210,.F.) ;
#46032=ORIENTED_EDGE('',*,*,#35686,.T.) ;
#46033=ORIENTED_EDGE('',*,*,#35211,.F.) ;
#46034=ORIENTED_EDGE('',*,*,#35690,.F.) ;
#46035=ORIENTED_EDGE('',*,*,#34920,.F.) ;
#46036=ORIENTED_EDGE('',*,*,#35687,.T.) ;
#46037=ORIENTED_EDGE('',*,*,#34915,.T.) ;
#46038=ORIENTED_EDGE('',*,*,#35691,.F.) ;
#46039=ORIENTED_EDGE('',*,*,#35688,.T.) ;
#46040=ORIENTED_EDGE('',*,*,#35690,.T.) ;
#46041=ORIENTED_EDGE('',*,*,#35689,.T.) ;
#46042=ORIENTED_EDGE('',*,*,#35692,.F.) ;
#46043=ORIENTED_EDGE('',*,*,#34921,.T.) ;
#46044=ORIENTED_EDGE('',*,*,#35691,.T.) ;
#46045=ORIENTED_EDGE('',*,*,#34922,.F.) ;
#46046=ORIENTED_EDGE('',*,*,#35692,.T.) ;
#46047=ORIENTED_EDGE('',*,*,#35207,.F.) ;
#46048=ORIENTED_EDGE('',*,*,#35693,.F.) ;
#46049=ORIENTED_EDGE('',*,*,#34738,.F.) ;
#46050=ORIENTED_EDGE('',*,*,#35694,.F.) ;
#46051=ORIENTED_EDGE('',*,*,#35058,.F.) ;
#46052=ORIENTED_EDGE('',*,*,#35695,.F.) ;
#46053=ORIENTED_EDGE('',*,*,#34742,.F.) ;
#46054=ORIENTED_EDGE('',*,*,#35696,.F.) ;
#46055=ORIENTED_EDGE('',*,*,#35050,.F.) ;
#46056=ORIENTED_EDGE('',*,*,#35697,.F.) ;
#46057=ORIENTED_EDGE('',*,*,#34737,.F.) ;
#46058=ORIENTED_EDGE('',*,*,#35698,.F.) ;
#46059=ORIENTED_EDGE('',*,*,#35054,.F.) ;
#46060=ORIENTED_EDGE('',*,*,#35694,.T.) ;
#46061=ORIENTED_EDGE('',*,*,#35697,.T.) ;
#46062=ORIENTED_EDGE('',*,*,#35699,.F.) ;
#46063=ORIENTED_EDGE('',*,*,#35693,.T.) ;
#46064=ORIENTED_EDGE('',*,*,#35057,.F.) ;
#46065=ORIENTED_EDGE('',*,*,#35700,.F.) ;
#46066=ORIENTED_EDGE('',*,*,#35060,.F.) ;
#46067=ORIENTED_EDGE('',*,*,#35696,.T.) ;
#46068=ORIENTED_EDGE('',*,*,#35062,.F.) ;
#46069=ORIENTED_EDGE('',*,*,#35701,.F.) ;
#46070=ORIENTED_EDGE('',*,*,#35051,.F.) ;
#46071=ORIENTED_EDGE('',*,*,#35698,.T.) ;
#46072=ORIENTED_EDGE('',*,*,#35695,.T.) ;
#46073=ORIENTED_EDGE('',*,*,#35702,.F.) ;
#46074=ORIENTED_EDGE('',*,*,#35699,.T.) ;
#46075=ORIENTED_EDGE('',*,*,#35053,.F.) ;
#46076=ORIENTED_EDGE('',*,*,#35703,.F.) ;
#46077=ORIENTED_EDGE('',*,*,#35059,.F.) ;
#46078=ORIENTED_EDGE('',*,*,#35700,.T.) ;
#46079=ORIENTED_EDGE('',*,*,#35056,.F.) ;
#46080=ORIENTED_EDGE('',*,*,#35704,.F.) ;
#46081=ORIENTED_EDGE('',*,*,#34724,.F.) ;
#46082=ORIENTED_EDGE('',*,*,#35701,.T.) ;
#46083=ORIENTED_EDGE('',*,*,#34726,.F.) ;
#46084=ORIENTED_EDGE('',*,*,#35705,.F.) ;
#46085=ORIENTED_EDGE('',*,*,#35048,.F.) ;
#46086=ORIENTED_EDGE('',*,*,#35702,.T.) ;
#46087=ORIENTED_EDGE('',*,*,#35049,.F.) ;
#46088=ORIENTED_EDGE('',*,*,#35706,.F.) ;
#46089=ORIENTED_EDGE('',*,*,#35055,.F.) ;
#46090=ORIENTED_EDGE('',*,*,#35704,.T.) ;
#46091=ORIENTED_EDGE('',*,*,#35703,.T.) ;
#46092=ORIENTED_EDGE('',*,*,#35707,.F.) ;
#46093=ORIENTED_EDGE('',*,*,#35706,.T.) ;
#46094=ORIENTED_EDGE('',*,*,#35705,.T.) ;
#46095=ORIENTED_EDGE('',*,*,#35708,.F.) ;
#46096=ORIENTED_EDGE('',*,*,#35707,.T.) ;
#46097=ORIENTED_EDGE('',*,*,#35052,.F.) ;
#46098=ORIENTED_EDGE('',*,*,#35708,.T.) ;
#46099=ORIENTED_EDGE('',*,*,#34725,.F.) ;
#62814=TOROIDAL_SURFACE('',#67765,1.75,0.15) ;
#62815=TOROIDAL_SURFACE('',#67770,1.75,0.15) ;
#62816=TOROIDAL_SURFACE('',#67775,1.64999999999999,0.15) ;
#62817=TOROIDAL_SURFACE('',#67781,1.64999999999999,0.15) ;
#62818=TOROIDAL_SURFACE('',#67785,1.64999999999999,0.15) ;
#62819=TOROIDAL_SURFACE('',#67791,1.64999999999999,0.15) ;
#62820=TOROIDAL_SURFACE('',#68047,0.3,0.15) ;
#62821=TOROIDAL_SURFACE('',#68056,0.3,0.15) ;
#62822=TOROIDAL_SURFACE('',#68083,0.3,0.15) ;
#62823=TOROIDAL_SURFACE('',#68103,0.3,0.15) ;
#62824=TOROIDAL_SURFACE('',#68105,1.6,0.15) ;
#62825=TOROIDAL_SURFACE('',#68122,1.15,0.15) ;
#62826=TOROIDAL_SURFACE('',#68124,0.3,0.15) ;
#62827=TOROIDAL_SURFACE('',#68127,0.3,0.15) ;
#62828=TOROIDAL_SURFACE('',#68144,0.3,0.15) ;
#62829=TOROIDAL_SURFACE('',#68152,0.3,0.15) ;
#62830=TOROIDAL_SURFACE('',#68171,1.6,0.15) ;
#62831=TOROIDAL_SURFACE('',#68197,0.3,0.15) ;
#62832=TOROIDAL_SURFACE('',#68199,0.3,0.15) ;
#62833=TOROIDAL_SURFACE('',#68211,0.3,0.15) ;
#62834=TOROIDAL_SURFACE('',#68213,0.3,0.15) ;
#62835=TOROIDAL_SURFACE('',#68219,1.15,0.15) ;
#62836=TOROIDAL_SURFACE('',#68223,0.3,0.15) ;
#62837=TOROIDAL_SURFACE('',#68226,0.3,0.15) ;
#62838=TOROIDAL_SURFACE('',#68243,0.3,0.15) ;
#62839=TOROIDAL_SURFACE('',#68245,0.3,0.15) ;
#62840=TOROIDAL_SURFACE('',#68247,0.3,0.15) ;
#62841=TOROIDAL_SURFACE('',#68249,0.3,0.15) ;
#62842=TOROIDAL_SURFACE('',#68259,0.3,0.15) ;
#62843=TOROIDAL_SURFACE('',#68261,0.3,0.15) ;
#62844=TOROIDAL_SURFACE('',#68267,0.3,0.15) ;
#62845=TOROIDAL_SURFACE('',#68270,0.3,0.15) ;
#62846=TOROIDAL_SURFACE('',#68287,0.3,0.15) ;
#62847=TOROIDAL_SURFACE('',#68289,0.3,0.15) ;
#62848=TOROIDAL_SURFACE('',#68291,0.3,0.15) ;
#62849=TOROIDAL_SURFACE('',#68293,0.3,0.15) ;
#62850=TOROIDAL_SURFACE('',#68303,0.3,0.15) ;
#62851=TOROIDAL_SURFACE('',#68305,0.3,0.15) ;
#62852=TOROIDAL_SURFACE('',#68311,0.3,0.15) ;
#62853=TOROIDAL_SURFACE('',#68314,0.3,0.15) ;
#62854=TOROIDAL_SURFACE('',#68331,0.3,0.15) ;
#62855=TOROIDAL_SURFACE('',#68333,0.3,0.15) ;
#62856=TOROIDAL_SURFACE('',#68335,0.3,0.15) ;
#62857=TOROIDAL_SURFACE('',#68337,0.3,0.15) ;
#62858=TOROIDAL_SURFACE('',#68347,0.3,0.15) ;
#62859=TOROIDAL_SURFACE('',#68349,0.3,0.15) ;
#62860=TOROIDAL_SURFACE('',#68355,0.3,0.15) ;
#62861=TOROIDAL_SURFACE('',#68358,0.3,0.15) ;
#62862=TOROIDAL_SURFACE('',#68375,0.3,0.15) ;
#62863=TOROIDAL_SURFACE('',#68377,0.3,0.15) ;
#62864=TOROIDAL_SURFACE('',#68379,0.3,0.15) ;
#62865=TOROIDAL_SURFACE('',#68381,0.3,0.15) ;
#62866=TOROIDAL_SURFACE('',#68391,0.3,0.15) ;
#62867=TOROIDAL_SURFACE('',#68393,0.3,0.15) ;
#62868=TOROIDAL_SURFACE('',#68399,0.3,0.15) ;
#62869=TOROIDAL_SURFACE('',#68402,0.3,0.15) ;
#62870=TOROIDAL_SURFACE('',#68419,0.3,0.15) ;
#62871=TOROIDAL_SURFACE('',#68421,0.3,0.15) ;
#62872=TOROIDAL_SURFACE('',#68423,0.3,0.15) ;
#62873=TOROIDAL_SURFACE('',#68425,0.3,0.15) ;
#62874=TOROIDAL_SURFACE('',#68435,0.3,0.15) ;
#62875=TOROIDAL_SURFACE('',#68437,0.3,0.15) ;
#62876=TOROIDAL_SURFACE('',#68443,0.3,0.15) ;
#62877=TOROIDAL_SURFACE('',#68446,0.3,0.15) ;
#62878=TOROIDAL_SURFACE('',#68463,0.3,0.15) ;
#62879=TOROIDAL_SURFACE('',#68465,0.3,0.15) ;
#62880=TOROIDAL_SURFACE('',#68467,0.3,0.15) ;
#62881=TOROIDAL_SURFACE('',#68469,0.3,0.15) ;
#62882=TOROIDAL_SURFACE('',#68479,0.3,0.15) ;
#62883=TOROIDAL_SURFACE('',#68481,0.3,0.15) ;
#62884=TOROIDAL_SURFACE('',#68487,0.3,0.15) ;
#62885=TOROIDAL_SURFACE('',#68490,0.3,0.15) ;
#62886=TOROIDAL_SURFACE('',#68507,0.3,0.15) ;
#62887=TOROIDAL_SURFACE('',#68509,0.3,0.15) ;
#62888=TOROIDAL_SURFACE('',#68511,0.3,0.15) ;
#62889=TOROIDAL_SURFACE('',#68513,0.3,0.15) ;
#62890=TOROIDAL_SURFACE('',#68523,0.3,0.15) ;
#62891=TOROIDAL_SURFACE('',#68525,0.3,0.15) ;
#62892=TOROIDAL_SURFACE('',#68531,0.3,0.15) ;
#62893=TOROIDAL_SURFACE('',#68534,0.3,0.15) ;
#62894=TOROIDAL_SURFACE('',#68551,0.3,0.15) ;
#62895=TOROIDAL_SURFACE('',#68553,0.3,0.15) ;
#62896=TOROIDAL_SURFACE('',#68555,0.3,0.15) ;
#62897=TOROIDAL_SURFACE('',#68557,0.3,0.15) ;
#62898=TOROIDAL_SURFACE('',#68567,0.3,0.15) ;
#62899=TOROIDAL_SURFACE('',#68569,0.3,0.15) ;
#62900=TOROIDAL_SURFACE('',#68575,0.3,0.15) ;
#62901=TOROIDAL_SURFACE('',#68578,0.3,0.15) ;
#62902=TOROIDAL_SURFACE('',#68595,0.3,0.15) ;
#62903=TOROIDAL_SURFACE('',#68597,0.3,0.15) ;
#62904=TOROIDAL_SURFACE('',#68599,0.3,0.15) ;
#62905=TOROIDAL_SURFACE('',#68601,0.3,0.15) ;
#62906=TOROIDAL_SURFACE('',#68611,0.3,0.15) ;
#62907=TOROIDAL_SURFACE('',#68613,0.3,0.15) ;
#62908=TOROIDAL_SURFACE('',#68619,0.3,0.15) ;
#62909=TOROIDAL_SURFACE('',#68622,0.3,0.15) ;
#62910=TOROIDAL_SURFACE('',#68639,0.3,0.15) ;
#62911=TOROIDAL_SURFACE('',#68641,0.3,0.15) ;
#62912=TOROIDAL_SURFACE('',#68643,0.3,0.15) ;
#62913=TOROIDAL_SURFACE('',#68645,0.3,0.15) ;
#62914=TOROIDAL_SURFACE('',#68655,0.3,0.15) ;
#62915=TOROIDAL_SURFACE('',#68657,0.3,0.15) ;
#62916=TOROIDAL_SURFACE('',#68663,0.3,0.15) ;
#62917=TOROIDAL_SURFACE('',#68666,0.3,0.15) ;
#62918=TOROIDAL_SURFACE('',#68683,0.3,0.15) ;
#62919=TOROIDAL_SURFACE('',#68685,0.3,0.15) ;
#62920=TOROIDAL_SURFACE('',#68687,0.3,0.15) ;
#62921=TOROIDAL_SURFACE('',#68689,0.3,0.15) ;
#62922=TOROIDAL_SURFACE('',#68699,0.3,0.15) ;
#62923=TOROIDAL_SURFACE('',#68701,0.3,0.15) ;
#62924=TOROIDAL_SURFACE('',#68707,0.3,0.15) ;
#62925=TOROIDAL_SURFACE('',#68710,0.3,0.15) ;
#62926=TOROIDAL_SURFACE('',#68727,0.3,0.15) ;
#62927=TOROIDAL_SURFACE('',#68729,0.3,0.15) ;
#62928=TOROIDAL_SURFACE('',#68731,0.3,0.15) ;
#62929=TOROIDAL_SURFACE('',#68733,0.3,0.15) ;
#62930=TOROIDAL_SURFACE('',#68743,0.3,0.15) ;
#62931=TOROIDAL_SURFACE('',#68745,0.3,0.15) ;
#63444=ADVANCED_FACE('',(#16159),#62814,.T.) ;
#63445=ADVANCED_FACE('',(#16160),#62815,.T.) ;
#63446=ADVANCED_FACE('',(#16161),#62816,.T.) ;
#63447=ADVANCED_FACE('',(#16162),#62817,.T.) ;
#63448=ADVANCED_FACE('',(#16163),#62818,.T.) ;
#63449=ADVANCED_FACE('',(#16164),#62819,.T.) ;
#63450=ADVANCED_FACE('',(#16165),#16128,.F.) ;
#63451=ADVANCED_FACE('',(#16166),#5947,.F.) ;
#63452=ADVANCED_FACE('',(#16167),#16129,.F.) ;
#63453=ADVANCED_FACE('',(#16168),#5948,.F.) ;
#63454=ADVANCED_FACE('',(#16169),#5949,.F.) ;
#63455=ADVANCED_FACE('',(#16170,#4989,#4990),#5065,.F.) ;
#63456=ADVANCED_FACE('',(#16171,#4991,#4992),#5066,.T.) ;
#63457=ADVANCED_FACE('',(#16172,#4993,#4994,#4995,#4996),#5067,.T.) ;
#63458=ADVANCED_FACE('',(#16173,#4997,#4998,#4999,#5000),#5068,.F.) ;
#63459=ADVANCED_FACE('',(#16174,#5001,#5002,#5003,#5004,#5005,#5006,#5007),
#5069,.T.) ;
#63460=ADVANCED_FACE('',(#16175,#5008,#5009,#5010,#5011,#5012,#5013,#5014),
#5070,.F.) ;
#63461=ADVANCED_FACE('',(#16176,#5015,#5016),#5071,.T.) ;
#63462=ADVANCED_FACE('',(#16177,#5017,#5018),#5072,.F.) ;
#63463=ADVANCED_FACE('',(#16178),#5073,.T.) ;
#63464=ADVANCED_FACE('',(#16179),#5074,.T.) ;
#63465=ADVANCED_FACE('',(#16180),#5075,.T.) ;
#63466=ADVANCED_FACE('',(#16181),#5076,.T.) ;
#63467=ADVANCED_FACE('',(#16182),#5077,.T.) ;
#63468=ADVANCED_FACE('',(#16183),#5078,.T.) ;
#63469=ADVANCED_FACE('',(#16184),#5079,.T.) ;
#63470=ADVANCED_FACE('',(#16185),#5950,.T.) ;
#63471=ADVANCED_FACE('',(#16186),#5951,.F.) ;
#63472=ADVANCED_FACE('',(#16187),#5080,.T.) ;
#63473=ADVANCED_FACE('',(#16188),#5081,.T.) ;
#63474=ADVANCED_FACE('',(#16189),#5082,.T.) ;
#63475=ADVANCED_FACE('',(#16190),#5083,.T.) ;
#63476=ADVANCED_FACE('',(#16191),#5084,.T.) ;
#63477=ADVANCED_FACE('',(#16192),#5085,.F.) ;
#63478=ADVANCED_FACE('',(#16193),#5086,.T.) ;
#63479=ADVANCED_FACE('',(#16194),#5087,.T.) ;
#63480=ADVANCED_FACE('',(#16195),#5088,.T.) ;
#63481=ADVANCED_FACE('',(#16196),#5089,.F.) ;
#63482=ADVANCED_FACE('',(#16197),#5090,.F.) ;
#63483=ADVANCED_FACE('',(#16198),#5091,.F.) ;
#63484=ADVANCED_FACE('',(#16199),#5092,.T.) ;
#63485=ADVANCED_FACE('',(#16200),#5093,.T.) ;
#63486=ADVANCED_FACE('',(#16201),#5094,.T.) ;
#63487=ADVANCED_FACE('',(#16202),#5952,.T.) ;
#63488=ADVANCED_FACE('',(#16203),#5953,.F.) ;
#63489=ADVANCED_FACE('',(#16204),#5095,.T.) ;
#63490=ADVANCED_FACE('',(#16205),#5096,.T.) ;
#63491=ADVANCED_FACE('',(#16206),#5954,.T.) ;
#63492=ADVANCED_FACE('',(#16207),#5955,.F.) ;
#63493=ADVANCED_FACE('',(#16208),#5097,.F.) ;
#63494=ADVANCED_FACE('',(#16209),#5098,.F.) ;
#63495=ADVANCED_FACE('',(#16210),#5099,.F.) ;
#63496=ADVANCED_FACE('',(#16211),#5100,.F.) ;
#63497=ADVANCED_FACE('',(#16212),#5101,.T.) ;
#63498=ADVANCED_FACE('',(#16213),#5102,.T.) ;
#63499=ADVANCED_FACE('',(#16214),#5103,.T.) ;
#63500=ADVANCED_FACE('',(#16215),#5104,.F.) ;
#63501=ADVANCED_FACE('',(#16216),#5105,.F.) ;
#63502=ADVANCED_FACE('',(#16217),#5106,.F.) ;
#63503=ADVANCED_FACE('',(#16218),#5107,.F.) ;
#63504=ADVANCED_FACE('',(#16219),#5108,.F.) ;
#63505=ADVANCED_FACE('',(#16220),#5109,.F.) ;
#63506=ADVANCED_FACE('',(#16221),#5110,.F.) ;
#63507=ADVANCED_FACE('',(#16222),#5111,.F.) ;
#63508=ADVANCED_FACE('',(#16223),#5112,.F.) ;
#63509=ADVANCED_FACE('',(#16224),#5113,.F.) ;
#63510=ADVANCED_FACE('',(#16225),#5114,.F.) ;
#63511=ADVANCED_FACE('',(#16226),#5115,.F.) ;
#63512=ADVANCED_FACE('',(#16227),#5116,.F.) ;
#63513=ADVANCED_FACE('',(#16228),#5117,.F.) ;
#63514=ADVANCED_FACE('',(#16229),#5118,.F.) ;
#63515=ADVANCED_FACE('',(#16230),#5119,.F.) ;
#63516=ADVANCED_FACE('',(#16231),#5120,.F.) ;
#63517=ADVANCED_FACE('',(#16232),#5121,.F.) ;
#63518=ADVANCED_FACE('',(#16233),#5122,.F.) ;
#63519=ADVANCED_FACE('',(#16234),#5123,.F.) ;
#63520=ADVANCED_FACE('',(#16235),#5124,.F.) ;
#63521=ADVANCED_FACE('',(#16236),#5125,.F.) ;
#63522=ADVANCED_FACE('',(#16237),#5126,.F.) ;
#63523=ADVANCED_FACE('',(#16238),#5127,.F.) ;
#63524=ADVANCED_FACE('',(#16239),#5128,.F.) ;
#63525=ADVANCED_FACE('',(#16240),#5129,.F.) ;
#63526=ADVANCED_FACE('',(#16241),#5130,.F.) ;
#63527=ADVANCED_FACE('',(#16242),#5131,.F.) ;
#63528=ADVANCED_FACE('',(#16243),#5132,.F.) ;
#63529=ADVANCED_FACE('',(#16244),#5133,.F.) ;
#63530=ADVANCED_FACE('',(#16245),#5134,.F.) ;
#63531=ADVANCED_FACE('',(#16246),#5135,.F.) ;
#63532=ADVANCED_FACE('',(#16247),#5136,.F.) ;
#63533=ADVANCED_FACE('',(#16248),#5137,.F.) ;
#63534=ADVANCED_FACE('',(#16249),#5138,.F.) ;
#63535=ADVANCED_FACE('',(#16250),#5139,.F.) ;
#63536=ADVANCED_FACE('',(#16251),#5140,.F.) ;
#63537=ADVANCED_FACE('',(#16252),#5141,.F.) ;
#63538=ADVANCED_FACE('',(#16253),#5142,.F.) ;
#63539=ADVANCED_FACE('',(#16254),#5143,.F.) ;
#63540=ADVANCED_FACE('',(#16255),#5144,.F.) ;
#63541=ADVANCED_FACE('',(#16256),#5145,.F.) ;
#63542=ADVANCED_FACE('',(#16257),#5146,.F.) ;
#63543=ADVANCED_FACE('',(#16258),#5147,.F.) ;
#63544=ADVANCED_FACE('',(#16259),#5148,.F.) ;
#63545=ADVANCED_FACE('',(#16260),#5149,.F.) ;
#63546=ADVANCED_FACE('',(#16261),#5150,.F.) ;
#63547=ADVANCED_FACE('',(#16262),#5151,.F.) ;
#63548=ADVANCED_FACE('',(#16263),#5152,.F.) ;
#63549=ADVANCED_FACE('',(#16264),#5956,.T.) ;
#63550=ADVANCED_FACE('',(#16265),#5957,.T.) ;
#63551=ADVANCED_FACE('',(#16266),#4182,.T.) ;
#63552=ADVANCED_FACE('',(#16267),#5958,.T.) ;
#63553=ADVANCED_FACE('',(#16268),#5959,.T.) ;
#63554=ADVANCED_FACE('',(#16269),#5960,.T.) ;
#63555=ADVANCED_FACE('',(#16270),#4183,.T.) ;
#63556=ADVANCED_FACE('',(#16271),#4184,.T.) ;
#63557=ADVANCED_FACE('',(#16272),#5961,.T.) ;
#63558=ADVANCED_FACE('',(#16273),#5962,.T.) ;
#63559=ADVANCED_FACE('',(#16274),#5963,.T.) ;
#63560=ADVANCED_FACE('',(#16275),#4185,.T.) ;
#63561=ADVANCED_FACE('',(#16276),#62820,.T.) ;
#63562=ADVANCED_FACE('',(#16277),#5964,.T.) ;
#63563=ADVANCED_FACE('',(#16278),#5965,.F.) ;
#63564=ADVANCED_FACE('',(#16279),#5966,.T.) ;
#63565=ADVANCED_FACE('',(#16280),#62821,.T.) ;
#63566=ADVANCED_FACE('',(#16281),#4186,.T.) ;
#63567=ADVANCED_FACE('',(#16282),#5967,.T.) ;
#63568=ADVANCED_FACE('',(#16283),#5968,.T.) ;
#63569=ADVANCED_FACE('',(#16284),#5969,.T.) ;
#63570=ADVANCED_FACE('',(#16285),#4187,.T.) ;
#63571=ADVANCED_FACE('',(#16286),#4188,.T.) ;
#63572=ADVANCED_FACE('',(#16287),#5970,.T.) ;
#63573=ADVANCED_FACE('',(#16288),#5971,.T.) ;
#63574=ADVANCED_FACE('',(#16289),#5972,.T.) ;
#63575=ADVANCED_FACE('',(#16290),#5973,.T.) ;
#63576=ADVANCED_FACE('',(#16291),#4189,.T.) ;
#63577=ADVANCED_FACE('',(#16292),#62822,.T.) ;
#63578=ADVANCED_FACE('',(#16293),#4190,.T.) ;
#63579=ADVANCED_FACE('',(#16294),#5974,.T.) ;
#63580=ADVANCED_FACE('',(#16295),#5975,.T.) ;
#63581=ADVANCED_FACE('',(#16296),#5976,.F.) ;
#63582=ADVANCED_FACE('',(#16297),#5977,.T.) ;
#63583=ADVANCED_FACE('',(#16298),#5978,.T.) ;
#63584=ADVANCED_FACE('',(#16299),#5979,.T.) ;
#63585=ADVANCED_FACE('',(#16300),#5980,.T.) ;
#63586=ADVANCED_FACE('',(#16301),#62823,.T.) ;
#63587=ADVANCED_FACE('',(#16302),#62824,.T.) ;
#63588=ADVANCED_FACE('',(#16303),#4191,.T.) ;
#63589=ADVANCED_FACE('',(#16304),#4192,.T.) ;
#63590=ADVANCED_FACE('',(#16305),#5981,.T.) ;
#63591=ADVANCED_FACE('',(#16306),#5982,.T.) ;
#63592=ADVANCED_FACE('',(#16307),#5983,.T.) ;
#63593=ADVANCED_FACE('',(#16308),#5984,.T.) ;
#63594=ADVANCED_FACE('',(#16309),#5985,.T.) ;
#63595=ADVANCED_FACE('',(#16310),#62825,.T.) ;
#63596=ADVANCED_FACE('',(#16311),#62826,.T.) ;
#63597=ADVANCED_FACE('',(#16312),#62827,.T.) ;
#63598=ADVANCED_FACE('',(#16313),#4193,.T.) ;
#63599=ADVANCED_FACE('',(#16314),#5986,.T.) ;
#63600=ADVANCED_FACE('',(#16315),#5987,.F.) ;
#63601=ADVANCED_FACE('',(#16316),#5988,.T.) ;
#63602=ADVANCED_FACE('',(#16317),#5989,.T.) ;
#63603=ADVANCED_FACE('',(#16318),#5990,.F.) ;
#63604=ADVANCED_FACE('',(#16319),#5991,.T.) ;
#63605=ADVANCED_FACE('',(#16320),#62828,.T.) ;
#63606=ADVANCED_FACE('',(#16321),#4194,.T.) ;
#63607=ADVANCED_FACE('',(#16322),#4195,.T.) ;
#63608=ADVANCED_FACE('',(#16323),#62829,.T.) ;
#63609=ADVANCED_FACE('',(#16324),#5992,.T.) ;
#63610=ADVANCED_FACE('',(#16325),#5993,.T.) ;
#63611=ADVANCED_FACE('',(#16326),#5994,.T.) ;
#63612=ADVANCED_FACE('',(#16327),#5995,.T.) ;
#63613=ADVANCED_FACE('',(#16328),#5996,.T.) ;
#63614=ADVANCED_FACE('',(#16329),#5997,.T.) ;
#63615=ADVANCED_FACE('',(#16330),#4196,.T.) ;
#63616=ADVANCED_FACE('',(#16331),#4197,.T.) ;
#63617=ADVANCED_FACE('',(#16332),#62830,.T.) ;
#63618=ADVANCED_FACE('',(#16333),#4198,.T.) ;
#63619=ADVANCED_FACE('',(#16334),#4199,.T.) ;
#63620=ADVANCED_FACE('',(#16335),#5998,.T.) ;
#63621=ADVANCED_FACE('',(#16336),#5999,.T.) ;
#63622=ADVANCED_FACE('',(#16337),#6000,.T.) ;
#63623=ADVANCED_FACE('',(#16338),#6001,.T.) ;
#63624=ADVANCED_FACE('',(#16339),#6002,.T.) ;
#63625=ADVANCED_FACE('',(#16340),#6003,.T.) ;
#63626=ADVANCED_FACE('',(#16341),#6004,.T.) ;
#63627=ADVANCED_FACE('',(#16342),#6005,.T.) ;
#63628=ADVANCED_FACE('',(#16343),#4200,.T.) ;
#63629=ADVANCED_FACE('',(#16344),#62831,.T.) ;
#63630=ADVANCED_FACE('',(#16345),#62832,.T.) ;
#63631=ADVANCED_FACE('',(#16346),#4201,.T.) ;
#63632=ADVANCED_FACE('',(#16347),#6006,.T.) ;
#63633=ADVANCED_FACE('',(#16348),#6007,.F.) ;
#63634=ADVANCED_FACE('',(#16349),#6008,.F.) ;
#63635=ADVANCED_FACE('',(#16350),#6009,.T.) ;
#63636=ADVANCED_FACE('',(#16351),#62833,.T.) ;
#63637=ADVANCED_FACE('',(#16352),#62834,.T.) ;
#63638=ADVANCED_FACE('',(#16353),#6010,.T.) ;
#63639=ADVANCED_FACE('',(#16354),#6011,.T.) ;
#63640=ADVANCED_FACE('',(#16355),#62835,.T.) ;
#63641=ADVANCED_FACE('',(#16356),#6012,.T.) ;
#63642=ADVANCED_FACE('',(#16357),#62836,.T.) ;
#63643=ADVANCED_FACE('',(#16358),#62837,.T.) ;
#63644=ADVANCED_FACE('',(#16359),#6013,.F.) ;
#63645=ADVANCED_FACE('',(#16360),#6014,.T.) ;
#63646=ADVANCED_FACE('',(#16361),#6015,.T.) ;
#63647=ADVANCED_FACE('',(#16362),#6016,.T.) ;
#63648=ADVANCED_FACE('',(#16363),#6017,.F.) ;
#63649=ADVANCED_FACE('',(#16364),#6018,.T.) ;
#63650=ADVANCED_FACE('',(#16365),#62838,.T.) ;
#63651=ADVANCED_FACE('',(#16366),#62839,.T.) ;
#63652=ADVANCED_FACE('',(#16367),#62840,.T.) ;
#63653=ADVANCED_FACE('',(#16368),#62841,.T.) ;
#63654=ADVANCED_FACE('',(#16369),#6019,.T.) ;
#63655=ADVANCED_FACE('',(#16370),#6020,.F.) ;
#63656=ADVANCED_FACE('',(#16371),#6021,.F.) ;
#63657=ADVANCED_FACE('',(#16372),#6022,.T.) ;
#63658=ADVANCED_FACE('',(#16373),#62842,.T.) ;
#63659=ADVANCED_FACE('',(#16374),#62843,.T.) ;
#63660=ADVANCED_FACE('',(#16375),#6023,.T.) ;
#63661=ADVANCED_FACE('',(#16376),#6024,.T.) ;
#63662=ADVANCED_FACE('',(#16377),#62844,.T.) ;
#63663=ADVANCED_FACE('',(#16378),#62845,.T.) ;
#63664=ADVANCED_FACE('',(#16379),#6025,.F.) ;
#63665=ADVANCED_FACE('',(#16380),#6026,.T.) ;
#63666=ADVANCED_FACE('',(#16381),#6027,.T.) ;
#63667=ADVANCED_FACE('',(#16382),#6028,.T.) ;
#63668=ADVANCED_FACE('',(#16383),#6029,.F.) ;
#63669=ADVANCED_FACE('',(#16384),#6030,.T.) ;
#63670=ADVANCED_FACE('',(#16385),#62846,.T.) ;
#63671=ADVANCED_FACE('',(#16386),#62847,.T.) ;
#63672=ADVANCED_FACE('',(#16387),#62848,.T.) ;
#63673=ADVANCED_FACE('',(#16388),#62849,.T.) ;
#63674=ADVANCED_FACE('',(#16389),#6031,.T.) ;
#63675=ADVANCED_FACE('',(#16390),#6032,.F.) ;
#63676=ADVANCED_FACE('',(#16391),#6033,.F.) ;
#63677=ADVANCED_FACE('',(#16392),#6034,.T.) ;
#63678=ADVANCED_FACE('',(#16393),#62850,.T.) ;
#63679=ADVANCED_FACE('',(#16394),#62851,.T.) ;
#63680=ADVANCED_FACE('',(#16395),#6035,.T.) ;
#63681=ADVANCED_FACE('',(#16396),#6036,.T.) ;
#63682=ADVANCED_FACE('',(#16397),#62852,.T.) ;
#63683=ADVANCED_FACE('',(#16398),#62853,.T.) ;
#63684=ADVANCED_FACE('',(#16399),#6037,.F.) ;
#63685=ADVANCED_FACE('',(#16400),#6038,.T.) ;
#63686=ADVANCED_FACE('',(#16401),#6039,.T.) ;
#63687=ADVANCED_FACE('',(#16402),#6040,.T.) ;
#63688=ADVANCED_FACE('',(#16403),#6041,.F.) ;
#63689=ADVANCED_FACE('',(#16404),#6042,.T.) ;
#63690=ADVANCED_FACE('',(#16405),#62854,.T.) ;
#63691=ADVANCED_FACE('',(#16406),#62855,.T.) ;
#63692=ADVANCED_FACE('',(#16407),#62856,.T.) ;
#63693=ADVANCED_FACE('',(#16408),#62857,.T.) ;
#63694=ADVANCED_FACE('',(#16409),#6043,.T.) ;
#63695=ADVANCED_FACE('',(#16410),#6044,.F.) ;
#63696=ADVANCED_FACE('',(#16411),#6045,.F.) ;
#63697=ADVANCED_FACE('',(#16412),#6046,.T.) ;
#63698=ADVANCED_FACE('',(#16413),#62858,.T.) ;
#63699=ADVANCED_FACE('',(#16414),#62859,.T.) ;
#63700=ADVANCED_FACE('',(#16415),#6047,.T.) ;
#63701=ADVANCED_FACE('',(#16416),#6048,.T.) ;
#63702=ADVANCED_FACE('',(#16417),#62860,.T.) ;
#63703=ADVANCED_FACE('',(#16418),#62861,.T.) ;
#63704=ADVANCED_FACE('',(#16419),#6049,.F.) ;
#63705=ADVANCED_FACE('',(#16420),#6050,.T.) ;
#63706=ADVANCED_FACE('',(#16421),#6051,.T.) ;
#63707=ADVANCED_FACE('',(#16422),#6052,.T.) ;
#63708=ADVANCED_FACE('',(#16423),#6053,.F.) ;
#63709=ADVANCED_FACE('',(#16424),#6054,.T.) ;
#63710=ADVANCED_FACE('',(#16425),#62862,.T.) ;
#63711=ADVANCED_FACE('',(#16426),#62863,.T.) ;
#63712=ADVANCED_FACE('',(#16427),#62864,.T.) ;
#63713=ADVANCED_FACE('',(#16428),#62865,.T.) ;
#63714=ADVANCED_FACE('',(#16429),#6055,.T.) ;
#63715=ADVANCED_FACE('',(#16430),#6056,.F.) ;
#63716=ADVANCED_FACE('',(#16431),#6057,.F.) ;
#63717=ADVANCED_FACE('',(#16432),#6058,.T.) ;
#63718=ADVANCED_FACE('',(#16433),#62866,.T.) ;
#63719=ADVANCED_FACE('',(#16434),#62867,.T.) ;
#63720=ADVANCED_FACE('',(#16435),#6059,.T.) ;
#63721=ADVANCED_FACE('',(#16436),#6060,.T.) ;
#63722=ADVANCED_FACE('',(#16437),#62868,.T.) ;
#63723=ADVANCED_FACE('',(#16438),#62869,.T.) ;
#63724=ADVANCED_FACE('',(#16439),#6061,.T.) ;
#63725=ADVANCED_FACE('',(#16440),#6062,.F.) ;
#63726=ADVANCED_FACE('',(#16441),#6063,.T.) ;
#63727=ADVANCED_FACE('',(#16442),#6064,.F.) ;
#63728=ADVANCED_FACE('',(#16443),#6065,.T.) ;
#63729=ADVANCED_FACE('',(#16444),#6066,.T.) ;
#63730=ADVANCED_FACE('',(#16445),#62870,.T.) ;
#63731=ADVANCED_FACE('',(#16446),#62871,.T.) ;
#63732=ADVANCED_FACE('',(#16447),#62872,.T.) ;
#63733=ADVANCED_FACE('',(#16448),#62873,.T.) ;
#63734=ADVANCED_FACE('',(#16449),#6067,.F.) ;
#63735=ADVANCED_FACE('',(#16450),#6068,.T.) ;
#63736=ADVANCED_FACE('',(#16451),#6069,.T.) ;
#63737=ADVANCED_FACE('',(#16452),#6070,.F.) ;
#63738=ADVANCED_FACE('',(#16453),#62874,.T.) ;
#63739=ADVANCED_FACE('',(#16454),#62875,.T.) ;
#63740=ADVANCED_FACE('',(#16455),#6071,.T.) ;
#63741=ADVANCED_FACE('',(#16456),#6072,.T.) ;
#63742=ADVANCED_FACE('',(#16457),#62876,.T.) ;
#63743=ADVANCED_FACE('',(#16458),#62877,.T.) ;
#63744=ADVANCED_FACE('',(#16459),#6073,.F.) ;
#63745=ADVANCED_FACE('',(#16460),#6074,.T.) ;
#63746=ADVANCED_FACE('',(#16461),#6075,.T.) ;
#63747=ADVANCED_FACE('',(#16462),#6076,.T.) ;
#63748=ADVANCED_FACE('',(#16463),#6077,.F.) ;
#63749=ADVANCED_FACE('',(#16464),#6078,.T.) ;
#63750=ADVANCED_FACE('',(#16465),#62878,.T.) ;
#63751=ADVANCED_FACE('',(#16466),#62879,.T.) ;
#63752=ADVANCED_FACE('',(#16467),#62880,.T.) ;
#63753=ADVANCED_FACE('',(#16468),#62881,.T.) ;
#63754=ADVANCED_FACE('',(#16469),#6079,.T.) ;
#63755=ADVANCED_FACE('',(#16470),#6080,.F.) ;
#63756=ADVANCED_FACE('',(#16471),#6081,.F.) ;
#63757=ADVANCED_FACE('',(#16472),#6082,.T.) ;
#63758=ADVANCED_FACE('',(#16473),#62882,.T.) ;
#63759=ADVANCED_FACE('',(#16474),#62883,.T.) ;
#63760=ADVANCED_FACE('',(#16475),#6083,.T.) ;
#63761=ADVANCED_FACE('',(#16476),#6084,.T.) ;
#63762=ADVANCED_FACE('',(#16477),#62884,.T.) ;
#63763=ADVANCED_FACE('',(#16478),#62885,.T.) ;
#63764=ADVANCED_FACE('',(#16479),#6085,.F.) ;
#63765=ADVANCED_FACE('',(#16480),#6086,.T.) ;
#63766=ADVANCED_FACE('',(#16481),#6087,.T.) ;
#63767=ADVANCED_FACE('',(#16482),#6088,.T.) ;
#63768=ADVANCED_FACE('',(#16483),#6089,.F.) ;
#63769=ADVANCED_FACE('',(#16484),#6090,.T.) ;
#63770=ADVANCED_FACE('',(#16485),#62886,.T.) ;
#63771=ADVANCED_FACE('',(#16486),#62887,.T.) ;
#63772=ADVANCED_FACE('',(#16487),#62888,.T.) ;
#63773=ADVANCED_FACE('',(#16488),#62889,.T.) ;
#63774=ADVANCED_FACE('',(#16489),#6091,.T.) ;
#63775=ADVANCED_FACE('',(#16490),#6092,.F.) ;
#63776=ADVANCED_FACE('',(#16491),#6093,.F.) ;
#63777=ADVANCED_FACE('',(#16492),#6094,.T.) ;
#63778=ADVANCED_FACE('',(#16493),#62890,.T.) ;
#63779=ADVANCED_FACE('',(#16494),#62891,.T.) ;
#63780=ADVANCED_FACE('',(#16495),#6095,.T.) ;
#63781=ADVANCED_FACE('',(#16496),#6096,.T.) ;
#63782=ADVANCED_FACE('',(#16497),#62892,.T.) ;
#63783=ADVANCED_FACE('',(#16498),#62893,.T.) ;
#63784=ADVANCED_FACE('',(#16499),#6097,.F.) ;
#63785=ADVANCED_FACE('',(#16500),#6098,.T.) ;
#63786=ADVANCED_FACE('',(#16501),#6099,.T.) ;
#63787=ADVANCED_FACE('',(#16502),#6100,.T.) ;
#63788=ADVANCED_FACE('',(#16503),#6101,.F.) ;
#63789=ADVANCED_FACE('',(#16504),#6102,.T.) ;
#63790=ADVANCED_FACE('',(#16505),#62894,.T.) ;
#63791=ADVANCED_FACE('',(#16506),#62895,.T.) ;
#63792=ADVANCED_FACE('',(#16507),#62896,.T.) ;
#63793=ADVANCED_FACE('',(#16508),#62897,.T.) ;
#63794=ADVANCED_FACE('',(#16509),#6103,.T.) ;
#63795=ADVANCED_FACE('',(#16510),#6104,.F.) ;
#63796=ADVANCED_FACE('',(#16511),#6105,.F.) ;
#63797=ADVANCED_FACE('',(#16512),#6106,.T.) ;
#63798=ADVANCED_FACE('',(#16513),#62898,.T.) ;
#63799=ADVANCED_FACE('',(#16514),#62899,.T.) ;
#63800=ADVANCED_FACE('',(#16515),#6107,.T.) ;
#63801=ADVANCED_FACE('',(#16516),#6108,.T.) ;
#63802=ADVANCED_FACE('',(#16517),#62900,.T.) ;
#63803=ADVANCED_FACE('',(#16518),#62901,.T.) ;
#63804=ADVANCED_FACE('',(#16519),#6109,.F.) ;
#63805=ADVANCED_FACE('',(#16520),#6110,.T.) ;
#63806=ADVANCED_FACE('',(#16521),#6111,.T.) ;
#63807=ADVANCED_FACE('',(#16522),#6112,.T.) ;
#63808=ADVANCED_FACE('',(#16523),#6113,.F.) ;
#63809=ADVANCED_FACE('',(#16524),#6114,.T.) ;
#63810=ADVANCED_FACE('',(#16525),#62902,.T.) ;
#63811=ADVANCED_FACE('',(#16526),#62903,.T.) ;
#63812=ADVANCED_FACE('',(#16527),#62904,.T.) ;
#63813=ADVANCED_FACE('',(#16528),#62905,.T.) ;
#63814=ADVANCED_FACE('',(#16529),#6115,.T.) ;
#63815=ADVANCED_FACE('',(#16530),#6116,.F.) ;
#63816=ADVANCED_FACE('',(#16531),#6117,.F.) ;
#63817=ADVANCED_FACE('',(#16532),#6118,.T.) ;
#63818=ADVANCED_FACE('',(#16533),#62906,.T.) ;
#63819=ADVANCED_FACE('',(#16534),#62907,.T.) ;
#63820=ADVANCED_FACE('',(#16535),#6119,.T.) ;
#63821=ADVANCED_FACE('',(#16536),#6120,.T.) ;
#63822=ADVANCED_FACE('',(#16537),#62908,.T.) ;
#63823=ADVANCED_FACE('',(#16538),#62909,.T.) ;
#63824=ADVANCED_FACE('',(#16539),#6121,.F.) ;
#63825=ADVANCED_FACE('',(#16540),#6122,.T.) ;
#63826=ADVANCED_FACE('',(#16541),#6123,.T.) ;
#63827=ADVANCED_FACE('',(#16542),#6124,.T.) ;
#63828=ADVANCED_FACE('',(#16543),#6125,.F.) ;
#63829=ADVANCED_FACE('',(#16544),#6126,.T.) ;
#63830=ADVANCED_FACE('',(#16545),#62910,.T.) ;
#63831=ADVANCED_FACE('',(#16546),#62911,.T.) ;
#63832=ADVANCED_FACE('',(#16547),#62912,.T.) ;
#63833=ADVANCED_FACE('',(#16548),#62913,.T.) ;
#63834=ADVANCED_FACE('',(#16549),#6127,.T.) ;
#63835=ADVANCED_FACE('',(#16550),#6128,.F.) ;
#63836=ADVANCED_FACE('',(#16551),#6129,.F.) ;
#63837=ADVANCED_FACE('',(#16552),#6130,.T.) ;
#63838=ADVANCED_FACE('',(#16553),#62914,.T.) ;
#63839=ADVANCED_FACE('',(#16554),#62915,.T.) ;
#63840=ADVANCED_FACE('',(#16555),#6131,.T.) ;
#63841=ADVANCED_FACE('',(#16556),#6132,.T.) ;
#63842=ADVANCED_FACE('',(#16557),#62916,.T.) ;
#63843=ADVANCED_FACE('',(#16558),#62917,.T.) ;
#63844=ADVANCED_FACE('',(#16559),#6133,.F.) ;
#63845=ADVANCED_FACE('',(#16560),#6134,.T.) ;
#63846=ADVANCED_FACE('',(#16561),#6135,.T.) ;
#63847=ADVANCED_FACE('',(#16562),#6136,.T.) ;
#63848=ADVANCED_FACE('',(#16563),#6137,.F.) ;
#63849=ADVANCED_FACE('',(#16564),#6138,.T.) ;
#63850=ADVANCED_FACE('',(#16565),#62918,.T.) ;
#63851=ADVANCED_FACE('',(#16566),#62919,.T.) ;
#63852=ADVANCED_FACE('',(#16567),#62920,.T.) ;
#63853=ADVANCED_FACE('',(#16568),#62921,.T.) ;
#63854=ADVANCED_FACE('',(#16569),#6139,.T.) ;
#63855=ADVANCED_FACE('',(#16570),#6140,.F.) ;
#63856=ADVANCED_FACE('',(#16571),#6141,.F.) ;
#63857=ADVANCED_FACE('',(#16572),#6142,.T.) ;
#63858=ADVANCED_FACE('',(#16573),#62922,.T.) ;
#63859=ADVANCED_FACE('',(#16574),#62923,.T.) ;
#63860=ADVANCED_FACE('',(#16575),#6143,.T.) ;
#63861=ADVANCED_FACE('',(#16576),#6144,.T.) ;
#63862=ADVANCED_FACE('',(#16577),#62924,.T.) ;
#63863=ADVANCED_FACE('',(#16578),#62925,.T.) ;
#63864=ADVANCED_FACE('',(#16579),#6145,.F.) ;
#63865=ADVANCED_FACE('',(#16580),#6146,.T.) ;
#63866=ADVANCED_FACE('',(#16581),#6147,.T.) ;
#63867=ADVANCED_FACE('',(#16582),#6148,.T.) ;
#63868=ADVANCED_FACE('',(#16583),#6149,.F.) ;
#63869=ADVANCED_FACE('',(#16584),#6150,.T.) ;
#63870=ADVANCED_FACE('',(#16585),#62926,.T.) ;
#63871=ADVANCED_FACE('',(#16586),#62927,.T.) ;
#63872=ADVANCED_FACE('',(#16587),#62928,.T.) ;
#63873=ADVANCED_FACE('',(#16588),#62929,.T.) ;
#63874=ADVANCED_FACE('',(#16589),#6151,.T.) ;
#63875=ADVANCED_FACE('',(#16590),#6152,.F.) ;
#63876=ADVANCED_FACE('',(#16591),#6153,.F.) ;
#63877=ADVANCED_FACE('',(#16592),#6154,.T.) ;
#63878=ADVANCED_FACE('',(#16593),#62930,.T.) ;
#63879=ADVANCED_FACE('',(#16594),#62931,.T.) ;
#63880=ADVANCED_FACE('',(#16595),#6155,.T.) ;
#63881=ADVANCED_FACE('',(#16596),#6156,.T.) ;
#63882=ADVANCED_FACE('',(#16597),#6157,.T.) ;
#63883=ADVANCED_FACE('',(#16598),#6158,.T.) ;
#63884=ADVANCED_FACE('',(#16599),#4202,.T.) ;
#63885=ADVANCED_FACE('',(#16600),#6159,.T.) ;
#63886=ADVANCED_FACE('',(#16601),#6160,.T.) ;
#63887=ADVANCED_FACE('',(#16602),#4203,.T.) ;
#63888=ADVANCED_FACE('',(#16603),#6161,.T.) ;
#63889=ADVANCED_FACE('',(#16604),#6162,.T.) ;
#63890=ADVANCED_FACE('',(#16605),#6163,.T.) ;
#63891=ADVANCED_FACE('',(#16606),#6164,.T.) ;
#63892=ADVANCED_FACE('',(#16607),#4204,.T.) ;
#63893=ADVANCED_FACE('',(#16608),#4205,.T.) ;
#63894=ADVANCED_FACE('',(#16609),#6165,.T.) ;
#67686=CLOSED_SHELL('',(#63444,#63445,#63446,#63447,#63448,#63449,#63450,
#63451,#63452,#63453,#63454,#63455,#63456,#63457,#63458,#63459,#63460,#63461,
#63462,#63463,#63464,#63465,#63466,#63467,#63468,#63469,#63470,#63471,#63472,
#63473,#63474,#63475,#63476,#63477,#63478,#63479,#63480,#63481,#63482,#63483,
#63484,#63485,#63486,#63487,#63488,#63489,#63490,#63491,#63492,#63493,#63494,
#63495,#63496,#63497,#63498,#63499,#63500,#63501,#63502,#63503,#63504,#63505,
#63506,#63507,#63508,#63509,#63510,#63511,#63512,#63513,#63514,#63515,#63516,
#63517,#63518,#63519,#63520,#63521,#63522,#63523,#63524,#63525,#63526,#63527,
#63528,#63529,#63530,#63531,#63532,#63533,#63534,#63535,#63536,#63537,#63538,
#63539,#63540,#63541,#63542,#63543,#63544,#63545,#63546,#63547,#63548,#63549,
#63550,#63551,#63552,#63553,#63554,#63555,#63556,#63557,#63558,#63559,#63560,
#63561,#63562,#63563,#63564,#63565,#63566,#63567,#63568,#63569,#63570,#63571,
#63572,#63573,#63574,#63575,#63576,#63577,#63578,#63579,#63580,#63581,#63582,
#63583,#63584,#63585,#63586,#63587,#63588,#63589,#63590,#63591,#63592,#63593,
#63594,#63595,#63596,#63597,#63598,#63599,#63600,#63601,#63602,#63603,#63604,
#63605,#63606,#63607,#63608,#63609,#63610,#63611,#63612,#63613,#63614,#63615,
#63616,#63617,#63618,#63619,#63620,#63621,#63622,#63623,#63624,#63625,#63626,
#63627,#63628,#63629,#63630,#63631,#63632,#63633,#63634,#63635,#63636,#63637,
#63638,#63639,#63640,#63641,#63642,#63643,#63644,#63645,#63646,#63647,#63648,
#63649,#63650,#63651,#63652,#63653,#63654,#63655,#63656,#63657,#63658,#63659,
#63660,#63661,#63662,#63663,#63664,#63665,#63666,#63667,#63668,#63669,#63670,
#63671,#63672,#63673,#63674,#63675,#63676,#63677,#63678,#63679,#63680,#63681,
#63682,#63683,#63684,#63685,#63686,#63687,#63688,#63689,#63690,#63691,#63692,
#63693,#63694,#63695,#63696,#63697,#63698,#63699,#63700,#63701,#63702,#63703,
#63704,#63705,#63706,#63707,#63708,#63709,#63710,#63711,#63712,#63713,#63714,
#63715,#63716,#63717,#63718,#63719,#63720,#63721,#63722,#63723,#63724,#63725,
#63726,#63727,#63728,#63729,#63730,#63731,#63732,#63733,#63734,#63735,#63736,
#63737,#63738,#63739,#63740,#63741,#63742,#63743,#63744,#63745,#63746,#63747,
#63748,#63749,#63750,#63751,#63752,#63753,#63754,#63755,#63756,#63757,#63758,
#63759,#63760,#63761,#63762,#63763,#63764,#63765,#63766,#63767,#63768,#63769,
#63770,#63771,#63772,#63773,#63774,#63775,#63776,#63777,#63778,#63779,#63780,
#63781,#63782,#63783,#63784,#63785,#63786,#63787,#63788,#63789,#63790,#63791,
#63792,#63793,#63794,#63795,#63796,#63797,#63798,#63799,#63800,#63801,#63802,
#63803,#63804,#63805,#63806,#63807,#63808,#63809,#63810,#63811,#63812,#63813,
#63814,#63815,#63816,#63817,#63818,#63819,#63820,#63821,#63822,#63823,#63824,
#63825,#63826,#63827,#63828,#63829,#63830,#63831,#63832,#63833,#63834,#63835,
#63836,#63837,#63838,#63839,#63840,#63841,#63842,#63843,#63844,#63845,#63846,
#63847,#63848,#63849,#63850,#63851,#63852,#63853,#63854,#63855,#63856,#63857,
#63858,#63859,#63860,#63861,#63862,#63863,#63864,#63865,#63866,#63867,#63868,
#63869,#63870,#63871,#63872,#63873,#63874,#63875,#63876,#63877,#63878,#63879,
#63880,#63881,#63882,#63883,#63884,#63885,#63886,#63887,#63888,#63889,#63890,
#63891,#63892,#63893,#63894)) ;
#67764=AXIS2_PLACEMENT_3D('',#99147,#76854,#76855) ;
#67765=AXIS2_PLACEMENT_3D('',#99148,#76856,#76857) ;
#67766=AXIS2_PLACEMENT_3D('',#99151,#76858,#76859) ;
#67767=AXIS2_PLACEMENT_3D('',#99152,#76860,#76861) ;
#67768=AXIS2_PLACEMENT_3D('',#99154,#76862,#76863) ;
#67769=AXIS2_PLACEMENT_3D('',#99155,#76864,#76865) ;
#67770=AXIS2_PLACEMENT_3D('',#99156,#76866,#76867) ;
#67771=AXIS2_PLACEMENT_3D('',#99158,#76868,#76869) ;
#67772=AXIS2_PLACEMENT_3D('',#99160,#76870,#76871) ;
#67773=AXIS2_PLACEMENT_3D('',#99162,#76872,#76873) ;
#67774=AXIS2_PLACEMENT_3D('',#99163,#76874,#76875) ;
#67775=AXIS2_PLACEMENT_3D('',#99164,#76876,#76877) ;
#67776=AXIS2_PLACEMENT_3D('',#99167,#76878,#76879) ;
#67777=AXIS2_PLACEMENT_3D('',#99168,#76880,#76881) ;
#67778=AXIS2_PLACEMENT_3D('',#99170,#76882,#76883) ;
#67779=AXIS2_PLACEMENT_3D('',#99172,#76884,#76885) ;
#67780=AXIS2_PLACEMENT_3D('',#99173,#76886,#76887) ;
#67781=AXIS2_PLACEMENT_3D('',#99174,#76888,#76889) ;
#67782=AXIS2_PLACEMENT_3D('',#99176,#76890,#76891) ;
#67783=AXIS2_PLACEMENT_3D('',#99178,#76892,#76893) ;
#67784=AXIS2_PLACEMENT_3D('',#99179,#76894,#76895) ;
#67785=AXIS2_PLACEMENT_3D('',#99180,#76896,#76897) ;
#67786=AXIS2_PLACEMENT_3D('',#99183,#76898,#76899) ;
#67787=AXIS2_PLACEMENT_3D('',#99184,#76900,#76901) ;
#67788=AXIS2_PLACEMENT_3D('',#99186,#76902,#76903) ;
#67789=AXIS2_PLACEMENT_3D('',#99188,#76904,#76905) ;
#67790=AXIS2_PLACEMENT_3D('',#99189,#76906,#76907) ;
#67791=AXIS2_PLACEMENT_3D('',#99190,#76908,#76909) ;
#67792=AXIS2_PLACEMENT_3D('',#99192,#76910,#76911) ;
#67793=AXIS2_PLACEMENT_3D('',#99194,#76912,#76913) ;
#67794=AXIS2_PLACEMENT_3D('',#99195,#76914,#76915) ;
#67795=AXIS2_PLACEMENT_3D('',#99196,#76916,#76917) ;
#67796=AXIS2_PLACEMENT_3D('',#99199,#76919,#76920) ;
#67797=AXIS2_PLACEMENT_3D('',#99200,#76921,#76922) ;
#67798=AXIS2_PLACEMENT_3D('',#99202,#76924,#76925) ;
#67799=AXIS2_PLACEMENT_3D('',#99205,#76927,#76928) ;
#67800=AXIS2_PLACEMENT_3D('',#99206,#76929,#76930) ;
#67801=AXIS2_PLACEMENT_3D('',#99208,#76932,#76933) ;
#67802=AXIS2_PLACEMENT_3D('',#99210,#76935,#76936) ;
#67803=AXIS2_PLACEMENT_3D('',#99225,#76943,#76944) ;
#67804=AXIS2_PLACEMENT_3D('',#99229,#76946,#76947) ;
#67805=AXIS2_PLACEMENT_3D('',#99233,#76949,#76950) ;
#67806=AXIS2_PLACEMENT_3D('',#99237,#76952,#76953) ;
#67807=AXIS2_PLACEMENT_3D('',#99239,#76955,#76956) ;
#67808=AXIS2_PLACEMENT_3D('',#99254,#76963,#76964) ;
#67809=AXIS2_PLACEMENT_3D('',#99258,#76966,#76967) ;
#67810=AXIS2_PLACEMENT_3D('',#99262,#76969,#76970) ;
#67811=AXIS2_PLACEMENT_3D('',#99266,#76972,#76973) ;
#67812=AXIS2_PLACEMENT_3D('',#99268,#76975,#76976) ;
#67813=AXIS2_PLACEMENT_3D('',#99271,#76977,#76978) ;
#67814=AXIS2_PLACEMENT_3D('',#99285,#76985,#76986) ;
#67815=AXIS2_PLACEMENT_3D('',#99293,#76990,#76991) ;
#67816=AXIS2_PLACEMENT_3D('',#99297,#76993,#76994) ;
#67817=AXIS2_PLACEMENT_3D('',#99301,#76996,#76997) ;
#67818=AXIS2_PLACEMENT_3D('',#99305,#76999,#77000) ;
#67819=AXIS2_PLACEMENT_3D('',#99309,#77002,#77003) ;
#67820=AXIS2_PLACEMENT_3D('',#99313,#77005,#77006) ;
#67821=AXIS2_PLACEMENT_3D('',#99317,#77008,#77009) ;
#67822=AXIS2_PLACEMENT_3D('',#99321,#77011,#77012) ;
#67823=AXIS2_PLACEMENT_3D('',#99325,#77014,#77015) ;
#67824=AXIS2_PLACEMENT_3D('',#99329,#77017,#77018) ;
#67825=AXIS2_PLACEMENT_3D('',#99333,#77020,#77021) ;
#67826=AXIS2_PLACEMENT_3D('',#99337,#77023,#77024) ;
#67827=AXIS2_PLACEMENT_3D('',#99341,#77026,#77027) ;
#67828=AXIS2_PLACEMENT_3D('',#99345,#77029,#77030) ;
#67829=AXIS2_PLACEMENT_3D('',#99349,#77032,#77033) ;
#67830=AXIS2_PLACEMENT_3D('',#99353,#77035,#77036) ;
#67831=AXIS2_PLACEMENT_3D('',#99355,#77038,#77039) ;
#67832=AXIS2_PLACEMENT_3D('',#99362,#77042,#77043) ;
#67833=AXIS2_PLACEMENT_3D('',#99370,#77047,#77048) ;
#67834=AXIS2_PLACEMENT_3D('',#99380,#77053,#77054) ;
#67835=AXIS2_PLACEMENT_3D('',#99384,#77056,#77057) ;
#67836=AXIS2_PLACEMENT_3D('',#99388,#77059,#77060) ;
#67837=AXIS2_PLACEMENT_3D('',#99392,#77062,#77063) ;
#67838=AXIS2_PLACEMENT_3D('',#99396,#77065,#77066) ;
#67839=AXIS2_PLACEMENT_3D('',#99400,#77068,#77069) ;
#67840=AXIS2_PLACEMENT_3D('',#99404,#77071,#77072) ;
#67841=AXIS2_PLACEMENT_3D('',#99408,#77074,#77075) ;
#67842=AXIS2_PLACEMENT_3D('',#99412,#77077,#77078) ;
#67843=AXIS2_PLACEMENT_3D('',#99416,#77080,#77081) ;
#67844=AXIS2_PLACEMENT_3D('',#99420,#77083,#77084) ;
#67845=AXIS2_PLACEMENT_3D('',#99424,#77086,#77087) ;
#67846=AXIS2_PLACEMENT_3D('',#99428,#77089,#77090) ;
#67847=AXIS2_PLACEMENT_3D('',#99432,#77092,#77093) ;
#67848=AXIS2_PLACEMENT_3D('',#99436,#77095,#77096) ;
#67849=AXIS2_PLACEMENT_3D('',#99440,#77098,#77099) ;
#67850=AXIS2_PLACEMENT_3D('',#99442,#77101,#77102) ;
#67851=AXIS2_PLACEMENT_3D('',#99449,#77105,#77106) ;
#67852=AXIS2_PLACEMENT_3D('',#99457,#77110,#77111) ;
#67853=AXIS2_PLACEMENT_3D('',#99467,#77116,#77117) ;
#67854=AXIS2_PLACEMENT_3D('',#99471,#77119,#77120) ;
#67855=AXIS2_PLACEMENT_3D('',#99475,#77122,#77123) ;
#67856=AXIS2_PLACEMENT_3D('',#99479,#77125,#77126) ;
#67857=AXIS2_PLACEMENT_3D('',#99483,#77128,#77129) ;
#67858=AXIS2_PLACEMENT_3D('',#99487,#77131,#77132) ;
#67859=AXIS2_PLACEMENT_3D('',#99491,#77134,#77135) ;
#67860=AXIS2_PLACEMENT_3D('',#99495,#77137,#77138) ;
#67861=AXIS2_PLACEMENT_3D('',#99499,#77140,#77141) ;
#67862=AXIS2_PLACEMENT_3D('',#99503,#77143,#77144) ;
#67863=AXIS2_PLACEMENT_3D('',#99507,#77146,#77147) ;
#67864=AXIS2_PLACEMENT_3D('',#99511,#77149,#77150) ;
#67865=AXIS2_PLACEMENT_3D('',#99515,#77152,#77153) ;
#67866=AXIS2_PLACEMENT_3D('',#99519,#77155,#77156) ;
#67867=AXIS2_PLACEMENT_3D('',#99523,#77158,#77159) ;
#67868=AXIS2_PLACEMENT_3D('',#99527,#77161,#77162) ;
#67869=AXIS2_PLACEMENT_3D('',#99531,#77164,#77165) ;
#67870=AXIS2_PLACEMENT_3D('',#99535,#77167,#77168) ;
#67871=AXIS2_PLACEMENT_3D('',#99539,#77170,#77171) ;
#67872=AXIS2_PLACEMENT_3D('',#99543,#77173,#77174) ;
#67873=AXIS2_PLACEMENT_3D('',#99547,#77176,#77177) ;
#67874=AXIS2_PLACEMENT_3D('',#99551,#77179,#77180) ;
#67875=AXIS2_PLACEMENT_3D('',#99555,#77182,#77183) ;
#67876=AXIS2_PLACEMENT_3D('',#99559,#77185,#77186) ;
#67877=AXIS2_PLACEMENT_3D('',#99563,#77188,#77189) ;
#67878=AXIS2_PLACEMENT_3D('',#99567,#77191,#77192) ;
#67879=AXIS2_PLACEMENT_3D('',#99571,#77194,#77195) ;
#67880=AXIS2_PLACEMENT_3D('',#99575,#77197,#77198) ;
#67881=AXIS2_PLACEMENT_3D('',#99577,#77200,#77201) ;
#67882=AXIS2_PLACEMENT_3D('',#99580,#77202,#77203) ;
#67883=AXIS2_PLACEMENT_3D('',#99594,#77210,#77211) ;
#67884=AXIS2_PLACEMENT_3D('',#99602,#77215,#77216) ;
#67885=AXIS2_PLACEMENT_3D('',#99606,#77218,#77219) ;
#67886=AXIS2_PLACEMENT_3D('',#99610,#77221,#77222) ;
#67887=AXIS2_PLACEMENT_3D('',#99614,#77224,#77225) ;
#67888=AXIS2_PLACEMENT_3D('',#99618,#77227,#77228) ;
#67889=AXIS2_PLACEMENT_3D('',#99622,#77230,#77231) ;
#67890=AXIS2_PLACEMENT_3D('',#99626,#77233,#77234) ;
#67891=AXIS2_PLACEMENT_3D('',#99630,#77236,#77237) ;
#67892=AXIS2_PLACEMENT_3D('',#99634,#77239,#77240) ;
#67893=AXIS2_PLACEMENT_3D('',#99638,#77242,#77243) ;
#67894=AXIS2_PLACEMENT_3D('',#99642,#77245,#77246) ;
#67895=AXIS2_PLACEMENT_3D('',#99646,#77248,#77249) ;
#67896=AXIS2_PLACEMENT_3D('',#99650,#77251,#77252) ;
#67897=AXIS2_PLACEMENT_3D('',#99654,#77254,#77255) ;
#67898=AXIS2_PLACEMENT_3D('',#99658,#77257,#77258) ;
#67899=AXIS2_PLACEMENT_3D('',#99662,#77260,#77261) ;
#67900=AXIS2_PLACEMENT_3D('',#99666,#77263,#77264) ;
#67901=AXIS2_PLACEMENT_3D('',#99670,#77266,#77267) ;
#67902=AXIS2_PLACEMENT_3D('',#99674,#77269,#77270) ;
#67903=AXIS2_PLACEMENT_3D('',#99678,#77272,#77273) ;
#67904=AXIS2_PLACEMENT_3D('',#99682,#77275,#77276) ;
#67905=AXIS2_PLACEMENT_3D('',#99686,#77278,#77279) ;
#67906=AXIS2_PLACEMENT_3D('',#99690,#77281,#77282) ;
#67907=AXIS2_PLACEMENT_3D('',#99694,#77284,#77285) ;
#67908=AXIS2_PLACEMENT_3D('',#99698,#77287,#77288) ;
#67909=AXIS2_PLACEMENT_3D('',#99702,#77290,#77291) ;
#67910=AXIS2_PLACEMENT_3D('',#99706,#77293,#77294) ;
#67911=AXIS2_PLACEMENT_3D('',#99710,#77296,#77297) ;
#67912=AXIS2_PLACEMENT_3D('',#99712,#77299,#77300) ;
#67913=AXIS2_PLACEMENT_3D('',#99715,#77301,#77302) ;
#67914=AXIS2_PLACEMENT_3D('',#99727,#77308,#77309) ;
#67915=AXIS2_PLACEMENT_3D('',#99733,#77313,#77314) ;
#67916=AXIS2_PLACEMENT_3D('',#99740,#77317,#77318) ;
#67917=AXIS2_PLACEMENT_3D('',#99748,#77322,#77323) ;
#67918=AXIS2_PLACEMENT_3D('',#99754,#77327,#77328) ;
#67919=AXIS2_PLACEMENT_3D('',#99763,#77333,#77334) ;
#67920=AXIS2_PLACEMENT_3D('',#99772,#77339,#77340) ;
#67921=AXIS2_PLACEMENT_3D('',#99781,#77345,#77346) ;
#67922=AXIS2_PLACEMENT_3D('',#99790,#77351,#77352) ;
#67923=AXIS2_PLACEMENT_3D('',#99799,#77357,#77358) ;
#67924=AXIS2_PLACEMENT_3D('',#99801,#77359,#77360) ;
#67925=AXIS2_PLACEMENT_3D('',#99804,#77362,#77363) ;
#67926=AXIS2_PLACEMENT_3D('',#99805,#77364,#77365) ;
#67927=AXIS2_PLACEMENT_3D('',#99806,#77366,#77367) ;
#67928=AXIS2_PLACEMENT_3D('',#99808,#77369,#77370) ;
#67929=AXIS2_PLACEMENT_3D('',#99810,#77372,#77373) ;
#67930=AXIS2_PLACEMENT_3D('',#99811,#77374,#77375) ;
#67931=AXIS2_PLACEMENT_3D('',#99812,#77376,#77377) ;
#67932=AXIS2_PLACEMENT_3D('',#99813,#77378,#77379) ;
#67933=AXIS2_PLACEMENT_3D('',#99814,#77380,#77381) ;
#67934=AXIS2_PLACEMENT_3D('',#99823,#77386,#77387) ;
#67935=AXIS2_PLACEMENT_3D('',#99832,#77392,#77393) ;
#67936=AXIS2_PLACEMENT_3D('',#99841,#77398,#77399) ;
#67937=AXIS2_PLACEMENT_3D('',#99850,#77404,#77405) ;
#67938=AXIS2_PLACEMENT_3D('',#99859,#77410,#77411) ;
#67939=AXIS2_PLACEMENT_3D('',#99868,#77416,#77417) ;
#67940=AXIS2_PLACEMENT_3D('',#99874,#77421,#77422) ;
#67941=AXIS2_PLACEMENT_3D('',#99876,#77424,#77425) ;
#67942=AXIS2_PLACEMENT_3D('',#99885,#77430,#77431) ;
#67943=AXIS2_PLACEMENT_3D('',#99894,#77436,#77437) ;
#67944=AXIS2_PLACEMENT_3D('',#99903,#77442,#77443) ;
#67945=AXIS2_PLACEMENT_3D('',#99906,#77446,#77447) ;
#67946=AXIS2_PLACEMENT_3D('',#99909,#77450,#77451) ;
#67947=AXIS2_PLACEMENT_3D('',#99910,#77452,#77453) ;
#67948=AXIS2_PLACEMENT_3D('',#99912,#77455,#77456) ;
#67949=AXIS2_PLACEMENT_3D('',#99913,#77457,#77458) ;
#67950=AXIS2_PLACEMENT_3D('',#99914,#77459,#77460) ;
#67951=AXIS2_PLACEMENT_3D('',#99915,#77461,#77462) ;
#67952=AXIS2_PLACEMENT_3D('',#99916,#77463,#77464) ;
#67953=AXIS2_PLACEMENT_3D('',#99917,#77465,#77466) ;
#67954=AXIS2_PLACEMENT_3D('',#99918,#77467,#77468) ;
#67955=AXIS2_PLACEMENT_3D('',#99922,#77470,#77471) ;
#67956=AXIS2_PLACEMENT_3D('',#99923,#77472,#77473) ;
#67957=AXIS2_PLACEMENT_3D('',#99924,#77474,#77475) ;
#67958=AXIS2_PLACEMENT_3D('',#99925,#77476,#77477) ;
#67959=AXIS2_PLACEMENT_3D('',#99927,#77479,#77480) ;
#67960=AXIS2_PLACEMENT_3D('',#99928,#77481,#77482) ;
#67961=AXIS2_PLACEMENT_3D('',#99929,#77483,#77484) ;
#67962=AXIS2_PLACEMENT_3D('',#99930,#77485,#77486) ;
#67963=AXIS2_PLACEMENT_3D('',#99931,#77487,#77488) ;
#67964=AXIS2_PLACEMENT_3D('',#99932,#77489,#77490) ;
#67965=AXIS2_PLACEMENT_3D('',#99941,#77495,#77496) ;
#67966=AXIS2_PLACEMENT_3D('',#99950,#77501,#77502) ;
#67967=AXIS2_PLACEMENT_3D('',#99959,#77507,#77508) ;
#67968=AXIS2_PLACEMENT_3D('',#99968,#77513,#77514) ;
#67969=AXIS2_PLACEMENT_3D('',#99977,#77519,#77520) ;
#67970=AXIS2_PLACEMENT_3D('',#99986,#77525,#77526) ;
#67971=AXIS2_PLACEMENT_3D('',#99988,#77528,#77529) ;
#67972=AXIS2_PLACEMENT_3D('',#99994,#77533,#77534) ;
#67973=AXIS2_PLACEMENT_3D('',#100003,#77539,#77540) ;
#67974=AXIS2_PLACEMENT_3D('',#100012,#77545,#77546) ;
#67975=AXIS2_PLACEMENT_3D('',#100021,#77551,#77552) ;
#67976=AXIS2_PLACEMENT_3D('',#100030,#77557,#77558) ;
#67977=AXIS2_PLACEMENT_3D('',#100039,#77563,#77564) ;
#67978=AXIS2_PLACEMENT_3D('',#100048,#77569,#77570) ;
#67979=AXIS2_PLACEMENT_3D('',#100057,#77575,#77576) ;
#67980=AXIS2_PLACEMENT_3D('',#100066,#77581,#77582) ;
#67981=AXIS2_PLACEMENT_3D('',#100075,#77587,#77588) ;
#67982=AXIS2_PLACEMENT_3D('',#100084,#77593,#77594) ;
#67983=AXIS2_PLACEMENT_3D('',#100093,#77599,#77600) ;
#67984=AXIS2_PLACEMENT_3D('',#100102,#77605,#77606) ;
#67985=AXIS2_PLACEMENT_3D('',#100111,#77611,#77612) ;
#67986=AXIS2_PLACEMENT_3D('',#100120,#77617,#77618) ;
#67987=AXIS2_PLACEMENT_3D('',#100129,#77623,#77624) ;
#67988=AXIS2_PLACEMENT_3D('',#100138,#77629,#77630) ;
#67989=AXIS2_PLACEMENT_3D('',#100147,#77635,#77636) ;
#67990=AXIS2_PLACEMENT_3D('',#100156,#77641,#77642) ;
#67991=AXIS2_PLACEMENT_3D('',#100165,#77647,#77648) ;
#67992=AXIS2_PLACEMENT_3D('',#100174,#77653,#77654) ;
#67993=AXIS2_PLACEMENT_3D('',#100183,#77659,#77660) ;
#67994=AXIS2_PLACEMENT_3D('',#100192,#77665,#77666) ;
#67995=AXIS2_PLACEMENT_3D('',#100201,#77671,#77672) ;
#67996=AXIS2_PLACEMENT_3D('',#100210,#77677,#77678) ;
#67997=AXIS2_PLACEMENT_3D('',#100219,#77683,#77684) ;
#67998=AXIS2_PLACEMENT_3D('',#100228,#77689,#77690) ;
#67999=AXIS2_PLACEMENT_3D('',#100237,#77695,#77696) ;
#68000=AXIS2_PLACEMENT_3D('',#100246,#77701,#77702) ;
#68001=AXIS2_PLACEMENT_3D('',#100255,#77707,#77708) ;
#68002=AXIS2_PLACEMENT_3D('',#100264,#77713,#77714) ;
#68003=AXIS2_PLACEMENT_3D('',#100273,#77719,#77720) ;
#68004=AXIS2_PLACEMENT_3D('',#100282,#77725,#77726) ;
#68005=AXIS2_PLACEMENT_3D('',#100291,#77731,#77732) ;
#68006=AXIS2_PLACEMENT_3D('',#100300,#77737,#77738) ;
#68007=AXIS2_PLACEMENT_3D('',#100309,#77743,#77744) ;
#68008=AXIS2_PLACEMENT_3D('',#100318,#77749,#77750) ;
#68009=AXIS2_PLACEMENT_3D('',#100327,#77755,#77756) ;
#68010=AXIS2_PLACEMENT_3D('',#100336,#77761,#77762) ;
#68011=AXIS2_PLACEMENT_3D('',#100345,#77767,#77768) ;
#68012=AXIS2_PLACEMENT_3D('',#100354,#77773,#77774) ;
#68013=AXIS2_PLACEMENT_3D('',#100363,#77779,#77780) ;
#68014=AXIS2_PLACEMENT_3D('',#100372,#77785,#77786) ;
#68015=AXIS2_PLACEMENT_3D('',#100381,#77791,#77792) ;
#68016=AXIS2_PLACEMENT_3D('',#100390,#77797,#77798) ;
#68017=AXIS2_PLACEMENT_3D('',#100399,#77803,#77804) ;
#68018=AXIS2_PLACEMENT_3D('',#100408,#77809,#77810) ;
#68019=AXIS2_PLACEMENT_3D('',#100417,#77815,#77816) ;
#68020=AXIS2_PLACEMENT_3D('',#100426,#77821,#77822) ;
#68021=AXIS2_PLACEMENT_3D('',#100427,#77823,#77824) ;
#68022=AXIS2_PLACEMENT_3D('',#100428,#77825,#77826) ;
#68023=AXIS2_PLACEMENT_3D('',#100429,#77827,#77828) ;
#68024=AXIS2_PLACEMENT_3D('',#100430,#77829,#77830) ;
#68025=AXIS2_PLACEMENT_3D('',#100431,#77831,#77832) ;
#68026=AXIS2_PLACEMENT_3D('',#100432,#77833,#77834) ;
#68027=AXIS2_PLACEMENT_3D('',#100433,#77835,#77836) ;
#68028=AXIS2_PLACEMENT_3D('',#100434,#77837,#77838) ;
#68029=AXIS2_PLACEMENT_3D('',#100435,#77839,#77840) ;
#68030=AXIS2_PLACEMENT_3D('',#100436,#77841,#77842) ;
#68031=AXIS2_PLACEMENT_3D('',#100437,#77843,#77844) ;
#68032=AXIS2_PLACEMENT_3D('',#100438,#77845,#77846) ;
#68033=AXIS2_PLACEMENT_3D('',#100439,#77847,#77848) ;
#68034=AXIS2_PLACEMENT_3D('',#100440,#77849,#77850) ;
#68035=AXIS2_PLACEMENT_3D('',#100441,#77851,#77852) ;
#68036=AXIS2_PLACEMENT_3D('',#100442,#77853,#77854) ;
#68037=AXIS2_PLACEMENT_3D('',#100443,#77855,#77856) ;
#68038=AXIS2_PLACEMENT_3D('',#100444,#77857,#77858) ;
#68039=AXIS2_PLACEMENT_3D('',#100445,#77859,#77860) ;
#68040=AXIS2_PLACEMENT_3D('',#100446,#77861,#77862) ;
#68041=AXIS2_PLACEMENT_3D('',#100447,#77863,#77864) ;
#68042=AXIS2_PLACEMENT_3D('',#100448,#77865,#77866) ;
#68043=AXIS2_PLACEMENT_3D('',#100449,#77867,#77868) ;
#68044=AXIS2_PLACEMENT_3D('',#100450,#77869,#77870) ;
#68045=AXIS2_PLACEMENT_3D('',#100451,#77871,#77872) ;
#68046=AXIS2_PLACEMENT_3D('',#100452,#77873,#77874) ;
#68047=AXIS2_PLACEMENT_3D('',#100453,#77875,#77876) ;
#68048=AXIS2_PLACEMENT_3D('',#100454,#77877,#77878) ;
#68049=AXIS2_PLACEMENT_3D('',#100455,#77879,#77880) ;
#68050=AXIS2_PLACEMENT_3D('',#100456,#77881,#77882) ;
#68051=AXIS2_PLACEMENT_3D('',#100457,#77883,#77884) ;
#68052=AXIS2_PLACEMENT_3D('',#100458,#77885,#77886) ;
#68053=AXIS2_PLACEMENT_3D('',#100459,#77887,#77888) ;
#68054=AXIS2_PLACEMENT_3D('',#100460,#77889,#77890) ;
#68055=AXIS2_PLACEMENT_3D('',#100461,#77891,#77892) ;
#68056=AXIS2_PLACEMENT_3D('',#100462,#77893,#77894) ;
#68057=AXIS2_PLACEMENT_3D('',#100463,#77895,#77896) ;
#68058=AXIS2_PLACEMENT_3D('',#100464,#77897,#77898) ;
#68059=AXIS2_PLACEMENT_3D('',#100465,#77899,#77900) ;
#68060=AXIS2_PLACEMENT_3D('',#100466,#77901,#77902) ;
#68061=AXIS2_PLACEMENT_3D('',#100467,#77903,#77904) ;
#68062=AXIS2_PLACEMENT_3D('',#100468,#77905,#77906) ;
#68063=AXIS2_PLACEMENT_3D('',#100469,#77907,#77908) ;
#68064=AXIS2_PLACEMENT_3D('',#100470,#77909,#77910) ;
#68065=AXIS2_PLACEMENT_3D('',#100471,#77911,#77912) ;
#68066=AXIS2_PLACEMENT_3D('',#100472,#77913,#77914) ;
#68067=AXIS2_PLACEMENT_3D('',#100473,#77915,#77916) ;
#68068=AXIS2_PLACEMENT_3D('',#100474,#77917,#77918) ;
#68069=AXIS2_PLACEMENT_3D('',#100475,#77919,#77920) ;
#68070=AXIS2_PLACEMENT_3D('',#100476,#77921,#77922) ;
#68071=AXIS2_PLACEMENT_3D('',#100477,#77923,#77924) ;
#68072=AXIS2_PLACEMENT_3D('',#100478,#77925,#77926) ;
#68073=AXIS2_PLACEMENT_3D('',#100479,#77927,#77928) ;
#68074=AXIS2_PLACEMENT_3D('',#100480,#77929,#77930) ;
#68075=AXIS2_PLACEMENT_3D('',#100481,#77931,#77932) ;
#68076=AXIS2_PLACEMENT_3D('',#100482,#77933,#77934) ;
#68077=AXIS2_PLACEMENT_3D('',#100483,#77935,#77936) ;
#68078=AXIS2_PLACEMENT_3D('',#100484,#77937,#77938) ;
#68079=AXIS2_PLACEMENT_3D('',#100485,#77939,#77940) ;
#68080=AXIS2_PLACEMENT_3D('',#100486,#77941,#77942) ;
#68081=AXIS2_PLACEMENT_3D('',#100487,#77943,#77944) ;
#68082=AXIS2_PLACEMENT_3D('',#100488,#77945,#77946) ;
#68083=AXIS2_PLACEMENT_3D('',#100489,#77947,#77948) ;
#68084=AXIS2_PLACEMENT_3D('',#100490,#77949,#77950) ;
#68085=AXIS2_PLACEMENT_3D('',#100491,#77951,#77952) ;
#68086=AXIS2_PLACEMENT_3D('',#100492,#77953,#77954) ;
#68087=AXIS2_PLACEMENT_3D('',#100493,#77955,#77956) ;
#68088=AXIS2_PLACEMENT_3D('',#100494,#77957,#77958) ;
#68089=AXIS2_PLACEMENT_3D('',#100495,#77959,#77960) ;
#68090=AXIS2_PLACEMENT_3D('',#100496,#77961,#77962) ;
#68091=AXIS2_PLACEMENT_3D('',#100497,#77963,#77964) ;
#68092=AXIS2_PLACEMENT_3D('',#100498,#77965,#77966) ;
#68093=AXIS2_PLACEMENT_3D('',#100499,#77967,#77968) ;
#68094=AXIS2_PLACEMENT_3D('',#100500,#77969,#77970) ;
#68095=AXIS2_PLACEMENT_3D('',#100501,#77971,#77972) ;
#68096=AXIS2_PLACEMENT_3D('',#100502,#77973,#77974) ;
#68097=AXIS2_PLACEMENT_3D('',#100503,#77975,#77976) ;
#68098=AXIS2_PLACEMENT_3D('',#100504,#77977,#77978) ;
#68099=AXIS2_PLACEMENT_3D('',#100505,#77979,#77980) ;
#68100=AXIS2_PLACEMENT_3D('',#100506,#77981,#77982) ;
#68101=AXIS2_PLACEMENT_3D('',#100507,#77983,#77984) ;
#68102=AXIS2_PLACEMENT_3D('',#100508,#77985,#77986) ;
#68103=AXIS2_PLACEMENT_3D('',#100509,#77987,#77988) ;
#68104=AXIS2_PLACEMENT_3D('',#100510,#77989,#77990) ;
#68105=AXIS2_PLACEMENT_3D('',#100511,#77991,#77992) ;
#68106=AXIS2_PLACEMENT_3D('',#100512,#77993,#77994) ;
#68107=AXIS2_PLACEMENT_3D('',#100513,#77995,#77996) ;
#68108=AXIS2_PLACEMENT_3D('',#100514,#77997,#77998) ;
#68109=AXIS2_PLACEMENT_3D('',#100515,#77999,#78000) ;
#68110=AXIS2_PLACEMENT_3D('',#100516,#78001,#78002) ;
#68111=AXIS2_PLACEMENT_3D('',#100517,#78003,#78004) ;
#68112=AXIS2_PLACEMENT_3D('',#100518,#78005,#78006) ;
#68113=AXIS2_PLACEMENT_3D('',#100519,#78007,#78008) ;
#68114=AXIS2_PLACEMENT_3D('',#100520,#78009,#78010) ;
#68115=AXIS2_PLACEMENT_3D('',#100521,#78011,#78012) ;
#68116=AXIS2_PLACEMENT_3D('',#100522,#78013,#78014) ;
#68117=AXIS2_PLACEMENT_3D('',#100523,#78015,#78016) ;
#68118=AXIS2_PLACEMENT_3D('',#100524,#78017,#78018) ;
#68119=AXIS2_PLACEMENT_3D('',#100525,#78019,#78020) ;
#68120=AXIS2_PLACEMENT_3D('',#100526,#78021,#78022) ;
#68121=AXIS2_PLACEMENT_3D('',#100527,#78023,#78024) ;
#68122=AXIS2_PLACEMENT_3D('',#100528,#78025,#78026) ;
#68123=AXIS2_PLACEMENT_3D('',#100529,#78027,#78028) ;
#68124=AXIS2_PLACEMENT_3D('',#100530,#78029,#78030) ;
#68125=AXIS2_PLACEMENT_3D('',#100531,#78031,#78032) ;
#68126=AXIS2_PLACEMENT_3D('',#100532,#78033,#78034) ;
#68127=AXIS2_PLACEMENT_3D('',#100533,#78035,#78036) ;
#68128=AXIS2_PLACEMENT_3D('',#100534,#78037,#78038) ;
#68129=AXIS2_PLACEMENT_3D('',#100535,#78039,#78040) ;
#68130=AXIS2_PLACEMENT_3D('',#100536,#78041,#78042) ;
#68131=AXIS2_PLACEMENT_3D('',#100537,#78043,#78044) ;
#68132=AXIS2_PLACEMENT_3D('',#100538,#78045,#78046) ;
#68133=AXIS2_PLACEMENT_3D('',#100539,#78047,#78048) ;
#68134=AXIS2_PLACEMENT_3D('',#100540,#78049,#78050) ;
#68135=AXIS2_PLACEMENT_3D('',#100541,#78051,#78052) ;
#68136=AXIS2_PLACEMENT_3D('',#100542,#78053,#78054) ;
#68137=AXIS2_PLACEMENT_3D('',#100543,#78055,#78056) ;
#68138=AXIS2_PLACEMENT_3D('',#100544,#78057,#78058) ;
#68139=AXIS2_PLACEMENT_3D('',#100545,#78059,#78060) ;
#68140=AXIS2_PLACEMENT_3D('',#100546,#78061,#78062) ;
#68141=AXIS2_PLACEMENT_3D('',#100547,#78063,#78064) ;
#68142=AXIS2_PLACEMENT_3D('',#100548,#78065,#78066) ;
#68143=AXIS2_PLACEMENT_3D('',#100549,#78067,#78068) ;
#68144=AXIS2_PLACEMENT_3D('',#100550,#78069,#78070) ;
#68145=AXIS2_PLACEMENT_3D('',#100551,#78071,#78072) ;
#68146=AXIS2_PLACEMENT_3D('',#100552,#78073,#78074) ;
#68147=AXIS2_PLACEMENT_3D('',#100553,#78075,#78076) ;
#68148=AXIS2_PLACEMENT_3D('',#100554,#78077,#78078) ;
#68149=AXIS2_PLACEMENT_3D('',#100555,#78079,#78080) ;
#68150=AXIS2_PLACEMENT_3D('',#100556,#78081,#78082) ;
#68151=AXIS2_PLACEMENT_3D('',#100557,#78083,#78084) ;
#68152=AXIS2_PLACEMENT_3D('',#100558,#78085,#78086) ;
#68153=AXIS2_PLACEMENT_3D('',#100559,#78087,#78088) ;
#68154=AXIS2_PLACEMENT_3D('',#100560,#78089,#78090) ;
#68155=AXIS2_PLACEMENT_3D('',#100561,#78091,#78092) ;
#68156=AXIS2_PLACEMENT_3D('',#100562,#78093,#78094) ;
#68157=AXIS2_PLACEMENT_3D('',#100563,#78095,#78096) ;
#68158=AXIS2_PLACEMENT_3D('',#100564,#78097,#78098) ;
#68159=AXIS2_PLACEMENT_3D('',#100565,#78099,#78100) ;
#68160=AXIS2_PLACEMENT_3D('',#100566,#78101,#78102) ;
#68161=AXIS2_PLACEMENT_3D('',#100567,#78103,#78104) ;
#68162=AXIS2_PLACEMENT_3D('',#100568,#78105,#78106) ;
#68163=AXIS2_PLACEMENT_3D('',#100569,#78107,#78108) ;
#68164=AXIS2_PLACEMENT_3D('',#100570,#78109,#78110) ;
#68165=AXIS2_PLACEMENT_3D('',#100571,#78111,#78112) ;
#68166=AXIS2_PLACEMENT_3D('',#100572,#78113,#78114) ;
#68167=AXIS2_PLACEMENT_3D('',#100573,#78115,#78116) ;
#68168=AXIS2_PLACEMENT_3D('',#100574,#78117,#78118) ;
#68169=AXIS2_PLACEMENT_3D('',#100575,#78119,#78120) ;
#68170=AXIS2_PLACEMENT_3D('',#100576,#78121,#78122) ;
#68171=AXIS2_PLACEMENT_3D('',#100577,#78123,#78124) ;
#68172=AXIS2_PLACEMENT_3D('',#100578,#78125,#78126) ;
#68173=AXIS2_PLACEMENT_3D('',#100579,#78127,#78128) ;
#68174=AXIS2_PLACEMENT_3D('',#100580,#78129,#78130) ;
#68175=AXIS2_PLACEMENT_3D('',#100581,#78131,#78132) ;
#68176=AXIS2_PLACEMENT_3D('',#100582,#78133,#78134) ;
#68177=AXIS2_PLACEMENT_3D('',#100583,#78135,#78136) ;
#68178=AXIS2_PLACEMENT_3D('',#100584,#78137,#78138) ;
#68179=AXIS2_PLACEMENT_3D('',#100585,#78139,#78140) ;
#68180=AXIS2_PLACEMENT_3D('',#100586,#78141,#78142) ;
#68181=AXIS2_PLACEMENT_3D('',#100587,#78143,#78144) ;
#68182=AXIS2_PLACEMENT_3D('',#100588,#78145,#78146) ;
#68183=AXIS2_PLACEMENT_3D('',#100589,#78147,#78148) ;
#68184=AXIS2_PLACEMENT_3D('',#100590,#78149,#78150) ;
#68185=AXIS2_PLACEMENT_3D('',#100591,#78151,#78152) ;
#68186=AXIS2_PLACEMENT_3D('',#100592,#78153,#78154) ;
#68187=AXIS2_PLACEMENT_3D('',#100593,#78155,#78156) ;
#68188=AXIS2_PLACEMENT_3D('',#100594,#78157,#78158) ;
#68189=AXIS2_PLACEMENT_3D('',#100595,#78159,#78160) ;
#68190=AXIS2_PLACEMENT_3D('',#100596,#78161,#78162) ;
#68191=AXIS2_PLACEMENT_3D('',#100597,#78163,#78164) ;
#68192=AXIS2_PLACEMENT_3D('',#100598,#78165,#78166) ;
#68193=AXIS2_PLACEMENT_3D('',#100599,#78167,#78168) ;
#68194=AXIS2_PLACEMENT_3D('',#100600,#78169,#78170) ;
#68195=AXIS2_PLACEMENT_3D('',#100601,#78171,#78172) ;
#68196=AXIS2_PLACEMENT_3D('',#100602,#78173,#78174) ;
#68197=AXIS2_PLACEMENT_3D('',#100603,#78175,#78176) ;
#68198=AXIS2_PLACEMENT_3D('',#100604,#78177,#78178) ;
#68199=AXIS2_PLACEMENT_3D('',#100605,#78179,#78180) ;
#68200=AXIS2_PLACEMENT_3D('',#100606,#78181,#78182) ;
#68201=AXIS2_PLACEMENT_3D('',#100607,#78183,#78184) ;
#68202=AXIS2_PLACEMENT_3D('',#100608,#78185,#78186) ;
#68203=AXIS2_PLACEMENT_3D('',#100609,#78187,#78188) ;
#68204=AXIS2_PLACEMENT_3D('',#100610,#78189,#78190) ;
#68205=AXIS2_PLACEMENT_3D('',#100611,#78191,#78192) ;
#68206=AXIS2_PLACEMENT_3D('',#100612,#78193,#78194) ;
#68207=AXIS2_PLACEMENT_3D('',#100613,#78195,#78196) ;
#68208=AXIS2_PLACEMENT_3D('',#100614,#78197,#78198) ;
#68209=AXIS2_PLACEMENT_3D('',#100615,#78199,#78200) ;
#68210=AXIS2_PLACEMENT_3D('',#100616,#78201,#78202) ;
#68211=AXIS2_PLACEMENT_3D('',#100617,#78203,#78204) ;
#68212=AXIS2_PLACEMENT_3D('',#100618,#78205,#78206) ;
#68213=AXIS2_PLACEMENT_3D('',#100619,#78207,#78208) ;
#68214=AXIS2_PLACEMENT_3D('',#100620,#78209,#78210) ;
#68215=AXIS2_PLACEMENT_3D('',#100621,#78211,#78212) ;
#68216=AXIS2_PLACEMENT_3D('',#100622,#78213,#78214) ;
#68217=AXIS2_PLACEMENT_3D('',#100623,#78215,#78216) ;
#68218=AXIS2_PLACEMENT_3D('',#100624,#78217,#78218) ;
#68219=AXIS2_PLACEMENT_3D('',#100625,#78219,#78220) ;
#68220=AXIS2_PLACEMENT_3D('',#100626,#78221,#78222) ;
#68221=AXIS2_PLACEMENT_3D('',#100627,#78223,#78224) ;
#68222=AXIS2_PLACEMENT_3D('',#100628,#78225,#78226) ;
#68223=AXIS2_PLACEMENT_3D('',#100629,#78227,#78228) ;
#68224=AXIS2_PLACEMENT_3D('',#100630,#78229,#78230) ;
#68225=AXIS2_PLACEMENT_3D('',#100631,#78231,#78232) ;
#68226=AXIS2_PLACEMENT_3D('',#100632,#78233,#78234) ;
#68227=AXIS2_PLACEMENT_3D('',#100633,#78235,#78236) ;
#68228=AXIS2_PLACEMENT_3D('',#100634,#78237,#78238) ;
#68229=AXIS2_PLACEMENT_3D('',#100635,#78239,#78240) ;
#68230=AXIS2_PLACEMENT_3D('',#100636,#78241,#78242) ;
#68231=AXIS2_PLACEMENT_3D('',#100637,#78243,#78244) ;
#68232=AXIS2_PLACEMENT_3D('',#100638,#78245,#78246) ;
#68233=AXIS2_PLACEMENT_3D('',#100639,#78247,#78248) ;
#68234=AXIS2_PLACEMENT_3D('',#100640,#78249,#78250) ;
#68235=AXIS2_PLACEMENT_3D('',#100641,#78251,#78252) ;
#68236=AXIS2_PLACEMENT_3D('',#100642,#78253,#78254) ;
#68237=AXIS2_PLACEMENT_3D('',#100643,#78255,#78256) ;
#68238=AXIS2_PLACEMENT_3D('',#100644,#78257,#78258) ;
#68239=AXIS2_PLACEMENT_3D('',#100645,#78259,#78260) ;
#68240=AXIS2_PLACEMENT_3D('',#100646,#78261,#78262) ;
#68241=AXIS2_PLACEMENT_3D('',#100647,#78263,#78264) ;
#68242=AXIS2_PLACEMENT_3D('',#100648,#78265,#78266) ;
#68243=AXIS2_PLACEMENT_3D('',#100649,#78267,#78268) ;
#68244=AXIS2_PLACEMENT_3D('',#100650,#78269,#78270) ;
#68245=AXIS2_PLACEMENT_3D('',#100651,#78271,#78272) ;
#68246=AXIS2_PLACEMENT_3D('',#100652,#78273,#78274) ;
#68247=AXIS2_PLACEMENT_3D('',#100653,#78275,#78276) ;
#68248=AXIS2_PLACEMENT_3D('',#100654,#78277,#78278) ;
#68249=AXIS2_PLACEMENT_3D('',#100655,#78279,#78280) ;
#68250=AXIS2_PLACEMENT_3D('',#100656,#78281,#78282) ;
#68251=AXIS2_PLACEMENT_3D('',#100657,#78283,#78284) ;
#68252=AXIS2_PLACEMENT_3D('',#100658,#78285,#78286) ;
#68253=AXIS2_PLACEMENT_3D('',#100659,#78287,#78288) ;
#68254=AXIS2_PLACEMENT_3D('',#100660,#78289,#78290) ;
#68255=AXIS2_PLACEMENT_3D('',#100661,#78291,#78292) ;
#68256=AXIS2_PLACEMENT_3D('',#100662,#78293,#78294) ;
#68257=AXIS2_PLACEMENT_3D('',#100663,#78295,#78296) ;
#68258=AXIS2_PLACEMENT_3D('',#100664,#78297,#78298) ;
#68259=AXIS2_PLACEMENT_3D('',#100665,#78299,#78300) ;
#68260=AXIS2_PLACEMENT_3D('',#100666,#78301,#78302) ;
#68261=AXIS2_PLACEMENT_3D('',#100667,#78303,#78304) ;
#68262=AXIS2_PLACEMENT_3D('',#100668,#78305,#78306) ;
#68263=AXIS2_PLACEMENT_3D('',#100669,#78307,#78308) ;
#68264=AXIS2_PLACEMENT_3D('',#100670,#78309,#78310) ;
#68265=AXIS2_PLACEMENT_3D('',#100671,#78311,#78312) ;
#68266=AXIS2_PLACEMENT_3D('',#100672,#78313,#78314) ;
#68267=AXIS2_PLACEMENT_3D('',#100673,#78315,#78316) ;
#68268=AXIS2_PLACEMENT_3D('',#100674,#78317,#78318) ;
#68269=AXIS2_PLACEMENT_3D('',#100675,#78319,#78320) ;
#68270=AXIS2_PLACEMENT_3D('',#100676,#78321,#78322) ;
#68271=AXIS2_PLACEMENT_3D('',#100677,#78323,#78324) ;
#68272=AXIS2_PLACEMENT_3D('',#100678,#78325,#78326) ;
#68273=AXIS2_PLACEMENT_3D('',#100679,#78327,#78328) ;
#68274=AXIS2_PLACEMENT_3D('',#100680,#78329,#78330) ;
#68275=AXIS2_PLACEMENT_3D('',#100681,#78331,#78332) ;
#68276=AXIS2_PLACEMENT_3D('',#100682,#78333,#78334) ;
#68277=AXIS2_PLACEMENT_3D('',#100683,#78335,#78336) ;
#68278=AXIS2_PLACEMENT_3D('',#100684,#78337,#78338) ;
#68279=AXIS2_PLACEMENT_3D('',#100685,#78339,#78340) ;
#68280=AXIS2_PLACEMENT_3D('',#100686,#78341,#78342) ;
#68281=AXIS2_PLACEMENT_3D('',#100687,#78343,#78344) ;
#68282=AXIS2_PLACEMENT_3D('',#100688,#78345,#78346) ;
#68283=AXIS2_PLACEMENT_3D('',#100689,#78347,#78348) ;
#68284=AXIS2_PLACEMENT_3D('',#100690,#78349,#78350) ;
#68285=AXIS2_PLACEMENT_3D('',#100691,#78351,#78352) ;
#68286=AXIS2_PLACEMENT_3D('',#100692,#78353,#78354) ;
#68287=AXIS2_PLACEMENT_3D('',#100693,#78355,#78356) ;
#68288=AXIS2_PLACEMENT_3D('',#100694,#78357,#78358) ;
#68289=AXIS2_PLACEMENT_3D('',#100695,#78359,#78360) ;
#68290=AXIS2_PLACEMENT_3D('',#100696,#78361,#78362) ;
#68291=AXIS2_PLACEMENT_3D('',#100697,#78363,#78364) ;
#68292=AXIS2_PLACEMENT_3D('',#100698,#78365,#78366) ;
#68293=AXIS2_PLACEMENT_3D('',#100699,#78367,#78368) ;
#68294=AXIS2_PLACEMENT_3D('',#100700,#78369,#78370) ;
#68295=AXIS2_PLACEMENT_3D('',#100701,#78371,#78372) ;
#68296=AXIS2_PLACEMENT_3D('',#100702,#78373,#78374) ;
#68297=AXIS2_PLACEMENT_3D('',#100703,#78375,#78376) ;
#68298=AXIS2_PLACEMENT_3D('',#100704,#78377,#78378) ;
#68299=AXIS2_PLACEMENT_3D('',#100705,#78379,#78380) ;
#68300=AXIS2_PLACEMENT_3D('',#100706,#78381,#78382) ;
#68301=AXIS2_PLACEMENT_3D('',#100707,#78383,#78384) ;
#68302=AXIS2_PLACEMENT_3D('',#100708,#78385,#78386) ;
#68303=AXIS2_PLACEMENT_3D('',#100709,#78387,#78388) ;
#68304=AXIS2_PLACEMENT_3D('',#100710,#78389,#78390) ;
#68305=AXIS2_PLACEMENT_3D('',#100711,#78391,#78392) ;
#68306=AXIS2_PLACEMENT_3D('',#100712,#78393,#78394) ;
#68307=AXIS2_PLACEMENT_3D('',#100713,#78395,#78396) ;
#68308=AXIS2_PLACEMENT_3D('',#100714,#78397,#78398) ;
#68309=AXIS2_PLACEMENT_3D('',#100715,#78399,#78400) ;
#68310=AXIS2_PLACEMENT_3D('',#100716,#78401,#78402) ;
#68311=AXIS2_PLACEMENT_3D('',#100717,#78403,#78404) ;
#68312=AXIS2_PLACEMENT_3D('',#100718,#78405,#78406) ;
#68313=AXIS2_PLACEMENT_3D('',#100719,#78407,#78408) ;
#68314=AXIS2_PLACEMENT_3D('',#100720,#78409,#78410) ;
#68315=AXIS2_PLACEMENT_3D('',#100721,#78411,#78412) ;
#68316=AXIS2_PLACEMENT_3D('',#100722,#78413,#78414) ;
#68317=AXIS2_PLACEMENT_3D('',#100723,#78415,#78416) ;
#68318=AXIS2_PLACEMENT_3D('',#100724,#78417,#78418) ;
#68319=AXIS2_PLACEMENT_3D('',#100725,#78419,#78420) ;
#68320=AXIS2_PLACEMENT_3D('',#100726,#78421,#78422) ;
#68321=AXIS2_PLACEMENT_3D('',#100727,#78423,#78424) ;
#68322=AXIS2_PLACEMENT_3D('',#100728,#78425,#78426) ;
#68323=AXIS2_PLACEMENT_3D('',#100729,#78427,#78428) ;
#68324=AXIS2_PLACEMENT_3D('',#100730,#78429,#78430) ;
#68325=AXIS2_PLACEMENT_3D('',#100731,#78431,#78432) ;
#68326=AXIS2_PLACEMENT_3D('',#100732,#78433,#78434) ;
#68327=AXIS2_PLACEMENT_3D('',#100733,#78435,#78436) ;
#68328=AXIS2_PLACEMENT_3D('',#100734,#78437,#78438) ;
#68329=AXIS2_PLACEMENT_3D('',#100735,#78439,#78440) ;
#68330=AXIS2_PLACEMENT_3D('',#100736,#78441,#78442) ;
#68331=AXIS2_PLACEMENT_3D('',#100737,#78443,#78444) ;
#68332=AXIS2_PLACEMENT_3D('',#100738,#78445,#78446) ;
#68333=AXIS2_PLACEMENT_3D('',#100739,#78447,#78448) ;
#68334=AXIS2_PLACEMENT_3D('',#100740,#78449,#78450) ;
#68335=AXIS2_PLACEMENT_3D('',#100741,#78451,#78452) ;
#68336=AXIS2_PLACEMENT_3D('',#100742,#78453,#78454) ;
#68337=AXIS2_PLACEMENT_3D('',#100743,#78455,#78456) ;
#68338=AXIS2_PLACEMENT_3D('',#100744,#78457,#78458) ;
#68339=AXIS2_PLACEMENT_3D('',#100745,#78459,#78460) ;
#68340=AXIS2_PLACEMENT_3D('',#100746,#78461,#78462) ;
#68341=AXIS2_PLACEMENT_3D('',#100747,#78463,#78464) ;
#68342=AXIS2_PLACEMENT_3D('',#100748,#78465,#78466) ;
#68343=AXIS2_PLACEMENT_3D('',#100749,#78467,#78468) ;
#68344=AXIS2_PLACEMENT_3D('',#100750,#78469,#78470) ;
#68345=AXIS2_PLACEMENT_3D('',#100751,#78471,#78472) ;
#68346=AXIS2_PLACEMENT_3D('',#100752,#78473,#78474) ;
#68347=AXIS2_PLACEMENT_3D('',#100753,#78475,#78476) ;
#68348=AXIS2_PLACEMENT_3D('',#100754,#78477,#78478) ;
#68349=AXIS2_PLACEMENT_3D('',#100755,#78479,#78480) ;
#68350=AXIS2_PLACEMENT_3D('',#100756,#78481,#78482) ;
#68351=AXIS2_PLACEMENT_3D('',#100757,#78483,#78484) ;
#68352=AXIS2_PLACEMENT_3D('',#100758,#78485,#78486) ;
#68353=AXIS2_PLACEMENT_3D('',#100759,#78487,#78488) ;
#68354=AXIS2_PLACEMENT_3D('',#100760,#78489,#78490) ;
#68355=AXIS2_PLACEMENT_3D('',#100761,#78491,#78492) ;
#68356=AXIS2_PLACEMENT_3D('',#100762,#78493,#78494) ;
#68357=AXIS2_PLACEMENT_3D('',#100763,#78495,#78496) ;
#68358=AXIS2_PLACEMENT_3D('',#100764,#78497,#78498) ;
#68359=AXIS2_PLACEMENT_3D('',#100765,#78499,#78500) ;
#68360=AXIS2_PLACEMENT_3D('',#100766,#78501,#78502) ;
#68361=AXIS2_PLACEMENT_3D('',#100767,#78503,#78504) ;
#68362=AXIS2_PLACEMENT_3D('',#100768,#78505,#78506) ;
#68363=AXIS2_PLACEMENT_3D('',#100769,#78507,#78508) ;
#68364=AXIS2_PLACEMENT_3D('',#100770,#78509,#78510) ;
#68365=AXIS2_PLACEMENT_3D('',#100771,#78511,#78512) ;
#68366=AXIS2_PLACEMENT_3D('',#100772,#78513,#78514) ;
#68367=AXIS2_PLACEMENT_3D('',#100773,#78515,#78516) ;
#68368=AXIS2_PLACEMENT_3D('',#100774,#78517,#78518) ;
#68369=AXIS2_PLACEMENT_3D('',#100775,#78519,#78520) ;
#68370=AXIS2_PLACEMENT_3D('',#100776,#78521,#78522) ;
#68371=AXIS2_PLACEMENT_3D('',#100777,#78523,#78524) ;
#68372=AXIS2_PLACEMENT_3D('',#100778,#78525,#78526) ;
#68373=AXIS2_PLACEMENT_3D('',#100779,#78527,#78528) ;
#68374=AXIS2_PLACEMENT_3D('',#100780,#78529,#78530) ;
#68375=AXIS2_PLACEMENT_3D('',#100781,#78531,#78532) ;
#68376=AXIS2_PLACEMENT_3D('',#100782,#78533,#78534) ;
#68377=AXIS2_PLACEMENT_3D('',#100783,#78535,#78536) ;
#68378=AXIS2_PLACEMENT_3D('',#100784,#78537,#78538) ;
#68379=AXIS2_PLACEMENT_3D('',#100785,#78539,#78540) ;
#68380=AXIS2_PLACEMENT_3D('',#100786,#78541,#78542) ;
#68381=AXIS2_PLACEMENT_3D('',#100787,#78543,#78544) ;
#68382=AXIS2_PLACEMENT_3D('',#100788,#78545,#78546) ;
#68383=AXIS2_PLACEMENT_3D('',#100789,#78547,#78548) ;
#68384=AXIS2_PLACEMENT_3D('',#100790,#78549,#78550) ;
#68385=AXIS2_PLACEMENT_3D('',#100791,#78551,#78552) ;
#68386=AXIS2_PLACEMENT_3D('',#100792,#78553,#78554) ;
#68387=AXIS2_PLACEMENT_3D('',#100793,#78555,#78556) ;
#68388=AXIS2_PLACEMENT_3D('',#100794,#78557,#78558) ;
#68389=AXIS2_PLACEMENT_3D('',#100795,#78559,#78560) ;
#68390=AXIS2_PLACEMENT_3D('',#100796,#78561,#78562) ;
#68391=AXIS2_PLACEMENT_3D('',#100797,#78563,#78564) ;
#68392=AXIS2_PLACEMENT_3D('',#100798,#78565,#78566) ;
#68393=AXIS2_PLACEMENT_3D('',#100799,#78567,#78568) ;
#68394=AXIS2_PLACEMENT_3D('',#100800,#78569,#78570) ;
#68395=AXIS2_PLACEMENT_3D('',#100801,#78571,#78572) ;
#68396=AXIS2_PLACEMENT_3D('',#100802,#78573,#78574) ;
#68397=AXIS2_PLACEMENT_3D('',#100803,#78575,#78576) ;
#68398=AXIS2_PLACEMENT_3D('',#100804,#78577,#78578) ;
#68399=AXIS2_PLACEMENT_3D('',#100805,#78579,#78580) ;
#68400=AXIS2_PLACEMENT_3D('',#100806,#78581,#78582) ;
#68401=AXIS2_PLACEMENT_3D('',#100807,#78583,#78584) ;
#68402=AXIS2_PLACEMENT_3D('',#100808,#78585,#78586) ;
#68403=AXIS2_PLACEMENT_3D('',#100809,#78587,#78588) ;
#68404=AXIS2_PLACEMENT_3D('',#100810,#78589,#78590) ;
#68405=AXIS2_PLACEMENT_3D('',#100811,#78591,#78592) ;
#68406=AXIS2_PLACEMENT_3D('',#100812,#78593,#78594) ;
#68407=AXIS2_PLACEMENT_3D('',#100813,#78595,#78596) ;
#68408=AXIS2_PLACEMENT_3D('',#100814,#78597,#78598) ;
#68409=AXIS2_PLACEMENT_3D('',#100815,#78599,#78600) ;
#68410=AXIS2_PLACEMENT_3D('',#100816,#78601,#78602) ;
#68411=AXIS2_PLACEMENT_3D('',#100817,#78603,#78604) ;
#68412=AXIS2_PLACEMENT_3D('',#100818,#78605,#78606) ;
#68413=AXIS2_PLACEMENT_3D('',#100819,#78607,#78608) ;
#68414=AXIS2_PLACEMENT_3D('',#100820,#78609,#78610) ;
#68415=AXIS2_PLACEMENT_3D('',#100821,#78611,#78612) ;
#68416=AXIS2_PLACEMENT_3D('',#100822,#78613,#78614) ;
#68417=AXIS2_PLACEMENT_3D('',#100823,#78615,#78616) ;
#68418=AXIS2_PLACEMENT_3D('',#100824,#78617,#78618) ;
#68419=AXIS2_PLACEMENT_3D('',#100825,#78619,#78620) ;
#68420=AXIS2_PLACEMENT_3D('',#100826,#78621,#78622) ;
#68421=AXIS2_PLACEMENT_3D('',#100827,#78623,#78624) ;
#68422=AXIS2_PLACEMENT_3D('',#100828,#78625,#78626) ;
#68423=AXIS2_PLACEMENT_3D('',#100829,#78627,#78628) ;
#68424=AXIS2_PLACEMENT_3D('',#100830,#78629,#78630) ;
#68425=AXIS2_PLACEMENT_3D('',#100831,#78631,#78632) ;
#68426=AXIS2_PLACEMENT_3D('',#100832,#78633,#78634) ;
#68427=AXIS2_PLACEMENT_3D('',#100833,#78635,#78636) ;
#68428=AXIS2_PLACEMENT_3D('',#100834,#78637,#78638) ;
#68429=AXIS2_PLACEMENT_3D('',#100835,#78639,#78640) ;
#68430=AXIS2_PLACEMENT_3D('',#100836,#78641,#78642) ;
#68431=AXIS2_PLACEMENT_3D('',#100837,#78643,#78644) ;
#68432=AXIS2_PLACEMENT_3D('',#100838,#78645,#78646) ;
#68433=AXIS2_PLACEMENT_3D('',#100839,#78647,#78648) ;
#68434=AXIS2_PLACEMENT_3D('',#100840,#78649,#78650) ;
#68435=AXIS2_PLACEMENT_3D('',#100841,#78651,#78652) ;
#68436=AXIS2_PLACEMENT_3D('',#100842,#78653,#78654) ;
#68437=AXIS2_PLACEMENT_3D('',#100843,#78655,#78656) ;
#68438=AXIS2_PLACEMENT_3D('',#100844,#78657,#78658) ;
#68439=AXIS2_PLACEMENT_3D('',#100845,#78659,#78660) ;
#68440=AXIS2_PLACEMENT_3D('',#100846,#78661,#78662) ;
#68441=AXIS2_PLACEMENT_3D('',#100847,#78663,#78664) ;
#68442=AXIS2_PLACEMENT_3D('',#100848,#78665,#78666) ;
#68443=AXIS2_PLACEMENT_3D('',#100849,#78667,#78668) ;
#68444=AXIS2_PLACEMENT_3D('',#100850,#78669,#78670) ;
#68445=AXIS2_PLACEMENT_3D('',#100851,#78671,#78672) ;
#68446=AXIS2_PLACEMENT_3D('',#100852,#78673,#78674) ;
#68447=AXIS2_PLACEMENT_3D('',#100853,#78675,#78676) ;
#68448=AXIS2_PLACEMENT_3D('',#100854,#78677,#78678) ;
#68449=AXIS2_PLACEMENT_3D('',#100855,#78679,#78680) ;
#68450=AXIS2_PLACEMENT_3D('',#100856,#78681,#78682) ;
#68451=AXIS2_PLACEMENT_3D('',#100857,#78683,#78684) ;
#68452=AXIS2_PLACEMENT_3D('',#100858,#78685,#78686) ;
#68453=AXIS2_PLACEMENT_3D('',#100859,#78687,#78688) ;
#68454=AXIS2_PLACEMENT_3D('',#100860,#78689,#78690) ;
#68455=AXIS2_PLACEMENT_3D('',#100861,#78691,#78692) ;
#68456=AXIS2_PLACEMENT_3D('',#100862,#78693,#78694) ;
#68457=AXIS2_PLACEMENT_3D('',#100863,#78695,#78696) ;
#68458=AXIS2_PLACEMENT_3D('',#100864,#78697,#78698) ;
#68459=AXIS2_PLACEMENT_3D('',#100865,#78699,#78700) ;
#68460=AXIS2_PLACEMENT_3D('',#100866,#78701,#78702) ;
#68461=AXIS2_PLACEMENT_3D('',#100867,#78703,#78704) ;
#68462=AXIS2_PLACEMENT_3D('',#100868,#78705,#78706) ;
#68463=AXIS2_PLACEMENT_3D('',#100869,#78707,#78708) ;
#68464=AXIS2_PLACEMENT_3D('',#100870,#78709,#78710) ;
#68465=AXIS2_PLACEMENT_3D('',#100871,#78711,#78712) ;
#68466=AXIS2_PLACEMENT_3D('',#100872,#78713,#78714) ;
#68467=AXIS2_PLACEMENT_3D('',#100873,#78715,#78716) ;
#68468=AXIS2_PLACEMENT_3D('',#100874,#78717,#78718) ;
#68469=AXIS2_PLACEMENT_3D('',#100875,#78719,#78720) ;
#68470=AXIS2_PLACEMENT_3D('',#100876,#78721,#78722) ;
#68471=AXIS2_PLACEMENT_3D('',#100877,#78723,#78724) ;
#68472=AXIS2_PLACEMENT_3D('',#100878,#78725,#78726) ;
#68473=AXIS2_PLACEMENT_3D('',#100879,#78727,#78728) ;
#68474=AXIS2_PLACEMENT_3D('',#100880,#78729,#78730) ;
#68475=AXIS2_PLACEMENT_3D('',#100881,#78731,#78732) ;
#68476=AXIS2_PLACEMENT_3D('',#100882,#78733,#78734) ;
#68477=AXIS2_PLACEMENT_3D('',#100883,#78735,#78736) ;
#68478=AXIS2_PLACEMENT_3D('',#100884,#78737,#78738) ;
#68479=AXIS2_PLACEMENT_3D('',#100885,#78739,#78740) ;
#68480=AXIS2_PLACEMENT_3D('',#100886,#78741,#78742) ;
#68481=AXIS2_PLACEMENT_3D('',#100887,#78743,#78744) ;
#68482=AXIS2_PLACEMENT_3D('',#100888,#78745,#78746) ;
#68483=AXIS2_PLACEMENT_3D('',#100889,#78747,#78748) ;
#68484=AXIS2_PLACEMENT_3D('',#100890,#78749,#78750) ;
#68485=AXIS2_PLACEMENT_3D('',#100891,#78751,#78752) ;
#68486=AXIS2_PLACEMENT_3D('',#100892,#78753,#78754) ;
#68487=AXIS2_PLACEMENT_3D('',#100893,#78755,#78756) ;
#68488=AXIS2_PLACEMENT_3D('',#100894,#78757,#78758) ;
#68489=AXIS2_PLACEMENT_3D('',#100895,#78759,#78760) ;
#68490=AXIS2_PLACEMENT_3D('',#100896,#78761,#78762) ;
#68491=AXIS2_PLACEMENT_3D('',#100897,#78763,#78764) ;
#68492=AXIS2_PLACEMENT_3D('',#100898,#78765,#78766) ;
#68493=AXIS2_PLACEMENT_3D('',#100899,#78767,#78768) ;
#68494=AXIS2_PLACEMENT_3D('',#100900,#78769,#78770) ;
#68495=AXIS2_PLACEMENT_3D('',#100901,#78771,#78772) ;
#68496=AXIS2_PLACEMENT_3D('',#100902,#78773,#78774) ;
#68497=AXIS2_PLACEMENT_3D('',#100903,#78775,#78776) ;
#68498=AXIS2_PLACEMENT_3D('',#100904,#78777,#78778) ;
#68499=AXIS2_PLACEMENT_3D('',#100905,#78779,#78780) ;
#68500=AXIS2_PLACEMENT_3D('',#100906,#78781,#78782) ;
#68501=AXIS2_PLACEMENT_3D('',#100907,#78783,#78784) ;
#68502=AXIS2_PLACEMENT_3D('',#100908,#78785,#78786) ;
#68503=AXIS2_PLACEMENT_3D('',#100909,#78787,#78788) ;
#68504=AXIS2_PLACEMENT_3D('',#100910,#78789,#78790) ;
#68505=AXIS2_PLACEMENT_3D('',#100911,#78791,#78792) ;
#68506=AXIS2_PLACEMENT_3D('',#100912,#78793,#78794) ;
#68507=AXIS2_PLACEMENT_3D('',#100913,#78795,#78796) ;
#68508=AXIS2_PLACEMENT_3D('',#100914,#78797,#78798) ;
#68509=AXIS2_PLACEMENT_3D('',#100915,#78799,#78800) ;
#68510=AXIS2_PLACEMENT_3D('',#100916,#78801,#78802) ;
#68511=AXIS2_PLACEMENT_3D('',#100917,#78803,#78804) ;
#68512=AXIS2_PLACEMENT_3D('',#100918,#78805,#78806) ;
#68513=AXIS2_PLACEMENT_3D('',#100919,#78807,#78808) ;
#68514=AXIS2_PLACEMENT_3D('',#100920,#78809,#78810) ;
#68515=AXIS2_PLACEMENT_3D('',#100921,#78811,#78812) ;
#68516=AXIS2_PLACEMENT_3D('',#100922,#78813,#78814) ;
#68517=AXIS2_PLACEMENT_3D('',#100923,#78815,#78816) ;
#68518=AXIS2_PLACEMENT_3D('',#100924,#78817,#78818) ;
#68519=AXIS2_PLACEMENT_3D('',#100925,#78819,#78820) ;
#68520=AXIS2_PLACEMENT_3D('',#100926,#78821,#78822) ;
#68521=AXIS2_PLACEMENT_3D('',#100927,#78823,#78824) ;
#68522=AXIS2_PLACEMENT_3D('',#100928,#78825,#78826) ;
#68523=AXIS2_PLACEMENT_3D('',#100929,#78827,#78828) ;
#68524=AXIS2_PLACEMENT_3D('',#100930,#78829,#78830) ;
#68525=AXIS2_PLACEMENT_3D('',#100931,#78831,#78832) ;
#68526=AXIS2_PLACEMENT_3D('',#100932,#78833,#78834) ;
#68527=AXIS2_PLACEMENT_3D('',#100933,#78835,#78836) ;
#68528=AXIS2_PLACEMENT_3D('',#100934,#78837,#78838) ;
#68529=AXIS2_PLACEMENT_3D('',#100935,#78839,#78840) ;
#68530=AXIS2_PLACEMENT_3D('',#100936,#78841,#78842) ;
#68531=AXIS2_PLACEMENT_3D('',#100937,#78843,#78844) ;
#68532=AXIS2_PLACEMENT_3D('',#100938,#78845,#78846) ;
#68533=AXIS2_PLACEMENT_3D('',#100939,#78847,#78848) ;
#68534=AXIS2_PLACEMENT_3D('',#100940,#78849,#78850) ;
#68535=AXIS2_PLACEMENT_3D('',#100941,#78851,#78852) ;
#68536=AXIS2_PLACEMENT_3D('',#100942,#78853,#78854) ;
#68537=AXIS2_PLACEMENT_3D('',#100943,#78855,#78856) ;
#68538=AXIS2_PLACEMENT_3D('',#100944,#78857,#78858) ;
#68539=AXIS2_PLACEMENT_3D('',#100945,#78859,#78860) ;
#68540=AXIS2_PLACEMENT_3D('',#100946,#78861,#78862) ;
#68541=AXIS2_PLACEMENT_3D('',#100947,#78863,#78864) ;
#68542=AXIS2_PLACEMENT_3D('',#100948,#78865,#78866) ;
#68543=AXIS2_PLACEMENT_3D('',#100949,#78867,#78868) ;
#68544=AXIS2_PLACEMENT_3D('',#100950,#78869,#78870) ;
#68545=AXIS2_PLACEMENT_3D('',#100951,#78871,#78872) ;
#68546=AXIS2_PLACEMENT_3D('',#100952,#78873,#78874) ;
#68547=AXIS2_PLACEMENT_3D('',#100953,#78875,#78876) ;
#68548=AXIS2_PLACEMENT_3D('',#100954,#78877,#78878) ;
#68549=AXIS2_PLACEMENT_3D('',#100955,#78879,#78880) ;
#68550=AXIS2_PLACEMENT_3D('',#100956,#78881,#78882) ;
#68551=AXIS2_PLACEMENT_3D('',#100957,#78883,#78884) ;
#68552=AXIS2_PLACEMENT_3D('',#100958,#78885,#78886) ;
#68553=AXIS2_PLACEMENT_3D('',#100959,#78887,#78888) ;
#68554=AXIS2_PLACEMENT_3D('',#100960,#78889,#78890) ;
#68555=AXIS2_PLACEMENT_3D('',#100961,#78891,#78892) ;
#68556=AXIS2_PLACEMENT_3D('',#100962,#78893,#78894) ;
#68557=AXIS2_PLACEMENT_3D('',#100963,#78895,#78896) ;
#68558=AXIS2_PLACEMENT_3D('',#100964,#78897,#78898) ;
#68559=AXIS2_PLACEMENT_3D('',#100965,#78899,#78900) ;
#68560=AXIS2_PLACEMENT_3D('',#100966,#78901,#78902) ;
#68561=AXIS2_PLACEMENT_3D('',#100967,#78903,#78904) ;
#68562=AXIS2_PLACEMENT_3D('',#100968,#78905,#78906) ;
#68563=AXIS2_PLACEMENT_3D('',#100969,#78907,#78908) ;
#68564=AXIS2_PLACEMENT_3D('',#100970,#78909,#78910) ;
#68565=AXIS2_PLACEMENT_3D('',#100971,#78911,#78912) ;
#68566=AXIS2_PLACEMENT_3D('',#100972,#78913,#78914) ;
#68567=AXIS2_PLACEMENT_3D('',#100973,#78915,#78916) ;
#68568=AXIS2_PLACEMENT_3D('',#100974,#78917,#78918) ;
#68569=AXIS2_PLACEMENT_3D('',#100975,#78919,#78920) ;
#68570=AXIS2_PLACEMENT_3D('',#100976,#78921,#78922) ;
#68571=AXIS2_PLACEMENT_3D('',#100977,#78923,#78924) ;
#68572=AXIS2_PLACEMENT_3D('',#100978,#78925,#78926) ;
#68573=AXIS2_PLACEMENT_3D('',#100979,#78927,#78928) ;
#68574=AXIS2_PLACEMENT_3D('',#100980,#78929,#78930) ;
#68575=AXIS2_PLACEMENT_3D('',#100981,#78931,#78932) ;
#68576=AXIS2_PLACEMENT_3D('',#100982,#78933,#78934) ;
#68577=AXIS2_PLACEMENT_3D('',#100983,#78935,#78936) ;
#68578=AXIS2_PLACEMENT_3D('',#100984,#78937,#78938) ;
#68579=AXIS2_PLACEMENT_3D('',#100985,#78939,#78940) ;
#68580=AXIS2_PLACEMENT_3D('',#100986,#78941,#78942) ;
#68581=AXIS2_PLACEMENT_3D('',#100987,#78943,#78944) ;
#68582=AXIS2_PLACEMENT_3D('',#100988,#78945,#78946) ;
#68583=AXIS2_PLACEMENT_3D('',#100989,#78947,#78948) ;
#68584=AXIS2_PLACEMENT_3D('',#100990,#78949,#78950) ;
#68585=AXIS2_PLACEMENT_3D('',#100991,#78951,#78952) ;
#68586=AXIS2_PLACEMENT_3D('',#100992,#78953,#78954) ;
#68587=AXIS2_PLACEMENT_3D('',#100993,#78955,#78956) ;
#68588=AXIS2_PLACEMENT_3D('',#100994,#78957,#78958) ;
#68589=AXIS2_PLACEMENT_3D('',#100995,#78959,#78960) ;
#68590=AXIS2_PLACEMENT_3D('',#100996,#78961,#78962) ;
#68591=AXIS2_PLACEMENT_3D('',#100997,#78963,#78964) ;
#68592=AXIS2_PLACEMENT_3D('',#100998,#78965,#78966) ;
#68593=AXIS2_PLACEMENT_3D('',#100999,#78967,#78968) ;
#68594=AXIS2_PLACEMENT_3D('',#101000,#78969,#78970) ;
#68595=AXIS2_PLACEMENT_3D('',#101001,#78971,#78972) ;
#68596=AXIS2_PLACEMENT_3D('',#101002,#78973,#78974) ;
#68597=AXIS2_PLACEMENT_3D('',#101003,#78975,#78976) ;
#68598=AXIS2_PLACEMENT_3D('',#101004,#78977,#78978) ;
#68599=AXIS2_PLACEMENT_3D('',#101005,#78979,#78980) ;
#68600=AXIS2_PLACEMENT_3D('',#101006,#78981,#78982) ;
#68601=AXIS2_PLACEMENT_3D('',#101007,#78983,#78984) ;
#68602=AXIS2_PLACEMENT_3D('',#101008,#78985,#78986) ;
#68603=AXIS2_PLACEMENT_3D('',#101009,#78987,#78988) ;
#68604=AXIS2_PLACEMENT_3D('',#101010,#78989,#78990) ;
#68605=AXIS2_PLACEMENT_3D('',#101011,#78991,#78992) ;
#68606=AXIS2_PLACEMENT_3D('',#101012,#78993,#78994) ;
#68607=AXIS2_PLACEMENT_3D('',#101013,#78995,#78996) ;
#68608=AXIS2_PLACEMENT_3D('',#101014,#78997,#78998) ;
#68609=AXIS2_PLACEMENT_3D('',#101015,#78999,#79000) ;
#68610=AXIS2_PLACEMENT_3D('',#101016,#79001,#79002) ;
#68611=AXIS2_PLACEMENT_3D('',#101017,#79003,#79004) ;
#68612=AXIS2_PLACEMENT_3D('',#101018,#79005,#79006) ;
#68613=AXIS2_PLACEMENT_3D('',#101019,#79007,#79008) ;
#68614=AXIS2_PLACEMENT_3D('',#101020,#79009,#79010) ;
#68615=AXIS2_PLACEMENT_3D('',#101021,#79011,#79012) ;
#68616=AXIS2_PLACEMENT_3D('',#101022,#79013,#79014) ;
#68617=AXIS2_PLACEMENT_3D('',#101023,#79015,#79016) ;
#68618=AXIS2_PLACEMENT_3D('',#101024,#79017,#79018) ;
#68619=AXIS2_PLACEMENT_3D('',#101025,#79019,#79020) ;
#68620=AXIS2_PLACEMENT_3D('',#101026,#79021,#79022) ;
#68621=AXIS2_PLACEMENT_3D('',#101027,#79023,#79024) ;
#68622=AXIS2_PLACEMENT_3D('',#101028,#79025,#79026) ;
#68623=AXIS2_PLACEMENT_3D('',#101029,#79027,#79028) ;
#68624=AXIS2_PLACEMENT_3D('',#101030,#79029,#79030) ;
#68625=AXIS2_PLACEMENT_3D('',#101031,#79031,#79032) ;
#68626=AXIS2_PLACEMENT_3D('',#101032,#79033,#79034) ;
#68627=AXIS2_PLACEMENT_3D('',#101033,#79035,#79036) ;
#68628=AXIS2_PLACEMENT_3D('',#101034,#79037,#79038) ;
#68629=AXIS2_PLACEMENT_3D('',#101035,#79039,#79040) ;
#68630=AXIS2_PLACEMENT_3D('',#101036,#79041,#79042) ;
#68631=AXIS2_PLACEMENT_3D('',#101037,#79043,#79044) ;
#68632=AXIS2_PLACEMENT_3D('',#101038,#79045,#79046) ;
#68633=AXIS2_PLACEMENT_3D('',#101039,#79047,#79048) ;
#68634=AXIS2_PLACEMENT_3D('',#101040,#79049,#79050) ;
#68635=AXIS2_PLACEMENT_3D('',#101041,#79051,#79052) ;
#68636=AXIS2_PLACEMENT_3D('',#101042,#79053,#79054) ;
#68637=AXIS2_PLACEMENT_3D('',#101043,#79055,#79056) ;
#68638=AXIS2_PLACEMENT_3D('',#101044,#79057,#79058) ;
#68639=AXIS2_PLACEMENT_3D('',#101045,#79059,#79060) ;
#68640=AXIS2_PLACEMENT_3D('',#101046,#79061,#79062) ;
#68641=AXIS2_PLACEMENT_3D('',#101047,#79063,#79064) ;
#68642=AXIS2_PLACEMENT_3D('',#101048,#79065,#79066) ;
#68643=AXIS2_PLACEMENT_3D('',#101049,#79067,#79068) ;
#68644=AXIS2_PLACEMENT_3D('',#101050,#79069,#79070) ;
#68645=AXIS2_PLACEMENT_3D('',#101051,#79071,#79072) ;
#68646=AXIS2_PLACEMENT_3D('',#101052,#79073,#79074) ;
#68647=AXIS2_PLACEMENT_3D('',#101053,#79075,#79076) ;
#68648=AXIS2_PLACEMENT_3D('',#101054,#79077,#79078) ;
#68649=AXIS2_PLACEMENT_3D('',#101055,#79079,#79080) ;
#68650=AXIS2_PLACEMENT_3D('',#101056,#79081,#79082) ;
#68651=AXIS2_PLACEMENT_3D('',#101057,#79083,#79084) ;
#68652=AXIS2_PLACEMENT_3D('',#101058,#79085,#79086) ;
#68653=AXIS2_PLACEMENT_3D('',#101059,#79087,#79088) ;
#68654=AXIS2_PLACEMENT_3D('',#101060,#79089,#79090) ;
#68655=AXIS2_PLACEMENT_3D('',#101061,#79091,#79092) ;
#68656=AXIS2_PLACEMENT_3D('',#101062,#79093,#79094) ;
#68657=AXIS2_PLACEMENT_3D('',#101063,#79095,#79096) ;
#68658=AXIS2_PLACEMENT_3D('',#101064,#79097,#79098) ;
#68659=AXIS2_PLACEMENT_3D('',#101065,#79099,#79100) ;
#68660=AXIS2_PLACEMENT_3D('',#101066,#79101,#79102) ;
#68661=AXIS2_PLACEMENT_3D('',#101067,#79103,#79104) ;
#68662=AXIS2_PLACEMENT_3D('',#101068,#79105,#79106) ;
#68663=AXIS2_PLACEMENT_3D('',#101069,#79107,#79108) ;
#68664=AXIS2_PLACEMENT_3D('',#101070,#79109,#79110) ;
#68665=AXIS2_PLACEMENT_3D('',#101071,#79111,#79112) ;
#68666=AXIS2_PLACEMENT_3D('',#101072,#79113,#79114) ;
#68667=AXIS2_PLACEMENT_3D('',#101073,#79115,#79116) ;
#68668=AXIS2_PLACEMENT_3D('',#101074,#79117,#79118) ;
#68669=AXIS2_PLACEMENT_3D('',#101075,#79119,#79120) ;
#68670=AXIS2_PLACEMENT_3D('',#101076,#79121,#79122) ;
#68671=AXIS2_PLACEMENT_3D('',#101077,#79123,#79124) ;
#68672=AXIS2_PLACEMENT_3D('',#101078,#79125,#79126) ;
#68673=AXIS2_PLACEMENT_3D('',#101079,#79127,#79128) ;
#68674=AXIS2_PLACEMENT_3D('',#101080,#79129,#79130) ;
#68675=AXIS2_PLACEMENT_3D('',#101081,#79131,#79132) ;
#68676=AXIS2_PLACEMENT_3D('',#101082,#79133,#79134) ;
#68677=AXIS2_PLACEMENT_3D('',#101083,#79135,#79136) ;
#68678=AXIS2_PLACEMENT_3D('',#101084,#79137,#79138) ;
#68679=AXIS2_PLACEMENT_3D('',#101085,#79139,#79140) ;
#68680=AXIS2_PLACEMENT_3D('',#101086,#79141,#79142) ;
#68681=AXIS2_PLACEMENT_3D('',#101087,#79143,#79144) ;
#68682=AXIS2_PLACEMENT_3D('',#101088,#79145,#79146) ;
#68683=AXIS2_PLACEMENT_3D('',#101089,#79147,#79148) ;
#68684=AXIS2_PLACEMENT_3D('',#101090,#79149,#79150) ;
#68685=AXIS2_PLACEMENT_3D('',#101091,#79151,#79152) ;
#68686=AXIS2_PLACEMENT_3D('',#101092,#79153,#79154) ;
#68687=AXIS2_PLACEMENT_3D('',#101093,#79155,#79156) ;
#68688=AXIS2_PLACEMENT_3D('',#101094,#79157,#79158) ;
#68689=AXIS2_PLACEMENT_3D('',#101095,#79159,#79160) ;
#68690=AXIS2_PLACEMENT_3D('',#101096,#79161,#79162) ;
#68691=AXIS2_PLACEMENT_3D('',#101097,#79163,#79164) ;
#68692=AXIS2_PLACEMENT_3D('',#101098,#79165,#79166) ;
#68693=AXIS2_PLACEMENT_3D('',#101099,#79167,#79168) ;
#68694=AXIS2_PLACEMENT_3D('',#101100,#79169,#79170) ;
#68695=AXIS2_PLACEMENT_3D('',#101101,#79171,#79172) ;
#68696=AXIS2_PLACEMENT_3D('',#101102,#79173,#79174) ;
#68697=AXIS2_PLACEMENT_3D('',#101103,#79175,#79176) ;
#68698=AXIS2_PLACEMENT_3D('',#101104,#79177,#79178) ;
#68699=AXIS2_PLACEMENT_3D('',#101105,#79179,#79180) ;
#68700=AXIS2_PLACEMENT_3D('',#101106,#79181,#79182) ;
#68701=AXIS2_PLACEMENT_3D('',#101107,#79183,#79184) ;
#68702=AXIS2_PLACEMENT_3D('',#101108,#79185,#79186) ;
#68703=AXIS2_PLACEMENT_3D('',#101109,#79187,#79188) ;
#68704=AXIS2_PLACEMENT_3D('',#101110,#79189,#79190) ;
#68705=AXIS2_PLACEMENT_3D('',#101111,#79191,#79192) ;
#68706=AXIS2_PLACEMENT_3D('',#101112,#79193,#79194) ;
#68707=AXIS2_PLACEMENT_3D('',#101113,#79195,#79196) ;
#68708=AXIS2_PLACEMENT_3D('',#101114,#79197,#79198) ;
#68709=AXIS2_PLACEMENT_3D('',#101115,#79199,#79200) ;
#68710=AXIS2_PLACEMENT_3D('',#101116,#79201,#79202) ;
#68711=AXIS2_PLACEMENT_3D('',#101117,#79203,#79204) ;
#68712=AXIS2_PLACEMENT_3D('',#101118,#79205,#79206) ;
#68713=AXIS2_PLACEMENT_3D('',#101119,#79207,#79208) ;
#68714=AXIS2_PLACEMENT_3D('',#101120,#79209,#79210) ;
#68715=AXIS2_PLACEMENT_3D('',#101121,#79211,#79212) ;
#68716=AXIS2_PLACEMENT_3D('',#101122,#79213,#79214) ;
#68717=AXIS2_PLACEMENT_3D('',#101123,#79215,#79216) ;
#68718=AXIS2_PLACEMENT_3D('',#101124,#79217,#79218) ;
#68719=AXIS2_PLACEMENT_3D('',#101125,#79219,#79220) ;
#68720=AXIS2_PLACEMENT_3D('',#101126,#79221,#79222) ;
#68721=AXIS2_PLACEMENT_3D('',#101127,#79223,#79224) ;
#68722=AXIS2_PLACEMENT_3D('',#101128,#79225,#79226) ;
#68723=AXIS2_PLACEMENT_3D('',#101129,#79227,#79228) ;
#68724=AXIS2_PLACEMENT_3D('',#101130,#79229,#79230) ;
#68725=AXIS2_PLACEMENT_3D('',#101131,#79231,#79232) ;
#68726=AXIS2_PLACEMENT_3D('',#101132,#79233,#79234) ;
#68727=AXIS2_PLACEMENT_3D('',#101133,#79235,#79236) ;
#68728=AXIS2_PLACEMENT_3D('',#101134,#79237,#79238) ;
#68729=AXIS2_PLACEMENT_3D('',#101135,#79239,#79240) ;
#68730=AXIS2_PLACEMENT_3D('',#101136,#79241,#79242) ;
#68731=AXIS2_PLACEMENT_3D('',#101137,#79243,#79244) ;
#68732=AXIS2_PLACEMENT_3D('',#101138,#79245,#79246) ;
#68733=AXIS2_PLACEMENT_3D('',#101139,#79247,#79248) ;
#68734=AXIS2_PLACEMENT_3D('',#101140,#79249,#79250) ;
#68735=AXIS2_PLACEMENT_3D('',#101141,#79251,#79252) ;
#68736=AXIS2_PLACEMENT_3D('',#101142,#79253,#79254) ;
#68737=AXIS2_PLACEMENT_3D('',#101143,#79255,#79256) ;
#68738=AXIS2_PLACEMENT_3D('',#101144,#79257,#79258) ;
#68739=AXIS2_PLACEMENT_3D('',#101145,#79259,#79260) ;
#68740=AXIS2_PLACEMENT_3D('',#101146,#79261,#79262) ;
#68741=AXIS2_PLACEMENT_3D('',#101147,#79263,#79264) ;
#68742=AXIS2_PLACEMENT_3D('',#101148,#79265,#79266) ;
#68743=AXIS2_PLACEMENT_3D('',#101149,#79267,#79268) ;
#68744=AXIS2_PLACEMENT_3D('',#101150,#79269,#79270) ;
#68745=AXIS2_PLACEMENT_3D('',#101151,#79271,#79272) ;
#68746=AXIS2_PLACEMENT_3D('',#101152,#79273,#79274) ;
#68747=AXIS2_PLACEMENT_3D('',#101153,#79275,#79276) ;
#68748=AXIS2_PLACEMENT_3D('',#101154,#79277,#79278) ;
#68749=AXIS2_PLACEMENT_3D('',#101155,#79279,#79280) ;
#68750=AXIS2_PLACEMENT_3D('',#101156,#79281,#79282) ;
#68751=AXIS2_PLACEMENT_3D('',#101157,#79283,#79284) ;
#68752=AXIS2_PLACEMENT_3D('',#101158,#79285,#79286) ;
#68753=AXIS2_PLACEMENT_3D('',#101159,#79287,#79288) ;
#68754=AXIS2_PLACEMENT_3D('',#101160,#79289,#79290) ;
#68755=AXIS2_PLACEMENT_3D('',#101161,#79291,#79292) ;
#68756=AXIS2_PLACEMENT_3D('',#101162,#79293,#79294) ;
#68757=AXIS2_PLACEMENT_3D('',#101163,#79295,#79296) ;
#68758=AXIS2_PLACEMENT_3D('',#101164,#79297,#79298) ;
#68759=AXIS2_PLACEMENT_3D('',#101165,#79299,#79300) ;
#68760=AXIS2_PLACEMENT_3D('',#101166,#79301,#79302) ;
#68761=AXIS2_PLACEMENT_3D('',#101167,#79303,#79304) ;
#68762=AXIS2_PLACEMENT_3D('',#101168,#79305,#79306) ;
#68763=AXIS2_PLACEMENT_3D('',#101169,#79307,#79308) ;
#68764=AXIS2_PLACEMENT_3D('',#101170,#79309,#79310) ;
#68765=AXIS2_PLACEMENT_3D('',#101171,#79311,#79312) ;
#68766=AXIS2_PLACEMENT_3D('',#101172,#79313,#79314) ;
#68767=AXIS2_PLACEMENT_3D('',#101173,#79315,#79316) ;
#68768=AXIS2_PLACEMENT_3D('',#101174,#79317,#79318) ;
#68769=AXIS2_PLACEMENT_3D('',#101175,#79319,#79320) ;
#68770=AXIS2_PLACEMENT_3D('',#101176,#79321,#79322) ;
#68771=AXIS2_PLACEMENT_3D('',#101177,#79323,#79324) ;
#68772=AXIS2_PLACEMENT_3D('',#101178,#79325,#79326) ;
#68773=AXIS2_PLACEMENT_3D('',#101179,#79327,#79328) ;
#68774=AXIS2_PLACEMENT_3D('',#101180,#79329,#79330) ;
#68775=AXIS2_PLACEMENT_3D('',#101181,#79331,#79332) ;
#68776=AXIS2_PLACEMENT_3D('',#101182,#79333,#79334) ;
#68777=AXIS2_PLACEMENT_3D('',#101183,#79335,#79336) ;
#76854=DIRECTION('axis',(0.,0.,1.)) ;
#76855=DIRECTION('refdir',(1.,0.,0.)) ;
#76856=DIRECTION('center_axis',(-1.,-3.65204942310907E-15,-6.7286639138916E-31)) ;
#76857=DIRECTION('ref_axis',(3.73969860926368E-15,-1.,0.)) ;
#76858=DIRECTION('center_axis',(-1.,-3.65204942310907E-15,-6.7286639138916E-31)) ;
#76859=DIRECTION('ref_axis',(3.65204942310907E-15,-1.,-4.60751496844179E-46)) ;
#76860=DIRECTION('center_axis',(-1.,-3.65204942310907E-15,-6.7286639138916E-31)) ;
#76861=DIRECTION('ref_axis',(3.65204942310907E-15,-1.,-4.60751496844179E-46)) ;
#76862=DIRECTION('center_axis',(6.7286639138916E-31,3.1453968851229E-45,
-1.)) ;
#76863=DIRECTION('ref_axis',(-4.67462326157961E-15,1.,0.)) ;
#76864=DIRECTION('center_axis',(1.,3.65204942310907E-15,6.7286639138916E-31)) ;
#76865=DIRECTION('ref_axis',(3.65204942310907E-15,-1.,-2.10629255700197E-46)) ;
#76866=DIRECTION('center_axis',(-1.,-3.65204942310907E-15,-6.7286639138916E-31)) ;
#76867=DIRECTION('ref_axis',(3.73969860926368E-15,-1.,0.)) ;
#76868=DIRECTION('center_axis',(-1.,-3.65204942310907E-15,-6.7286639138916E-31)) ;
#76869=DIRECTION('ref_axis',(3.65204942310907E-15,-1.,-2.10629255700197E-46)) ;
#76870=DIRECTION('center_axis',(6.7286639138916E-31,3.1453968851229E-45,
-1.)) ;
#76871=DIRECTION('ref_axis',(-4.67462326157961E-15,1.,0.)) ;
#76872=DIRECTION('center_axis',(1.,3.65204942310907E-15,6.7286639138916E-31)) ;
#76873=DIRECTION('ref_axis',(3.65204942310907E-15,-1.,-4.60751496844179E-46)) ;
#76874=DIRECTION('center_axis',(1.,3.65204942310907E-15,6.7286639138916E-31)) ;
#76875=DIRECTION('ref_axis',(3.65204942310907E-15,-1.,-4.60751496844179E-46)) ;
#76876=DIRECTION('center_axis',(0.,-1.,-1.83697019872103E-16)) ;
#76877=DIRECTION('ref_axis',(0.,1.8503717077086E-16,-1.)) ;
#76878=DIRECTION('center_axis',(0.,-1.,-1.83697019872103E-16)) ;
#76879=DIRECTION('ref_axis',(0.,1.83697019872103E-16,-1.)) ;
#76880=DIRECTION('center_axis',(0.,-1.,-1.83697019872103E-16)) ;
#76881=DIRECTION('ref_axis',(0.,1.83697019872103E-16,-1.)) ;
#76882=DIRECTION('center_axis',(-1.,0.,0.)) ;
#76883=DIRECTION('ref_axis',(0.,-1.92747052886313E-16,1.)) ;
#76884=DIRECTION('center_axis',(0.,1.,1.83697019872103E-16)) ;
#76885=DIRECTION('ref_axis',(0.,1.83697019872103E-16,-1.)) ;
#76886=DIRECTION('center_axis',(0.,1.,1.83697019872103E-16)) ;
#76887=DIRECTION('ref_axis',(0.,1.83697019872103E-16,-1.)) ;
#76888=DIRECTION('center_axis',(-4.15069017696469E-34,1.,1.83697019872103E-16)) ;
#76889=DIRECTION('ref_axis',(0.,-1.8503717077086E-16,1.)) ;
#76890=DIRECTION('center_axis',(-4.15069017696469E-34,1.,1.83697019872103E-16)) ;
#76891=DIRECTION('ref_axis',(-5.57464581117898E-51,-1.83697019872103E-16,
1.)) ;
#76892=DIRECTION('center_axis',(-1.,-4.15069017696469E-34,-8.00033299054114E-50)) ;
#76893=DIRECTION('ref_axis',(0.,1.92747052886313E-16,-1.)) ;
#76894=DIRECTION('center_axis',(4.15069017696469E-34,-1.,-1.83697019872103E-16)) ;
#76895=DIRECTION('ref_axis',(-1.3756804551505E-50,-1.83697019872103E-16,
1.)) ;
#76896=DIRECTION('center_axis',(0.,-1.,-1.83697019872103E-16)) ;
#76897=DIRECTION('ref_axis',(0.,1.8503717077086E-16,-1.)) ;
#76898=DIRECTION('center_axis',(0.,-1.,-1.83697019872103E-16)) ;
#76899=DIRECTION('ref_axis',(0.,1.83697019872103E-16,-1.)) ;
#76900=DIRECTION('center_axis',(0.,-1.,-1.83697019872103E-16)) ;
#76901=DIRECTION('ref_axis',(0.,1.83697019872103E-16,-1.)) ;
#76902=DIRECTION('center_axis',(-1.,0.,0.)) ;
#76903=DIRECTION('ref_axis',(0.,-1.92747052886313E-16,1.)) ;
#76904=DIRECTION('center_axis',(0.,1.,1.83697019872103E-16)) ;
#76905=DIRECTION('ref_axis',(0.,1.83697019872103E-16,-1.)) ;
#76906=DIRECTION('center_axis',(0.,1.,1.83697019872103E-16)) ;
#76907=DIRECTION('ref_axis',(0.,1.83697019872103E-16,-1.)) ;
#76908=DIRECTION('center_axis',(-4.15069017696469E-34,1.,1.83697019872103E-16)) ;
#76909=DIRECTION('ref_axis',(0.,-1.8503717077086E-16,1.)) ;
#76910=DIRECTION('center_axis',(-4.15069017696469E-34,1.,1.83697019872103E-16)) ;
#76911=DIRECTION('ref_axis',(-5.57464581117898E-51,-1.83697019872103E-16,
1.)) ;
#76912=DIRECTION('center_axis',(-1.,-4.15069017696469E-34,-8.00033299054114E-50)) ;
#76913=DIRECTION('ref_axis',(0.,1.92747052886313E-16,-1.)) ;
#76914=DIRECTION('center_axis',(4.15069017696469E-34,-1.,-1.83697019872103E-16)) ;
#76915=DIRECTION('ref_axis',(-1.3756804551505E-50,-1.83697019872103E-16,
1.)) ;
#76916=DIRECTION('center_axis',(0.,1.,1.83697019872103E-16)) ;
#76917=DIRECTION('ref_axis',(0.,-1.83697019872103E-16,1.)) ;
#76918=DIRECTION('',(-8.65956056235478E-17,0.70710678118656,-0.707106781186535)) ;
#76919=DIRECTION('center_axis',(0.,1.,1.83697019872103E-16)) ;
#76920=DIRECTION('ref_axis',(0.,-1.83697019872103E-16,1.)) ;
#76921=DIRECTION('center_axis',(0.,1.,1.83697019872103E-16)) ;
#76922=DIRECTION('ref_axis',(0.,-1.83697019872103E-16,1.)) ;
#76923=DIRECTION('',(0.,1.,1.83697019872103E-16)) ;
#76924=DIRECTION('center_axis',(0.,1.,1.83697019872103E-16)) ;
#76925=DIRECTION('ref_axis',(0.,-1.83697019872103E-16,1.)) ;
#76926=DIRECTION('',(-8.65956056235478E-17,0.70710678118656,-0.707106781186535)) ;
#76927=DIRECTION('center_axis',(0.,1.,1.83697019872103E-16)) ;
#76928=DIRECTION('ref_axis',(0.,-1.83697019872103E-16,1.)) ;
#76929=DIRECTION('center_axis',(0.,1.,1.83697019872103E-16)) ;
#76930=DIRECTION('ref_axis',(0.,-1.83697019872103E-16,1.)) ;
#76931=DIRECTION('',(0.,1.,1.83697019872103E-16)) ;
#76932=DIRECTION('center_axis',(1.,3.65204942310907E-15,6.7286639138916E-31)) ;
#76933=DIRECTION('ref_axis',(-3.65204942310907E-15,1.,-8.63909056582784E-47)) ;
#76934=DIRECTION('',(1.,3.65204942310907E-15,6.7286639138916E-31)) ;
#76935=DIRECTION('center_axis',(-1.,-3.65204942310907E-15,-6.7286639138916E-31)) ;
#76936=DIRECTION('ref_axis',(3.65204942310907E-15,-1.,-1.30970071666515E-61)) ;
#76937=DIRECTION('',(0.,-2.47817639425257E-16,1.)) ;
#76938=DIRECTION('',(3.65204942310907E-15,-1.,1.22867065825113E-46)) ;
#76939=DIRECTION('',(1.03517906367563E-32,1.81408990951823E-16,-1.)) ;
#76940=DIRECTION('',(-3.65204942310907E-15,1.,7.70988211545247E-16)) ;
#76941=DIRECTION('',(0.,2.47817639425258E-16,-1.)) ;
#76942=DIRECTION('',(1.03517906367563E-32,1.81408990951823E-16,-1.)) ;
#76943=DIRECTION('center_axis',(1.,3.65204942310907E-15,6.7286639138916E-31)) ;
#76944=DIRECTION('ref_axis',(3.65204942310907E-15,-1.,2.45734131650226E-45)) ;
#76945=DIRECTION('',(3.65204942310907E-15,-1.,-3.44027784310316E-46)) ;
#76946=DIRECTION('center_axis',(1.,3.65204942310907E-15,6.7286639138916E-31)) ;
#76947=DIRECTION('ref_axis',(3.65204942310907E-15,-1.,2.45734131650226E-45)) ;
#76948=DIRECTION('',(-6.7286639138916E-31,-2.45734131650226E-45,1.)) ;
#76949=DIRECTION('center_axis',(1.,3.65204942310907E-15,6.7286639138916E-31)) ;
#76950=DIRECTION('ref_axis',(3.65204942310907E-15,-1.,2.45734131650226E-45)) ;
#76951=DIRECTION('',(-3.65204942310907E-15,1.,3.44027784310316E-46)) ;
#76952=DIRECTION('center_axis',(1.,3.65204942310907E-15,6.7286639138916E-31)) ;
#76953=DIRECTION('ref_axis',(3.65204942310907E-15,-1.,2.45734131650226E-45)) ;
#76954=DIRECTION('',(6.7286639138916E-31,2.45734131650226E-45,-1.)) ;
#76955=DIRECTION('center_axis',(-1.,-3.65204942310907E-15,-6.7286639138916E-31)) ;
#76956=DIRECTION('ref_axis',(3.65204942310907E-15,-1.,-1.30970071666515E-61)) ;
#76957=DIRECTION('',(-1.03517906367563E-32,-1.81408990951823E-16,1.)) ;
#76958=DIRECTION('',(-3.65204942310907E-15,1.,-1.22867065825113E-46)) ;
#76959=DIRECTION('',(0.,-2.47817639425257E-16,1.)) ;
#76960=DIRECTION('',(0.,-1.81408990951823E-16,1.)) ;
#76961=DIRECTION('',(0.,2.47817639425258E-16,-1.)) ;
#76962=DIRECTION('',(3.65204942310907E-15,-1.,-7.70988211545247E-16)) ;
#76963=DIRECTION('center_axis',(-1.,-3.65204942310907E-15,-6.7286639138916E-31)) ;
#76964=DIRECTION('ref_axis',(3.65204942310907E-15,-1.,2.45734131650226E-45)) ;
#76965=DIRECTION('',(-3.65204942310907E-15,1.,3.44027784310316E-46)) ;
#76966=DIRECTION('center_axis',(-1.,-3.65204942310907E-15,-6.7286639138916E-31)) ;
#76967=DIRECTION('ref_axis',(3.65204942310907E-15,-1.,2.45734131650226E-45)) ;
#76968=DIRECTION('',(-6.7286639138916E-31,-2.45734131650226E-45,1.)) ;
#76969=DIRECTION('center_axis',(-1.,-3.65204942310907E-15,-6.7286639138916E-31)) ;
#76970=DIRECTION('ref_axis',(3.65204942310907E-15,-1.,2.45734131650226E-45)) ;
#76971=DIRECTION('',(3.65204942310907E-15,-1.,-3.44027784310316E-46)) ;
#76972=DIRECTION('center_axis',(-1.,-3.65204942310907E-15,-6.7286639138916E-31)) ;
#76973=DIRECTION('ref_axis',(3.65204942310907E-15,-1.,2.45734131650226E-45)) ;
#76974=DIRECTION('',(6.7286639138916E-31,2.45734131650226E-45,-1.)) ;
#76975=DIRECTION('center_axis',(4.72515227845561E-31,7.02672800395669E-16,
-1.)) ;
#76976=DIRECTION('ref_axis',(2.70755867152026E-31,1.,7.02672800395669E-16)) ;
#76977=DIRECTION('center_axis',(4.72515227845561E-31,7.02672800395669E-16,
-1.)) ;
#76978=DIRECTION('ref_axis',(-3.32023598379838E-46,1.,7.02672800395669E-16)) ;
#76979=DIRECTION('',(-7.43707788821665E-32,1.,7.02672800395669E-16)) ;
#76980=DIRECTION('',(-1.,-7.43707788821671E-32,8.21355058201474E-31)) ;
#76981=DIRECTION('',(-1.,-7.43707788821671E-32,8.21355058201474E-31)) ;
#76982=DIRECTION('',(3.49501116159781E-15,-1.,-7.02672800395669E-16)) ;
#76983=DIRECTION('',(-1.,4.18667286880966E-31,-4.7251522784556E-31)) ;
#76984=DIRECTION('',(-7.43707788821665E-32,1.,7.02672800395669E-16)) ;
#76985=DIRECTION('center_axis',(4.72515227845561E-31,7.02672800395669E-16,
-1.)) ;
#76986=DIRECTION('ref_axis',(-3.32023598379838E-46,1.,7.02672800395669E-16)) ;
#76987=DIRECTION('',(-1.,4.18667286880966E-31,-4.7251522784556E-31)) ;
#76988=DIRECTION('',(-2.16840434497101E-16,1.,7.02672800395669E-16)) ;
#76989=DIRECTION('',(1.,-4.18667286880966E-31,4.7251522784556E-31)) ;
#76990=DIRECTION('center_axis',(4.72515227845561E-31,7.02672800395669E-16,
-1.)) ;
#76991=DIRECTION('ref_axis',(-3.32023598379838E-46,1.,7.02672800395669E-16)) ;
#76992=DIRECTION('',(1.97633094273713E-47,-1.,-7.02672800395669E-16)) ;
#76993=DIRECTION('center_axis',(4.72515227845561E-31,7.02672800395669E-16,
-1.)) ;
#76994=DIRECTION('ref_axis',(-3.32023598379838E-46,1.,7.02672800395669E-16)) ;
#76995=DIRECTION('',(1.,-3.32023598379838E-46,4.72515227845561E-31)) ;
#76996=DIRECTION('center_axis',(4.72515227845561E-31,7.02672800395669E-16,
-1.)) ;
#76997=DIRECTION('ref_axis',(-3.32023598379838E-46,1.,7.02672800395669E-16)) ;
#76998=DIRECTION('',(-1.97633094273713E-47,1.,7.02672800395669E-16)) ;
#76999=DIRECTION('center_axis',(4.72515227845561E-31,7.02672800395669E-16,
-1.)) ;
#77000=DIRECTION('ref_axis',(-3.32023598379838E-46,1.,7.02672800395669E-16)) ;
#77001=DIRECTION('',(-1.,3.32023598379838E-46,-4.72515227845561E-31)) ;
#77002=DIRECTION('center_axis',(4.72515227845561E-31,7.02672800395669E-16,
-1.)) ;
#77003=DIRECTION('ref_axis',(-3.32023598379838E-46,1.,7.02672800395669E-16)) ;
#77004=DIRECTION('',(-8.67361737988404E-17,-1.,-7.02672800395669E-16)) ;
#77005=DIRECTION('center_axis',(4.72515227845561E-31,7.02672800395669E-16,
-1.)) ;
#77006=DIRECTION('ref_axis',(-3.32023598379838E-46,1.,7.02672800395669E-16)) ;
#77007=DIRECTION('',(1.,-3.32023598379838E-46,4.72515227845561E-31)) ;
#77008=DIRECTION('center_axis',(4.72515227845561E-31,7.02672800395669E-16,
-1.)) ;
#77009=DIRECTION('ref_axis',(-3.32023598379838E-46,1.,7.02672800395669E-16)) ;
#77010=DIRECTION('',(1.73472347597681E-16,1.,7.02672800395669E-16)) ;
#77011=DIRECTION('center_axis',(4.72515227845561E-31,7.02672800395669E-16,
-1.)) ;
#77012=DIRECTION('ref_axis',(-3.32023598379838E-46,1.,7.02672800395669E-16)) ;
#77013=DIRECTION('',(-1.,3.32023598379838E-46,-4.72515227845561E-31)) ;
#77014=DIRECTION('center_axis',(4.72515227845561E-31,7.02672800395669E-16,
-1.)) ;
#77015=DIRECTION('ref_axis',(-3.32023598379838E-46,1.,7.02672800395669E-16)) ;
#77016=DIRECTION('',(3.46944695195361E-16,1.,7.02672800395669E-16)) ;
#77017=DIRECTION('center_axis',(4.72515227845561E-31,7.02672800395669E-16,
-1.)) ;
#77018=DIRECTION('ref_axis',(-3.32023598379838E-46,1.,7.02672800395669E-16)) ;
#77019=DIRECTION('',(-1.,3.32023598379838E-46,-4.72515227845561E-31)) ;
#77020=DIRECTION('center_axis',(4.72515227845561E-31,7.02672800395669E-16,
-1.)) ;
#77021=DIRECTION('ref_axis',(-3.32023598379838E-46,1.,7.02672800395669E-16)) ;
#77022=DIRECTION('',(-1.73472347597681E-16,-1.,-7.02672800395669E-16)) ;
#77023=DIRECTION('center_axis',(4.72515227845561E-31,7.02672800395669E-16,
-1.)) ;
#77024=DIRECTION('ref_axis',(-3.32023598379838E-46,1.,7.02672800395669E-16)) ;
#77025=DIRECTION('',(1.,-3.32023598379838E-46,4.72515227845561E-31)) ;
#77026=DIRECTION('center_axis',(4.72515227845561E-31,7.02672800395669E-16,
-1.)) ;
#77027=DIRECTION('ref_axis',(-3.32023598379838E-46,1.,7.02672800395669E-16)) ;
#77028=DIRECTION('',(6.93889390390723E-16,1.,7.02672800395669E-16)) ;
#77029=DIRECTION('center_axis',(4.72515227845561E-31,7.02672800395669E-16,
-1.)) ;
#77030=DIRECTION('ref_axis',(-3.32023598379838E-46,1.,7.02672800395669E-16)) ;
#77031=DIRECTION('',(-1.,3.32023598379838E-46,-4.72515227845561E-31)) ;
#77032=DIRECTION('center_axis',(4.72515227845561E-31,7.02672800395669E-16,
-1.)) ;
#77033=DIRECTION('ref_axis',(-3.32023598379838E-46,1.,7.02672800395669E-16)) ;
#77034=DIRECTION('',(4.15029497974802E-48,-1.,-7.02672800395669E-16)) ;
#77035=DIRECTION('center_axis',(4.72515227845561E-31,7.02672800395669E-16,
-1.)) ;
#77036=DIRECTION('ref_axis',(-3.32023598379838E-46,1.,7.02672800395669E-16)) ;
#77037=DIRECTION('',(1.,-3.32023598379838E-46,4.72515227845561E-31)) ;
#77038=DIRECTION('center_axis',(4.72515227845561E-31,7.02672800395669E-16,
-1.)) ;
#77039=DIRECTION('ref_axis',(2.70755867152026E-31,1.,7.02672800395669E-16)) ;
#77040=DIRECTION('',(-1.,-7.43707788821671E-32,8.21355058201474E-31)) ;
#77041=DIRECTION('',(7.43707788821665E-32,-1.,-7.02672800395669E-16)) ;
#77042=DIRECTION('center_axis',(-4.72515227845561E-31,-7.02672800395669E-16,
1.)) ;
#77043=DIRECTION('ref_axis',(-3.32023598379838E-46,1.,7.02672800395669E-16)) ;
#77044=DIRECTION('',(-1.,4.18667286880966E-31,-4.7251522784556E-31)) ;
#77045=DIRECTION('',(2.16840434497101E-16,-1.,-7.02672800395669E-16)) ;
#77046=DIRECTION('',(1.,-4.18667286880966E-31,4.7251522784556E-31)) ;
#77047=DIRECTION('center_axis',(-4.72515227845561E-31,-7.02672800395669E-16,
1.)) ;
#77048=DIRECTION('ref_axis',(-3.32023598379838E-46,1.,7.02672800395669E-16)) ;
#77049=DIRECTION('',(7.43707788821665E-32,-1.,-7.02672800395669E-16)) ;
#77050=DIRECTION('',(1.,-4.18667286880966E-31,4.7251522784556E-31)) ;
#77051=DIRECTION('',(-3.49501116159781E-15,1.,7.02672800395669E-16)) ;
#77052=DIRECTION('',(-1.,-7.43707788821671E-32,8.21355058201474E-31)) ;
#77053=DIRECTION('center_axis',(-4.72515227845561E-31,-7.02672800395669E-16,
1.)) ;
#77054=DIRECTION('ref_axis',(-3.32023598379838E-46,1.,7.02672800395669E-16)) ;
#77055=DIRECTION('',(-1.97633094273713E-47,1.,7.02672800395669E-16)) ;
#77056=DIRECTION('center_axis',(-4.72515227845561E-31,-7.02672800395669E-16,
1.)) ;
#77057=DIRECTION('ref_axis',(-3.32023598379838E-46,1.,7.02672800395669E-16)) ;
#77058=DIRECTION('',(1.,-3.32023598379838E-46,4.72515227845561E-31)) ;
#77059=DIRECTION('center_axis',(-4.72515227845561E-31,-7.02672800395669E-16,
1.)) ;
#77060=DIRECTION('ref_axis',(-3.32023598379838E-46,1.,7.02672800395669E-16)) ;
#77061=DIRECTION('',(1.97633094273713E-47,-1.,-7.02672800395669E-16)) ;
#77062=DIRECTION('center_axis',(-4.72515227845561E-31,-7.02672800395669E-16,
1.)) ;
#77063=DIRECTION('ref_axis',(-3.32023598379838E-46,1.,7.02672800395669E-16)) ;
#77064=DIRECTION('',(-1.,3.32023598379838E-46,-4.72515227845561E-31)) ;
#77065=DIRECTION('center_axis',(-4.72515227845561E-31,-7.02672800395669E-16,
1.)) ;
#77066=DIRECTION('ref_axis',(-3.32023598379838E-46,1.,7.02672800395669E-16)) ;
#77067=DIRECTION('',(8.67361737988404E-17,1.,7.02672800395669E-16)) ;
#77068=DIRECTION('center_axis',(-4.72515227845561E-31,-7.02672800395669E-16,
1.)) ;
#77069=DIRECTION('ref_axis',(-3.32023598379838E-46,1.,7.02672800395669E-16)) ;
#77070=DIRECTION('',(1.,-3.32023598379838E-46,4.72515227845561E-31)) ;
#77071=DIRECTION('center_axis',(-4.72515227845561E-31,-7.02672800395669E-16,
1.)) ;
#77072=DIRECTION('ref_axis',(-3.32023598379838E-46,1.,7.02672800395669E-16)) ;
#77073=DIRECTION('',(-1.73472347597681E-16,-1.,-7.02672800395669E-16)) ;
#77074=DIRECTION('center_axis',(-4.72515227845561E-31,-7.02672800395669E-16,
1.)) ;
#77075=DIRECTION('ref_axis',(-3.32023598379838E-46,1.,7.02672800395669E-16)) ;
#77076=DIRECTION('',(-1.,3.32023598379838E-46,-4.72515227845561E-31)) ;
#77077=DIRECTION('center_axis',(-4.72515227845561E-31,-7.02672800395669E-16,
1.)) ;
#77078=DIRECTION('ref_axis',(-3.32023598379838E-46,1.,7.02672800395669E-16)) ;
#77079=DIRECTION('',(-3.46944695195361E-16,-1.,-7.02672800395669E-16)) ;
#77080=DIRECTION('center_axis',(-4.72515227845561E-31,-7.02672800395669E-16,
1.)) ;
#77081=DIRECTION('ref_axis',(-3.32023598379838E-46,1.,7.02672800395669E-16)) ;
#77082=DIRECTION('',(-1.,3.32023598379838E-46,-4.72515227845561E-31)) ;
#77083=DIRECTION('center_axis',(-4.72515227845561E-31,-7.02672800395669E-16,
1.)) ;
#77084=DIRECTION('ref_axis',(-3.32023598379838E-46,1.,7.02672800395669E-16)) ;
#77085=DIRECTION('',(1.73472347597681E-16,1.,7.02672800395669E-16)) ;
#77086=DIRECTION('center_axis',(-4.72515227845561E-31,-7.02672800395669E-16,
1.)) ;
#77087=DIRECTION('ref_axis',(-3.32023598379838E-46,1.,7.02672800395669E-16)) ;
#77088=DIRECTION('',(1.,-3.32023598379838E-46,4.72515227845561E-31)) ;
#77089=DIRECTION('center_axis',(-4.72515227845561E-31,-7.02672800395669E-16,
1.)) ;
#77090=DIRECTION('ref_axis',(-3.32023598379838E-46,1.,7.02672800395669E-16)) ;
#77091=DIRECTION('',(-6.93889390390723E-16,-1.,-7.02672800395669E-16)) ;
#77092=DIRECTION('center_axis',(-4.72515227845561E-31,-7.02672800395669E-16,
1.)) ;
#77093=DIRECTION('ref_axis',(-3.32023598379838E-46,1.,7.02672800395669E-16)) ;
#77094=DIRECTION('',(-1.,3.32023598379838E-46,-4.72515227845561E-31)) ;
#77095=DIRECTION('center_axis',(-4.72515227845561E-31,-7.02672800395669E-16,
1.)) ;
#77096=DIRECTION('ref_axis',(-3.32023598379838E-46,1.,7.02672800395669E-16)) ;
#77097=DIRECTION('',(-4.15029497974802E-48,1.,7.02672800395669E-16)) ;
#77098=DIRECTION('center_axis',(-4.72515227845561E-31,-7.02672800395669E-16,
1.)) ;
#77099=DIRECTION('ref_axis',(-3.32023598379838E-46,1.,7.02672800395669E-16)) ;
#77100=DIRECTION('',(1.,-3.32023598379838E-46,4.72515227845561E-31)) ;
#77101=DIRECTION('center_axis',(-8.13512808509168E-31,-3.26576826218999E-61,
1.)) ;
#77102=DIRECTION('ref_axis',(1.,4.27339674608664E-31,8.13512808509168E-31)) ;
#77103=DIRECTION('',(-1.,-4.27339674608664E-31,-8.13512808509168E-31)) ;
#77104=DIRECTION('',(4.27339674608664E-31,-1.,2.10694726592902E-62)) ;
#77105=DIRECTION('center_axis',(-4.93038065763132E-32,0.,1.)) ;
#77106=DIRECTION('ref_axis',(1.,0.,4.93038065763132E-32)) ;
#77107=DIRECTION('',(-1.,4.27339674608665E-31,-4.93038065763132E-32)) ;
#77108=DIRECTION('',(2.16840434497101E-16,-1.,1.06910588403688E-47)) ;
#77109=DIRECTION('',(1.,-4.27339674608665E-31,4.93038065763132E-32)) ;
#77110=DIRECTION('center_axis',(-4.93038065763132E-32,0.,1.)) ;
#77111=DIRECTION('ref_axis',(1.,0.,4.93038065763132E-32)) ;
#77112=DIRECTION('',(4.27339674608664E-31,-1.,2.10694726592902E-62)) ;
#77113=DIRECTION('',(1.,-4.27339674608665E-31,4.93038065763132E-32)) ;
#77114=DIRECTION('',(-3.49247269410375E-15,1.,-1.72192198183147E-46)) ;
#77115=DIRECTION('',(-1.,-4.27339674608664E-31,-8.13512808509168E-31)) ;
#77116=DIRECTION('center_axis',(-4.93038065763132E-32,0.,1.)) ;
#77117=DIRECTION('ref_axis',(1.,0.,4.93038065763132E-32)) ;
#77118=DIRECTION('',(1.73472347597681E-16,-1.,8.55284707229503E-48)) ;
#77119=DIRECTION('center_axis',(-4.93038065763132E-32,0.,1.)) ;
#77120=DIRECTION('ref_axis',(1.,0.,4.93038065763132E-32)) ;
#77121=DIRECTION('',(-1.,0.,-4.93038065763132E-32)) ;
#77122=DIRECTION('center_axis',(-4.93038065763132E-32,0.,1.)) ;
#77123=DIRECTION('ref_axis',(1.,0.,4.93038065763132E-32)) ;
#77124=DIRECTION('',(-2.60208521396521E-16,1.,-1.28292706084425E-47)) ;
#77125=DIRECTION('center_axis',(-4.93038065763132E-32,0.,1.)) ;
#77126=DIRECTION('ref_axis',(1.,0.,4.93038065763132E-32)) ;
#77127=DIRECTION('',(1.,0.,4.93038065763132E-32)) ;
#77128=DIRECTION('center_axis',(-4.93038065763132E-32,0.,1.)) ;
#77129=DIRECTION('ref_axis',(1.,0.,4.93038065763132E-32)) ;
#77130=DIRECTION('',(0.,-1.,0.)) ;
#77131=DIRECTION('center_axis',(-4.93038065763132E-32,0.,1.)) ;
#77132=DIRECTION('ref_axis',(1.,0.,4.93038065763132E-32)) ;
#77133=DIRECTION('',(-1.,0.,-4.93038065763132E-32)) ;
#77134=DIRECTION('center_axis',(-4.93038065763132E-32,0.,1.)) ;
#77135=DIRECTION('ref_axis',(1.,0.,4.93038065763132E-32)) ;
#77136=DIRECTION('',(-3.46944695195361E-16,1.,-1.71056941445901E-47)) ;
#77137=DIRECTION('center_axis',(-4.93038065763132E-32,0.,1.)) ;
#77138=DIRECTION('ref_axis',(1.,0.,4.93038065763132E-32)) ;
#77139=DIRECTION('',(1.,0.,4.93038065763132E-32)) ;
#77140=DIRECTION('center_axis',(-4.93038065763132E-32,0.,1.)) ;
#77141=DIRECTION('ref_axis',(1.,0.,4.93038065763132E-32)) ;
#77142=DIRECTION('',(6.93889390390723E-16,-1.,3.42113882891801E-47)) ;
#77143=DIRECTION('center_axis',(-4.93038065763132E-32,0.,1.)) ;
#77144=DIRECTION('ref_axis',(1.,0.,4.93038065763132E-32)) ;
#77145=DIRECTION('',(-1.,0.,-4.93038065763132E-32)) ;
#77146=DIRECTION('center_axis',(-4.93038065763132E-32,0.,1.)) ;
#77147=DIRECTION('ref_axis',(1.,0.,4.93038065763132E-32)) ;
#77148=DIRECTION('',(0.,1.,0.)) ;
#77149=DIRECTION('center_axis',(-4.93038065763132E-32,0.,1.)) ;
#77150=DIRECTION('ref_axis',(1.,0.,4.93038065763132E-32)) ;
#77151=DIRECTION('',(1.,0.,4.93038065763132E-32)) ;
#77152=DIRECTION('center_axis',(-4.93038065763132E-32,0.,1.)) ;
#77153=DIRECTION('ref_axis',(1.,0.,4.93038065763132E-32)) ;
#77154=DIRECTION('',(0.,-1.,0.)) ;
#77155=DIRECTION('center_axis',(-4.93038065763132E-32,0.,1.)) ;
#77156=DIRECTION('ref_axis',(1.,0.,4.93038065763132E-32)) ;
#77157=DIRECTION('',(-1.,0.,-4.93038065763132E-32)) ;
#77158=DIRECTION('center_axis',(-4.93038065763132E-32,0.,1.)) ;
#77159=DIRECTION('ref_axis',(1.,0.,4.93038065763132E-32)) ;
#77160=DIRECTION('',(0.,1.,0.)) ;
#77161=DIRECTION('center_axis',(-4.93038065763132E-32,0.,1.)) ;
#77162=DIRECTION('ref_axis',(1.,0.,4.93038065763132E-32)) ;
#77163=DIRECTION('',(1.,0.,4.93038065763132E-32)) ;
#77164=DIRECTION('center_axis',(-4.93038065763132E-32,0.,1.)) ;
#77165=DIRECTION('ref_axis',(1.,0.,4.93038065763132E-32)) ;
#77166=DIRECTION('',(0.,-1.,0.)) ;
#77167=DIRECTION('center_axis',(-4.93038065763132E-32,0.,1.)) ;
#77168=DIRECTION('ref_axis',(1.,0.,4.93038065763132E-32)) ;
#77169=DIRECTION('',(-1.,0.,-4.93038065763132E-32)) ;
#77170=DIRECTION('center_axis',(-4.93038065763132E-32,0.,1.)) ;
#77171=DIRECTION('ref_axis',(1.,0.,4.93038065763132E-32)) ;
#77172=DIRECTION('',(0.,1.,0.)) ;
#77173=DIRECTION('center_axis',(-4.93038065763132E-32,0.,1.)) ;
#77174=DIRECTION('ref_axis',(1.,0.,4.93038065763132E-32)) ;
#77175=DIRECTION('',(1.,0.,4.93038065763132E-32)) ;
#77176=DIRECTION('center_axis',(-4.93038065763132E-32,0.,1.)) ;
#77177=DIRECTION('ref_axis',(1.,0.,4.93038065763132E-32)) ;
#77178=DIRECTION('',(3.46944695195361E-16,-1.,1.71056941445901E-47)) ;
#77179=DIRECTION('center_axis',(-4.93038065763132E-32,0.,1.)) ;
#77180=DIRECTION('ref_axis',(1.,0.,4.93038065763132E-32)) ;
#77181=DIRECTION('',(-1.,0.,-4.93038065763132E-32)) ;
#77182=DIRECTION('center_axis',(-4.93038065763132E-32,0.,1.)) ;
#77183=DIRECTION('ref_axis',(1.,0.,4.93038065763132E-32)) ;
#77184=DIRECTION('',(0.,1.,0.)) ;
#77185=DIRECTION('center_axis',(-4.93038065763132E-32,0.,1.)) ;
#77186=DIRECTION('ref_axis',(1.,0.,4.93038065763132E-32)) ;
#77187=DIRECTION('',(1.,0.,4.93038065763132E-32)) ;
#77188=DIRECTION('center_axis',(-4.93038065763132E-32,0.,1.)) ;
#77189=DIRECTION('ref_axis',(1.,0.,4.93038065763132E-32)) ;
#77190=DIRECTION('',(-3.46944695195361E-16,1.,-1.71056941445901E-47)) ;
#77191=DIRECTION('center_axis',(-4.93038065763132E-32,0.,1.)) ;
#77192=DIRECTION('ref_axis',(1.,0.,4.93038065763132E-32)) ;
#77193=DIRECTION('',(1.,0.,4.93038065763132E-32)) ;
#77194=DIRECTION('center_axis',(-4.93038065763132E-32,0.,1.)) ;
#77195=DIRECTION('ref_axis',(1.,0.,4.93038065763132E-32)) ;
#77196=DIRECTION('',(0.,-1.,0.)) ;
#77197=DIRECTION('center_axis',(-4.93038065763132E-32,0.,1.)) ;
#77198=DIRECTION('ref_axis',(1.,0.,4.93038065763132E-32)) ;
#77199=DIRECTION('',(-1.,0.,-4.93038065763132E-32)) ;
#77200=DIRECTION('center_axis',(-8.13512808509168E-31,-3.26576826218999E-61,
1.)) ;
#77201=DIRECTION('ref_axis',(1.,4.27339674608664E-31,8.13512808509168E-31)) ;
#77202=DIRECTION('center_axis',(4.93038065763132E-32,0.,-1.)) ;
#77203=DIRECTION('ref_axis',(1.,0.,4.93038065763132E-32)) ;
#77204=DIRECTION('',(-4.27339674608664E-31,1.,-2.10694726592902E-62)) ;
#77205=DIRECTION('',(-1.,-4.27339674608664E-31,-8.13512808509168E-31)) ;
#77206=DIRECTION('',(-1.,-4.27339674608664E-31,-8.13512808509168E-31)) ;
#77207=DIRECTION('',(3.49247269410375E-15,-1.,1.72192198183147E-46)) ;
#77208=DIRECTION('',(-1.,4.27339674608665E-31,-4.93038065763132E-32)) ;
#77209=DIRECTION('',(-4.27339674608664E-31,1.,-2.10694726592902E-62)) ;
#77210=DIRECTION('center_axis',(4.93038065763132E-32,0.,-1.)) ;
#77211=DIRECTION('ref_axis',(1.,0.,4.93038065763132E-32)) ;
#77212=DIRECTION('',(-1.,4.27339674608665E-31,-4.93038065763132E-32)) ;
#77213=DIRECTION('',(-2.16840434497101E-16,1.,-1.06910588403688E-47)) ;
#77214=DIRECTION('',(1.,-4.27339674608665E-31,4.93038065763132E-32)) ;
#77215=DIRECTION('center_axis',(4.93038065763132E-32,0.,-1.)) ;
#77216=DIRECTION('ref_axis',(1.,0.,4.93038065763132E-32)) ;
#77217=DIRECTION('',(-1.73472347597681E-16,1.,-8.55284707229503E-48)) ;
#77218=DIRECTION('center_axis',(4.93038065763132E-32,0.,-1.)) ;
#77219=DIRECTION('ref_axis',(1.,0.,4.93038065763132E-32)) ;
#77220=DIRECTION('',(-1.,0.,-4.93038065763132E-32)) ;
#77221=DIRECTION('center_axis',(4.93038065763132E-32,0.,-1.)) ;
#77222=DIRECTION('ref_axis',(1.,0.,4.93038065763132E-32)) ;
#77223=DIRECTION('',(2.60208521396521E-16,-1.,1.28292706084425E-47)) ;
#77224=DIRECTION('center_axis',(4.93038065763132E-32,0.,-1.)) ;
#77225=DIRECTION('ref_axis',(1.,0.,4.93038065763132E-32)) ;
#77226=DIRECTION('',(1.,0.,4.93038065763132E-32)) ;
#77227=DIRECTION('center_axis',(4.93038065763132E-32,0.,-1.)) ;
#77228=DIRECTION('ref_axis',(1.,0.,4.93038065763132E-32)) ;
#77229=DIRECTION('',(0.,1.,0.)) ;
#77230=DIRECTION('center_axis',(4.93038065763132E-32,0.,-1.)) ;
#77231=DIRECTION('ref_axis',(1.,0.,4.93038065763132E-32)) ;
#77232=DIRECTION('',(-1.,0.,-4.93038065763132E-32)) ;
#77233=DIRECTION('center_axis',(4.93038065763132E-32,0.,-1.)) ;
#77234=DIRECTION('ref_axis',(1.,0.,4.93038065763132E-32)) ;
#77235=DIRECTION('',(3.46944695195361E-16,-1.,1.71056941445901E-47)) ;
#77236=DIRECTION('center_axis',(4.93038065763132E-32,0.,-1.)) ;
#77237=DIRECTION('ref_axis',(1.,0.,4.93038065763132E-32)) ;
#77238=DIRECTION('',(1.,0.,4.93038065763132E-32)) ;
#77239=DIRECTION('center_axis',(4.93038065763132E-32,0.,-1.)) ;
#77240=DIRECTION('ref_axis',(1.,0.,4.93038065763132E-32)) ;
#77241=DIRECTION('',(-6.93889390390723E-16,1.,-3.42113882891801E-47)) ;
#77242=DIRECTION('center_axis',(4.93038065763132E-32,0.,-1.)) ;
#77243=DIRECTION('ref_axis',(1.,0.,4.93038065763132E-32)) ;
#77244=DIRECTION('',(-1.,0.,-4.93038065763132E-32)) ;
#77245=DIRECTION('center_axis',(4.93038065763132E-32,0.,-1.)) ;
#77246=DIRECTION('ref_axis',(1.,0.,4.93038065763132E-32)) ;
#77247=DIRECTION('',(0.,-1.,0.)) ;
#77248=DIRECTION('center_axis',(4.93038065763132E-32,0.,-1.)) ;
#77249=DIRECTION('ref_axis',(1.,0.,4.93038065763132E-32)) ;
#77250=DIRECTION('',(1.,0.,4.93038065763132E-32)) ;
#77251=DIRECTION('center_axis',(4.93038065763132E-32,0.,-1.)) ;
#77252=DIRECTION('ref_axis',(1.,0.,4.93038065763132E-32)) ;
#77253=DIRECTION('',(0.,1.,0.)) ;
#77254=DIRECTION('center_axis',(4.93038065763132E-32,0.,-1.)) ;
#77255=DIRECTION('ref_axis',(1.,0.,4.93038065763132E-32)) ;
#77256=DIRECTION('',(-1.,0.,-4.93038065763132E-32)) ;
#77257=DIRECTION('center_axis',(4.93038065763132E-32,0.,-1.)) ;
#77258=DIRECTION('ref_axis',(1.,0.,4.93038065763132E-32)) ;
#77259=DIRECTION('',(0.,-1.,0.)) ;
#77260=DIRECTION('center_axis',(4.93038065763132E-32,0.,-1.)) ;
#77261=DIRECTION('ref_axis',(1.,0.,4.93038065763132E-32)) ;
#77262=DIRECTION('',(1.,0.,4.93038065763132E-32)) ;
#77263=DIRECTION('center_axis',(4.93038065763132E-32,0.,-1.)) ;
#77264=DIRECTION('ref_axis',(1.,0.,4.93038065763132E-32)) ;
#77265=DIRECTION('',(0.,1.,0.)) ;
#77266=DIRECTION('center_axis',(4.93038065763132E-32,0.,-1.)) ;
#77267=DIRECTION('ref_axis',(1.,0.,4.93038065763132E-32)) ;
#77268=DIRECTION('',(-1.,0.,-4.93038065763132E-32)) ;
#77269=DIRECTION('center_axis',(4.93038065763132E-32,0.,-1.)) ;
#77270=DIRECTION('ref_axis',(1.,0.,4.93038065763132E-32)) ;
#77271=DIRECTION('',(0.,-1.,0.)) ;
#77272=DIRECTION('center_axis',(4.93038065763132E-32,0.,-1.)) ;
#77273=DIRECTION('ref_axis',(1.,0.,4.93038065763132E-32)) ;
#77274=DIRECTION('',(1.,0.,4.93038065763132E-32)) ;
#77275=DIRECTION('center_axis',(4.93038065763132E-32,0.,-1.)) ;
#77276=DIRECTION('ref_axis',(1.,0.,4.93038065763132E-32)) ;
#77277=DIRECTION('',(-3.46944695195361E-16,1.,-1.71056941445901E-47)) ;
#77278=DIRECTION('center_axis',(4.93038065763132E-32,0.,-1.)) ;
#77279=DIRECTION('ref_axis',(1.,0.,4.93038065763132E-32)) ;
#77280=DIRECTION('',(-1.,0.,-4.93038065763132E-32)) ;
#77281=DIRECTION('center_axis',(4.93038065763132E-32,0.,-1.)) ;
#77282=DIRECTION('ref_axis',(1.,0.,4.93038065763132E-32)) ;
#77283=DIRECTION('',(0.,-1.,0.)) ;
#77284=DIRECTION('center_axis',(4.93038065763132E-32,0.,-1.)) ;
#77285=DIRECTION('ref_axis',(1.,0.,4.93038065763132E-32)) ;
#77286=DIRECTION('',(1.,0.,4.93038065763132E-32)) ;
#77287=DIRECTION('center_axis',(4.93038065763132E-32,0.,-1.)) ;
#77288=DIRECTION('ref_axis',(1.,0.,4.93038065763132E-32)) ;
#77289=DIRECTION('',(3.46944695195361E-16,-1.,1.71056941445901E-47)) ;
#77290=DIRECTION('center_axis',(4.93038065763132E-32,0.,-1.)) ;
#77291=DIRECTION('ref_axis',(1.,0.,4.93038065763132E-32)) ;
#77292=DIRECTION('',(1.,0.,4.93038065763132E-32)) ;
#77293=DIRECTION('center_axis',(4.93038065763132E-32,0.,-1.)) ;
#77294=DIRECTION('ref_axis',(1.,0.,4.93038065763132E-32)) ;
#77295=DIRECTION('',(0.,1.,0.)) ;
#77296=DIRECTION('center_axis',(4.93038065763132E-32,0.,-1.)) ;
#77297=DIRECTION('ref_axis',(1.,0.,4.93038065763132E-32)) ;
#77298=DIRECTION('',(-1.,0.,-4.93038065763132E-32)) ;
#77299=DIRECTION('center_axis',(-4.15069017696469E-34,1.,1.83697019872103E-16)) ;
#77300=DIRECTION('ref_axis',(4.60199940496102E-66,-1.83697019872103E-16,
1.)) ;
#77301=DIRECTION('center_axis',(-4.15069017696469E-34,1.,1.83697019872103E-16)) ;
#77302=DIRECTION('ref_axis',(1.85623770982812E-63,-1.83697019872103E-16,
1.)) ;
#77303=DIRECTION('',(6.04532600737121E-48,-1.83697019872103E-16,1.)) ;
#77304=DIRECTION('',(-1.,-3.29092219981587E-32,0.)) ;
#77305=DIRECTION('',(0.,2.16840434497101E-16,-1.)) ;
#77306=DIRECTION('',(-1.,-3.29092219981587E-32,0.)) ;
#77307=DIRECTION('',(6.04532600737121E-48,-1.83697019872103E-16,1.)) ;
#77308=DIRECTION('center_axis',(-4.15069017696469E-34,1.,1.83697019872103E-16)) ;
#77309=DIRECTION('ref_axis',(1.85623770982812E-63,-1.83697019872103E-16,
1.)) ;
#77310=DIRECTION('',(-1.,-4.15069017696469E-34,-7.62469415920825E-50)) ;
#77311=DIRECTION('',(6.04532600737121E-48,-1.83697019872103E-16,1.)) ;
#77312=DIRECTION('',(1.,4.15069017696469E-34,7.62469415920825E-50)) ;
#77313=DIRECTION('center_axis',(-4.15069017696469E-34,1.,1.83697019872103E-16)) ;
#77314=DIRECTION('ref_axis',(4.60199940496102E-66,-1.83697019872103E-16,
1.)) ;
#77315=DIRECTION('',(-1.,-3.29092219981587E-32,0.)) ;
#77316=DIRECTION('',(-6.04532600737121E-48,1.83697019872103E-16,-1.)) ;
#77317=DIRECTION('center_axis',(4.15069017696469E-34,-1.,-1.83697019872103E-16)) ;
#77318=DIRECTION('ref_axis',(-7.37593019805628E-50,-1.83697019872103E-16,
1.)) ;
#77319=DIRECTION('',(-1.,-4.15069017696469E-34,-7.62469415920825E-50)) ;
#77320=DIRECTION('',(-6.04532600737121E-48,1.83697019872103E-16,-1.)) ;
#77321=DIRECTION('',(1.,4.15069017696469E-34,7.62469415920825E-50)) ;
#77322=DIRECTION('center_axis',(4.15069017696469E-34,-1.,-1.83697019872103E-16)) ;
#77323=DIRECTION('ref_axis',(-7.37593019805628E-50,-1.83697019872103E-16,
1.)) ;
#77324=DIRECTION('',(-6.04532600737121E-48,1.83697019872103E-16,-1.)) ;
#77325=DIRECTION('',(-1.,-3.29092219981587E-32,0.)) ;
#77326=DIRECTION('',(0.,2.16840434497101E-16,-1.)) ;
#77327=DIRECTION('center_axis',(-1.,-3.29092219981587E-32,0.)) ;
#77328=DIRECTION('ref_axis',(0.,0.,1.)) ;
#77329=DIRECTION('',(-3.29092219981587E-32,-1.,0.)) ;
#77330=DIRECTION('',(6.04532600737121E-48,-1.83697019872103E-16,1.)) ;
#77331=DIRECTION('',(-3.29092219981587E-32,1.,1.83697019872103E-16)) ;
#77332=DIRECTION('',(-6.04532600737121E-48,1.83697019872103E-16,-1.)) ;
#77333=DIRECTION('center_axis',(-1.,-3.29092219981587E-32,0.)) ;
#77334=DIRECTION('ref_axis',(0.,0.,1.)) ;
#77335=DIRECTION('',(3.29092219981587E-32,-1.,-1.83697019872103E-16)) ;
#77336=DIRECTION('',(6.04532600737121E-48,-1.83697019872103E-16,1.)) ;
#77337=DIRECTION('',(3.29092219981587E-32,1.,0.)) ;
#77338=DIRECTION('',(-6.04532600737121E-48,1.83697019872103E-16,-1.)) ;
#77339=DIRECTION('center_axis',(-1.,-3.29092219981587E-32,0.)) ;
#77340=DIRECTION('ref_axis',(0.,0.,1.)) ;
#77341=DIRECTION('',(6.04532600737121E-48,-1.83697019872103E-16,1.)) ;
#77342=DIRECTION('',(-3.29092219981587E-32,1.,1.83697019872103E-16)) ;
#77343=DIRECTION('',(-6.04532600737121E-48,1.83697019872103E-16,-1.)) ;
#77344=DIRECTION('',(3.29092219981587E-32,-1.,-1.83697019872103E-16)) ;
#77345=DIRECTION('center_axis',(0.,1.83697019872103E-16,-1.)) ;
#77346=DIRECTION('ref_axis',(-4.15069017696464E-34,1.,1.83697019872103E-16)) ;
#77347=DIRECTION('',(-1.,-4.15069017696469E-34,-7.62469415920825E-50)) ;
#77348=DIRECTION('',(-3.29092219981587E-32,1.,1.83697019872103E-16)) ;
#77349=DIRECTION('',(1.,4.15069017696469E-34,7.62469415920825E-50)) ;
#77350=DIRECTION('',(3.29092219981587E-32,-1.,-1.83697019872103E-16)) ;
#77351=DIRECTION('center_axis',(0.,-1.83697019872103E-16,1.)) ;
#77352=DIRECTION('ref_axis',(4.15069017696464E-34,-1.,-1.83697019872103E-16)) ;
#77353=DIRECTION('',(1.,4.15069017696469E-34,7.62469415920825E-50)) ;
#77354=DIRECTION('',(-3.29092219981587E-32,1.,1.83697019872103E-16)) ;
#77355=DIRECTION('',(-1.,-4.15069017696469E-34,-7.62469415920825E-50)) ;
#77356=DIRECTION('',(3.29092219981587E-32,-1.,-1.83697019872103E-16)) ;
#77357=DIRECTION('center_axis',(-1.,-3.29092219981587E-32,0.)) ;
#77358=DIRECTION('ref_axis',(0.,0.,1.)) ;
#77359=DIRECTION('center_axis',(1.,3.29092219981587E-32,0.)) ;
#77360=DIRECTION('ref_axis',(3.29092219981587E-32,-1.,0.)) ;
#77361=DIRECTION('',(3.94430452610506E-31,-2.89120579329467E-16,-1.)) ;
#77362=DIRECTION('center_axis',(-1.,-3.29092219981587E-32,0.)) ;
#77363=DIRECTION('ref_axis',(3.29092219981587E-32,-1.,0.)) ;
#77364=DIRECTION('center_axis',(1.,3.29092219981587E-32,0.)) ;
#77365=DIRECTION('ref_axis',(0.,0.,-1.)) ;
#77366=DIRECTION('center_axis',(-1.,-3.29092219981587E-32,0.)) ;
#77367=DIRECTION('ref_axis',(-3.29092219981587E-32,1.,-6.24500451351651E-14)) ;
#77368=DIRECTION('',(-6.4275824215152E-33,1.,2.16840434497101E-16)) ;
#77369=DIRECTION('center_axis',(-1.,-3.29092219981587E-32,0.)) ;
#77370=DIRECTION('ref_axis',(0.,0.,1.)) ;
#77371=DIRECTION('',(3.94430452610506E-31,-2.89120579329467E-16,-1.)) ;
#77372=DIRECTION('center_axis',(1.,3.29092219981587E-32,0.)) ;
#77373=DIRECTION('ref_axis',(-3.29092219981587E-32,1.,0.)) ;
#77374=DIRECTION('center_axis',(1.,3.29092219981587E-32,0.)) ;
#77375=DIRECTION('ref_axis',(3.29092219981587E-32,-1.,0.)) ;
#77376=DIRECTION('center_axis',(1.,3.29092219981587E-32,0.)) ;
#77377=DIRECTION('ref_axis',(-3.29092219981587E-32,1.,0.)) ;
#77378=DIRECTION('center_axis',(-1.,-3.29092219981587E-32,0.)) ;
#77379=DIRECTION('ref_axis',(3.29092219981587E-32,-1.,0.)) ;
#77380=DIRECTION('center_axis',(-4.27339674608665E-31,-1.,-2.10694726592902E-62)) ;
#77381=DIRECTION('ref_axis',(4.93038065763132E-32,-3.97608260439759E-77,
-1.)) ;
#77382=DIRECTION('',(8.13512808509168E-31,9.86076131526265E-32,-1.)) ;
#77383=DIRECTION('',(1.,-4.27339674608665E-31,4.93038065763132E-32)) ;
#77384=DIRECTION('',(-7.39557098644695E-32,-9.86076131526265E-32,1.)) ;
#77385=DIRECTION('',(-1.,4.27339674608665E-31,-4.93038065763132E-32)) ;
#77386=DIRECTION('center_axis',(-1.,-4.27339674608664E-31,-4.93038065763132E-32)) ;
#77387=DIRECTION('ref_axis',(-4.93038065763132E-32,0.,1.)) ;
#77388=DIRECTION('',(4.27339674608664E-31,-1.,2.10694726592902E-62)) ;
#77389=DIRECTION('',(-8.13512808509168E-31,-9.86076131526265E-32,1.)) ;
#77390=DIRECTION('',(-4.27339674608664E-31,1.,-2.10694726592902E-62)) ;
#77391=DIRECTION('',(8.13512808509168E-31,9.86076131526265E-32,-1.)) ;
#77392=DIRECTION('center_axis',(-4.27339674608665E-31,-1.,-2.10694726592902E-62)) ;
#77393=DIRECTION('ref_axis',(4.93038065763132E-32,-3.97608260439759E-77,
-1.)) ;
#77394=DIRECTION('',(1.,-4.27339674608665E-31,4.93038065763132E-32)) ;
#77395=DIRECTION('',(-8.13512808509168E-31,-9.86076131526265E-32,1.)) ;
#77396=DIRECTION('',(-1.,4.27339674608665E-31,-4.93038065763132E-32)) ;
#77397=DIRECTION('',(7.39557098644699E-31,9.86076131526265E-32,-1.)) ;
#77398=DIRECTION('center_axis',(-1.,-2.168404344971E-16,-7.39557098644699E-31)) ;
#77399=DIRECTION('ref_axis',(2.168404344971E-16,-1.,-9.86076131526265E-32)) ;
#77400=DIRECTION('',(2.16840434497101E-16,-1.,1.06910588403688E-47)) ;
#77401=DIRECTION('',(-7.39557098644699E-31,-9.86076131526265E-32,1.)) ;
#77402=DIRECTION('',(-2.16840434497101E-16,1.,-1.06910588403688E-47)) ;
#77403=DIRECTION('',(7.39557098644699E-31,9.86076131526265E-32,-1.)) ;
#77404=DIRECTION('center_axis',(4.27339674608665E-31,1.,2.10694726592902E-62)) ;
#77405=DIRECTION('ref_axis',(-4.93038065763132E-32,3.97608260439759E-77,
1.)) ;
#77406=DIRECTION('',(-1.,4.27339674608665E-31,-4.93038065763132E-32)) ;
#77407=DIRECTION('',(-7.39557098644699E-31,-9.86076131526265E-32,1.)) ;
#77408=DIRECTION('',(1.,-4.27339674608665E-31,4.93038065763132E-32)) ;
#77409=DIRECTION('',(8.13512808509168E-31,9.86076131526265E-32,-1.)) ;
#77410=DIRECTION('center_axis',(-1.,-3.49247269410375E-15,-7.39557098644699E-32)) ;
#77411=DIRECTION('ref_axis',(3.49247269410375E-15,-1.,3.2391255885562E-16)) ;
#77412=DIRECTION('',(3.49247269410375E-15,-1.,1.72192198183147E-46)) ;
#77413=DIRECTION('',(7.39557098644695E-32,9.86076131526265E-32,-1.)) ;
#77414=DIRECTION('',(-3.49247269410375E-15,1.,-1.72192198183147E-46)) ;
#77415=DIRECTION('',(-1.08370143847609E-30,2.89120579329467E-16,1.)) ;
#77416=DIRECTION('center_axis',(-1.,-4.27339674608664E-31,-4.93038065763132E-32)) ;
#77417=DIRECTION('ref_axis',(-4.93038065763132E-32,0.,1.)) ;
#77418=DIRECTION('',(4.27339674608664E-31,-1.,2.10694726592902E-62)) ;
#77419=DIRECTION('',(-8.13512808509168E-31,-9.86076131526265E-32,1.)) ;
#77420=DIRECTION('',(-4.27339674608664E-31,1.,-2.10694726592902E-62)) ;
#77421=DIRECTION('center_axis',(4.7978874716823E-31,1.,-2.89120579329467E-16)) ;
#77422=DIRECTION('ref_axis',(-3.94430452610506E-31,2.89120579329467E-16,
1.)) ;
#77423=DIRECTION('',(1.08370143847609E-30,-2.89120579329467E-16,-1.)) ;
#77424=DIRECTION('center_axis',(-2.14282066180855E-30,7.70988211545247E-16,
-1.)) ;
#77425=DIRECTION('ref_axis',(0.,1.,7.70988211545247E-16)) ;
#77426=DIRECTION('',(3.65204942310907E-15,-1.,-7.70988211545247E-16)) ;
#77427=DIRECTION('',(-1.,-3.49148133884313E-15,-5.4907029126972E-31)) ;
#77428=DIRECTION('',(-3.65204942310907E-15,1.,7.70988211545247E-16)) ;
#77429=DIRECTION('',(1.,3.65204942310907E-15,6.72866391389159E-31)) ;
#77430=DIRECTION('center_axis',(-3.49148133884313E-15,1.,1.81408990951823E-16)) ;
#77431=DIRECTION('ref_axis',(-1.,-3.49148133884313E-15,0.)) ;
#77432=DIRECTION('',(-1.03517906367563E-32,-1.81408990951823E-16,1.)) ;
#77433=DIRECTION('',(-1.,-3.49148133884313E-15,-6.7286639138916E-31)) ;
#77434=DIRECTION('',(1.03517906367563E-32,1.81408990951823E-16,-1.)) ;
#77435=DIRECTION('',(1.,3.49148133884313E-15,5.4907029126972E-31)) ;
#77436=DIRECTION('center_axis',(6.7286639138916E-31,2.33447425067715E-45,
-1.)) ;
#77437=DIRECTION('ref_axis',(-1.,-8.92425379131539E-92,-6.7286639138916E-31)) ;
#77438=DIRECTION('',(-3.65204942310907E-15,1.,-1.22867065825113E-46)) ;
#77439=DIRECTION('',(-1.,-3.65204942310907E-15,-6.7286639138916E-31)) ;
#77440=DIRECTION('',(3.65204942310907E-15,-1.,1.22867065825113E-46)) ;
#77441=DIRECTION('',(1.,3.49148133884313E-15,6.7286639138916E-31)) ;
#77442=DIRECTION('center_axis',(3.65204942310907E-15,-1.,-2.47817639425257E-16)) ;
#77443=DIRECTION('ref_axis',(1.,3.65204942310907E-15,0.)) ;
#77444=DIRECTION('',(1.,3.65204942310907E-15,6.7286639138916E-31)) ;
#77445=DIRECTION('',(1.,3.65204942310907E-15,6.12323399573677E-17)) ;
#77446=DIRECTION('center_axis',(-3.65204942310907E-15,1.,2.47817639425258E-16)) ;
#77447=DIRECTION('ref_axis',(-1.,-3.65204942310907E-15,0.)) ;
#77448=DIRECTION('',(-1.,-3.65204942310907E-15,-6.72866391389159E-31)) ;
#77449=DIRECTION('',(1.,3.65204942310907E-15,6.12323399573677E-17)) ;
#77450=DIRECTION('center_axis',(0.,0.,-1.)) ;
#77451=DIRECTION('ref_axis',(-1.,0.,0.)) ;
#77452=DIRECTION('center_axis',(-1.03517906367563E-32,-1.81408990951823E-16,
1.)) ;
#77453=DIRECTION('ref_axis',(1.87790789395849E-48,-1.,-1.81408990951823E-16)) ;
#77454=DIRECTION('',(3.29092219981587E-32,1.,0.)) ;
#77455=DIRECTION('center_axis',(0.,0.,1.)) ;
#77456=DIRECTION('ref_axis',(1.,0.,0.)) ;
#77457=DIRECTION('center_axis',(0.,0.,1.)) ;
#77458=DIRECTION('ref_axis',(1.,0.,0.)) ;
#77459=DIRECTION('center_axis',(1.03517906367563E-32,1.81408990951823E-16,
-1.)) ;
#77460=DIRECTION('ref_axis',(1.87790789395849E-48,-1.,-1.81408990951823E-16)) ;
#77461=DIRECTION('center_axis',(0.,0.,-1.)) ;
#77462=DIRECTION('ref_axis',(-1.,0.,0.)) ;
#77463=DIRECTION('center_axis',(-1.03517906367563E-32,-1.81408990951823E-16,
1.)) ;
#77464=DIRECTION('ref_axis',(1.87790789395849E-48,-1.,-1.81408990951823E-16)) ;
#77465=DIRECTION('center_axis',(-1.03517906367563E-32,-1.81408990951823E-16,
1.)) ;
#77466=DIRECTION('ref_axis',(1.87790789395849E-48,-1.,-1.81408990951823E-16)) ;
#77467=DIRECTION('center_axis',(-1.,5.06932053596301E-14,2.51253409742467E-28)) ;
#77468=DIRECTION('ref_axis',(-5.06932053596301E-14,-1.,-9.19700082708845E-58)) ;
#77469=DIRECTION('',(4.42639173855935E-31,8.67361737988403E-16,-1.)) ;
#77470=DIRECTION('center_axis',(1.,-5.06932053596301E-14,-2.51253409742467E-28)) ;
#77471=DIRECTION('ref_axis',(-5.06932053596301E-14,-1.,-9.19700082708845E-58)) ;
#77472=DIRECTION('center_axis',(-1.,5.06932053596301E-14,2.51253409742467E-28)) ;
#77473=DIRECTION('ref_axis',(-5.06932053596301E-14,-1.,1.62924697510308E-57)) ;
#77474=DIRECTION('center_axis',(1.,0.,0.)) ;
#77475=DIRECTION('ref_axis',(0.,0.,-1.)) ;
#77476=DIRECTION('center_axis',(-1.,-3.29092219981587E-32,0.)) ;
#77477=DIRECTION('ref_axis',(3.29092219981587E-32,-1.,0.)) ;
#77478=DIRECTION('',(4.42639173855935E-31,8.67361737988403E-16,-1.)) ;
#77479=DIRECTION('center_axis',(-1.,0.,0.)) ;
#77480=DIRECTION('ref_axis',(0.,0.,1.)) ;
#77481=DIRECTION('center_axis',(-1.,-3.29092219981587E-32,0.)) ;
#77482=DIRECTION('ref_axis',(3.29092219981587E-32,-1.,0.)) ;
#77483=DIRECTION('center_axis',(1.,-5.06932053596301E-14,-2.51253409742467E-28)) ;
#77484=DIRECTION('ref_axis',(-5.06932053596301E-14,-1.,-2.48867833802847E-46)) ;
#77485=DIRECTION('center_axis',(-1.,-3.29092219981587E-32,0.)) ;
#77486=DIRECTION('ref_axis',(3.29092219981587E-32,-1.,0.)) ;
#77487=DIRECTION('center_axis',(-1.,5.06932053596301E-14,2.51253409742467E-28)) ;
#77488=DIRECTION('ref_axis',(-5.06932053596301E-14,-1.,1.69691425681666E-45)) ;
#77489=DIRECTION('center_axis',(-4.18667286880966E-31,-1.,-8.60595472516328E-62)) ;
#77490=DIRECTION('ref_axis',(2.05555938924125E-31,-1.72481183944414E-76,
-1.)) ;
#77491=DIRECTION('',(1.,-4.18667286880966E-31,4.7251522784556E-31)) ;
#77492=DIRECTION('',(-8.21355058201474E-31,3.43874493783169E-61,-1.)) ;
#77493=DIRECTION('',(-1.,4.18667286880966E-31,-4.7251522784556E-31)) ;
#77494=DIRECTION('',(5.76147612141447E-31,-2.41214157618207E-61,1.)) ;
#77495=DIRECTION('center_axis',(1.,2.168404344971E-16,-5.76147612141446E-31)) ;
#77496=DIRECTION('ref_axis',(-2.168404344971E-16,1.,-2.50236562288566E-63)) ;
#77497=DIRECTION('',(-2.16840434497101E-16,1.,7.02672800395669E-16)) ;
#77498=DIRECTION('',(-5.76147612141447E-31,2.33363072919793E-61,-1.)) ;
#77499=DIRECTION('',(2.16840434497101E-16,-1.,-7.02672800395669E-16)) ;
#77500=DIRECTION('',(5.76147612141447E-31,-2.33363072919793E-61,1.)) ;
#77501=DIRECTION('center_axis',(4.18667286880966E-31,1.,8.60595472516328E-62)) ;
#77502=DIRECTION('ref_axis',(-2.05555938924125E-31,1.72481183944414E-76,
1.)) ;
#77503=DIRECTION('',(-1.,4.18667286880966E-31,-4.7251522784556E-31)) ;
#77504=DIRECTION('',(-5.76147612141447E-31,2.41214157618207E-61,-1.)) ;
#77505=DIRECTION('',(1.,-4.18667286880966E-31,4.7251522784556E-31)) ;
#77506=DIRECTION('',(8.21355058201474E-31,-3.43874493783169E-61,1.)) ;
#77507=DIRECTION('center_axis',(1.,7.43707788821671E-32,2.05555938924125E-31)) ;
#77508=DIRECTION('ref_axis',(2.05555938924125E-31,0.,-1.)) ;
#77509=DIRECTION('',(-7.43707788821665E-32,1.,7.02672800395669E-16)) ;
#77510=DIRECTION('',(-8.21355058201474E-31,3.43874493783169E-61,-1.)) ;
#77511=DIRECTION('',(7.43707788821665E-32,-1.,-7.02672800395669E-16)) ;
#77512=DIRECTION('',(8.21355058201474E-31,-3.43874493783169E-61,1.)) ;
#77513=DIRECTION('center_axis',(-4.18667286880966E-31,-1.,-8.60595472516328E-62)) ;
#77514=DIRECTION('ref_axis',(2.05555938924125E-31,-1.72481183944414E-76,
-1.)) ;
#77515=DIRECTION('',(-1.,4.18667286880966E-31,-4.7251522784556E-31)) ;
#77516=DIRECTION('',(-8.21355058201474E-31,3.43874493783169E-61,-1.)) ;
#77517=DIRECTION('',(1.,-4.18667286880966E-31,4.7251522784556E-31)) ;
#77518=DIRECTION('',(-2.73644213932283E-30,1.14565880617704E-60,1.)) ;
#77519=DIRECTION('center_axis',(1.,3.49501116159781E-15,2.76935136132099E-30)) ;
#77520=DIRECTION('ref_axis',(-1.18287628881384E-30,1.13081975060932E-15,
-1.)) ;
#77521=DIRECTION('',(2.73644213932283E-30,-1.24460305557223E-60,-1.)) ;
#77522=DIRECTION('',(-3.49501116159781E-15,1.,7.02672800395669E-16)) ;
#77523=DIRECTION('',(2.94996816089511E-31,-8.67361737988403E-16,1.)) ;
#77524=DIRECTION('',(3.49501116159781E-15,-1.,-7.02672800395669E-16)) ;
#77525=DIRECTION('center_axis',(2.70755867152026E-31,1.,8.67361737988403E-16)) ;
#77526=DIRECTION('ref_axis',(-4.42639173855935E-31,-8.67361737988403E-16,
1.)) ;
#77527=DIRECTION('',(-2.94996816089511E-31,8.67361737988403E-16,-1.)) ;
#77528=DIRECTION('center_axis',(1.,7.43707788821671E-32,2.05555938924125E-31)) ;
#77529=DIRECTION('ref_axis',(2.05555938924125E-31,0.,-1.)) ;
#77530=DIRECTION('',(8.21355058201474E-31,-3.43874493783169E-61,1.)) ;
#77531=DIRECTION('',(-7.43707788821665E-32,1.,7.02672800395669E-16)) ;
#77532=DIRECTION('',(7.43707788821665E-32,-1.,-7.02672800395669E-16)) ;
#77533=DIRECTION('center_axis',(0.,-1.,0.)) ;
#77534=DIRECTION('ref_axis',(0.,0.,-1.)) ;
#77535=DIRECTION('',(1.,0.,4.93038065763132E-32)) ;
#77536=DIRECTION('',(0.,0.,-1.)) ;
#77537=DIRECTION('',(-1.,0.,-4.93038065763132E-32)) ;
#77538=DIRECTION('',(0.,0.,1.)) ;
#77539=DIRECTION('center_axis',(-1.,0.,0.)) ;
#77540=DIRECTION('ref_axis',(0.,0.,1.)) ;
#77541=DIRECTION('',(0.,-1.,0.)) ;
#77542=DIRECTION('',(0.,0.,-1.)) ;
#77543=DIRECTION('',(0.,1.,0.)) ;
#77544=DIRECTION('',(0.,0.,1.)) ;
#77545=DIRECTION('center_axis',(0.,1.,0.)) ;
#77546=DIRECTION('ref_axis',(0.,0.,1.)) ;
#77547=DIRECTION('',(1.,0.,4.93038065763132E-32)) ;
#77548=DIRECTION('',(0.,0.,1.)) ;
#77549=DIRECTION('',(-1.,0.,-4.93038065763132E-32)) ;
#77550=DIRECTION('',(0.,0.,-1.)) ;
#77551=DIRECTION('center_axis',(1.,0.,0.)) ;
#77552=DIRECTION('ref_axis',(0.,0.,-1.)) ;
#77553=DIRECTION('',(0.,1.,0.)) ;
#77554=DIRECTION('',(0.,0.,-1.)) ;
#77555=DIRECTION('',(0.,-1.,0.)) ;
#77556=DIRECTION('',(0.,0.,1.)) ;
#77557=DIRECTION('center_axis',(0.,-1.,0.)) ;
#77558=DIRECTION('ref_axis',(0.,0.,-1.)) ;
#77559=DIRECTION('',(1.,0.,4.93038065763132E-32)) ;
#77560=DIRECTION('',(0.,0.,-1.)) ;
#77561=DIRECTION('',(-1.,0.,-4.93038065763132E-32)) ;
#77562=DIRECTION('',(0.,0.,1.)) ;
#77563=DIRECTION('center_axis',(-1.,0.,0.)) ;
#77564=DIRECTION('ref_axis',(0.,0.,1.)) ;
#77565=DIRECTION('',(0.,-1.,0.)) ;
#77566=DIRECTION('',(0.,0.,-1.)) ;
#77567=DIRECTION('',(0.,1.,0.)) ;
#77568=DIRECTION('',(0.,0.,1.)) ;
#77569=DIRECTION('center_axis',(0.,1.,0.)) ;
#77570=DIRECTION('ref_axis',(0.,0.,1.)) ;
#77571=DIRECTION('',(1.,0.,4.93038065763132E-32)) ;
#77572=DIRECTION('',(0.,0.,1.)) ;
#77573=DIRECTION('',(-1.,0.,-4.93038065763132E-32)) ;
#77574=DIRECTION('',(0.,0.,-1.)) ;
#77575=DIRECTION('center_axis',(1.,0.,0.)) ;
#77576=DIRECTION('ref_axis',(0.,0.,-1.)) ;
#77577=DIRECTION('',(0.,1.,0.)) ;
#77578=DIRECTION('',(0.,0.,-1.)) ;
#77579=DIRECTION('',(0.,-1.,0.)) ;
#77580=DIRECTION('',(0.,0.,1.)) ;
#77581=DIRECTION('center_axis',(0.,-1.,0.)) ;
#77582=DIRECTION('ref_axis',(0.,0.,-1.)) ;
#77583=DIRECTION('',(1.,0.,4.93038065763132E-32)) ;
#77584=DIRECTION('',(0.,0.,-1.)) ;
#77585=DIRECTION('',(-1.,0.,-4.93038065763132E-32)) ;
#77586=DIRECTION('',(0.,0.,1.)) ;
#77587=DIRECTION('center_axis',(-1.,0.,0.)) ;
#77588=DIRECTION('ref_axis',(0.,0.,1.)) ;
#77589=DIRECTION('',(0.,-1.,0.)) ;
#77590=DIRECTION('',(0.,0.,-1.)) ;
#77591=DIRECTION('',(0.,1.,0.)) ;
#77592=DIRECTION('',(0.,0.,1.)) ;
#77593=DIRECTION('center_axis',(0.,1.,0.)) ;
#77594=DIRECTION('ref_axis',(0.,0.,1.)) ;
#77595=DIRECTION('',(1.,0.,4.93038065763132E-32)) ;
#77596=DIRECTION('',(0.,0.,1.)) ;
#77597=DIRECTION('',(-1.,0.,-4.93038065763132E-32)) ;
#77598=DIRECTION('',(0.,0.,-1.)) ;
#77599=DIRECTION('center_axis',(1.,6.93889390390723E-16,0.)) ;
#77600=DIRECTION('ref_axis',(-6.93889390390723E-16,1.,0.)) ;
#77601=DIRECTION('',(-6.93889390390723E-16,1.,-3.42113882891801E-47)) ;
#77602=DIRECTION('',(0.,0.,-1.)) ;
#77603=DIRECTION('',(6.93889390390723E-16,-1.,3.42113882891801E-47)) ;
#77604=DIRECTION('',(0.,0.,1.)) ;
#77605=DIRECTION('center_axis',(0.,-1.,0.)) ;
#77606=DIRECTION('ref_axis',(0.,0.,-1.)) ;
#77607=DIRECTION('',(1.,0.,4.93038065763132E-32)) ;
#77608=DIRECTION('',(0.,0.,-1.)) ;
#77609=DIRECTION('',(-1.,0.,-4.93038065763132E-32)) ;
#77610=DIRECTION('',(0.,0.,1.)) ;
#77611=DIRECTION('center_axis',(-1.,0.,0.)) ;
#77612=DIRECTION('ref_axis',(0.,0.,1.)) ;
#77613=DIRECTION('',(0.,-1.,0.)) ;
#77614=DIRECTION('',(0.,0.,-1.)) ;
#77615=DIRECTION('',(0.,1.,0.)) ;
#77616=DIRECTION('',(0.,0.,1.)) ;
#77617=DIRECTION('center_axis',(0.,1.,0.)) ;
#77618=DIRECTION('ref_axis',(0.,0.,1.)) ;
#77619=DIRECTION('',(1.,0.,4.93038065763132E-32)) ;
#77620=DIRECTION('',(0.,0.,1.)) ;
#77621=DIRECTION('',(-1.,0.,-4.93038065763132E-32)) ;
#77622=DIRECTION('',(0.,0.,-1.)) ;
#77623=DIRECTION('center_axis',(1.,3.46944695195361E-16,0.)) ;
#77624=DIRECTION('ref_axis',(-3.46944695195361E-16,1.,0.)) ;
#77625=DIRECTION('',(-3.46944695195361E-16,1.,-1.71056941445901E-47)) ;
#77626=DIRECTION('',(0.,0.,-1.)) ;
#77627=DIRECTION('',(3.46944695195361E-16,-1.,1.71056941445901E-47)) ;
#77628=DIRECTION('',(0.,0.,1.)) ;
#77629=DIRECTION('center_axis',(0.,-1.,0.)) ;
#77630=DIRECTION('ref_axis',(0.,0.,-1.)) ;
#77631=DIRECTION('',(1.,0.,4.93038065763132E-32)) ;
#77632=DIRECTION('',(0.,0.,-1.)) ;
#77633=DIRECTION('',(-1.,0.,-4.93038065763132E-32)) ;
#77634=DIRECTION('',(0.,0.,1.)) ;
#77635=DIRECTION('center_axis',(-1.,-3.46944695195361E-16,0.)) ;
#77636=DIRECTION('ref_axis',(3.46944695195361E-16,-1.,0.)) ;
#77637=DIRECTION('',(3.46944695195361E-16,-1.,1.71056941445901E-47)) ;
#77638=DIRECTION('',(0.,0.,-1.)) ;
#77639=DIRECTION('',(-3.46944695195361E-16,1.,-1.71056941445901E-47)) ;
#77640=DIRECTION('',(0.,0.,1.)) ;
#77641=DIRECTION('center_axis',(0.,1.,0.)) ;
#77642=DIRECTION('ref_axis',(0.,0.,1.)) ;
#77643=DIRECTION('',(1.,0.,4.93038065763132E-32)) ;
#77644=DIRECTION('',(0.,0.,1.)) ;
#77645=DIRECTION('',(-1.,0.,-4.93038065763132E-32)) ;
#77646=DIRECTION('',(0.,0.,-1.)) ;
#77647=DIRECTION('center_axis',(1.,0.,0.)) ;
#77648=DIRECTION('ref_axis',(0.,0.,-1.)) ;
#77649=DIRECTION('',(0.,1.,0.)) ;
#77650=DIRECTION('',(0.,0.,-1.)) ;
#77651=DIRECTION('',(0.,-1.,0.)) ;
#77652=DIRECTION('',(0.,0.,1.)) ;
#77653=DIRECTION('center_axis',(0.,-1.,0.)) ;
#77654=DIRECTION('ref_axis',(0.,0.,-1.)) ;
#77655=DIRECTION('',(-1.,0.,-4.93038065763132E-32)) ;
#77656=DIRECTION('',(0.,0.,1.)) ;
#77657=DIRECTION('',(1.,0.,4.93038065763132E-32)) ;
#77658=DIRECTION('',(0.,0.,-1.)) ;
#77659=DIRECTION('center_axis',(-1.,-3.46944695195361E-16,0.)) ;
#77660=DIRECTION('ref_axis',(3.46944695195361E-16,-1.,0.)) ;
#77661=DIRECTION('',(3.46944695195361E-16,-1.,1.71056941445901E-47)) ;
#77662=DIRECTION('',(0.,0.,-1.)) ;
#77663=DIRECTION('',(-3.46944695195361E-16,1.,-1.71056941445901E-47)) ;
#77664=DIRECTION('',(0.,0.,1.)) ;
#77665=DIRECTION('center_axis',(0.,1.,0.)) ;
#77666=DIRECTION('ref_axis',(0.,0.,1.)) ;
#77667=DIRECTION('',(-1.,0.,-4.93038065763132E-32)) ;
#77668=DIRECTION('',(0.,0.,-1.)) ;
#77669=DIRECTION('',(1.,0.,4.93038065763132E-32)) ;
#77670=DIRECTION('',(0.,0.,1.)) ;
#77671=DIRECTION('center_axis',(1.,0.,0.)) ;
#77672=DIRECTION('ref_axis',(0.,0.,-1.)) ;
#77673=DIRECTION('',(0.,1.,0.)) ;
#77674=DIRECTION('',(0.,0.,-1.)) ;
#77675=DIRECTION('',(0.,-1.,0.)) ;
#77676=DIRECTION('',(0.,0.,1.)) ;
#77677=DIRECTION('center_axis',(1.,1.73472347597681E-16,0.)) ;
#77678=DIRECTION('ref_axis',(-1.73472347597681E-16,1.,0.)) ;
#77679=DIRECTION('',(-1.73472347597681E-16,1.,-8.55284707229503E-48)) ;
#77680=DIRECTION('',(0.,0.,-1.)) ;
#77681=DIRECTION('',(1.73472347597681E-16,-1.,8.55284707229503E-48)) ;
#77682=DIRECTION('',(0.,0.,1.)) ;
#77683=DIRECTION('center_axis',(0.,-1.,0.)) ;
#77684=DIRECTION('ref_axis',(0.,0.,-1.)) ;
#77685=DIRECTION('',(1.,0.,4.93038065763132E-32)) ;
#77686=DIRECTION('',(0.,0.,-1.)) ;
#77687=DIRECTION('',(-1.,0.,-4.93038065763132E-32)) ;
#77688=DIRECTION('',(0.,0.,1.)) ;
#77689=DIRECTION('center_axis',(-1.,-2.60208521396521E-16,0.)) ;
#77690=DIRECTION('ref_axis',(2.60208521396521E-16,-1.,0.)) ;
#77691=DIRECTION('',(2.60208521396521E-16,-1.,1.28292706084425E-47)) ;
#77692=DIRECTION('',(0.,0.,-1.)) ;
#77693=DIRECTION('',(-2.60208521396521E-16,1.,-1.28292706084425E-47)) ;
#77694=DIRECTION('',(0.,0.,1.)) ;
#77695=DIRECTION('center_axis',(0.,1.,0.)) ;
#77696=DIRECTION('ref_axis',(0.,0.,1.)) ;
#77697=DIRECTION('',(1.,0.,4.93038065763132E-32)) ;
#77698=DIRECTION('',(0.,0.,1.)) ;
#77699=DIRECTION('',(-1.,0.,-4.93038065763132E-32)) ;
#77700=DIRECTION('',(0.,0.,-1.)) ;
#77701=DIRECTION('center_axis',(0.,-1.,-7.02672800395669E-16)) ;
#77702=DIRECTION('ref_axis',(0.,7.02672800395669E-16,-1.)) ;
#77703=DIRECTION('',(1.,-3.32023598379838E-46,4.72515227845561E-31)) ;
#77704=DIRECTION('',(4.72515227845561E-31,7.02672800395669E-16,-1.)) ;
#77705=DIRECTION('',(-1.,3.32023598379838E-46,-4.72515227845561E-31)) ;
#77706=DIRECTION('',(-4.72515227845561E-31,-7.02672800395669E-16,1.)) ;
#77707=DIRECTION('center_axis',(1.,-6.93889390390723E-16,-1.50619732651321E-32)) ;
#77708=DIRECTION('ref_axis',(6.93889390390723E-16,1.,-3.11691497273953E-64)) ;
#77709=DIRECTION('',(-6.93889390390723E-16,-1.,-7.02672800395669E-16)) ;
#77710=DIRECTION('',(-4.72515227845561E-31,-7.02672800395669E-16,1.)) ;
#77711=DIRECTION('',(6.93889390390723E-16,1.,7.02672800395669E-16)) ;
#77712=DIRECTION('',(4.72515227845561E-31,7.02672800395669E-16,-1.)) ;
#77713=DIRECTION('center_axis',(0.,1.,7.02672800395669E-16)) ;
#77714=DIRECTION('ref_axis',(0.,-7.02672800395669E-16,1.)) ;
#77715=DIRECTION('',(1.,-3.32023598379838E-46,4.72515227845561E-31)) ;
#77716=DIRECTION('',(-4.72515227845561E-31,-7.02672800395669E-16,1.)) ;
#77717=DIRECTION('',(-1.,3.32023598379838E-46,-4.72515227845561E-31)) ;
#77718=DIRECTION('',(4.72515227845561E-31,7.02672800395669E-16,-1.)) ;
#77719=DIRECTION('center_axis',(-1.,3.2787330340009E-46,-4.72515227845561E-31)) ;
#77720=DIRECTION('ref_axis',(-4.72515227845561E-31,0.,1.)) ;
#77721=DIRECTION('',(-4.15029497974802E-48,1.,7.02672800395669E-16)) ;
#77722=DIRECTION('',(-4.72515227845561E-31,-7.02672800395669E-16,1.)) ;
#77723=DIRECTION('',(4.15029497974802E-48,-1.,-7.02672800395669E-16)) ;
#77724=DIRECTION('',(4.72515227845561E-31,7.02672800395669E-16,-1.)) ;
#77725=DIRECTION('center_axis',(0.,1.,7.02672800395669E-16)) ;
#77726=DIRECTION('ref_axis',(0.,-7.02672800395669E-16,1.)) ;
#77727=DIRECTION('',(-1.,3.32023598379838E-46,-4.72515227845561E-31)) ;
#77728=DIRECTION('',(4.72515227845561E-31,7.02672800395669E-16,-1.)) ;
#77729=DIRECTION('',(1.,-3.32023598379838E-46,4.72515227845561E-31)) ;
#77730=DIRECTION('',(-4.72515227845561E-31,-7.02672800395669E-16,1.)) ;
#77731=DIRECTION('center_axis',(1.,-3.12260288952466E-46,4.72515227845561E-31)) ;
#77732=DIRECTION('ref_axis',(4.72515227845561E-31,0.,-1.)) ;
#77733=DIRECTION('',(1.97633094273713E-47,-1.,-7.02672800395669E-16)) ;
#77734=DIRECTION('',(-4.72515227845561E-31,-7.02672800395669E-16,1.)) ;
#77735=DIRECTION('',(-1.97633094273713E-47,1.,7.02672800395669E-16)) ;
#77736=DIRECTION('',(4.72515227845561E-31,7.02672800395669E-16,-1.)) ;
#77737=DIRECTION('center_axis',(0.,-1.,-7.02672800395669E-16)) ;
#77738=DIRECTION('ref_axis',(0.,7.02672800395669E-16,-1.)) ;
#77739=DIRECTION('',(-1.,3.32023598379838E-46,-4.72515227845561E-31)) ;
#77740=DIRECTION('',(-4.72515227845561E-31,-7.02672800395669E-16,1.)) ;
#77741=DIRECTION('',(1.,-3.32023598379838E-46,4.72515227845561E-31)) ;
#77742=DIRECTION('',(4.72515227845561E-31,7.02672800395669E-16,-1.)) ;
#77743=DIRECTION('center_axis',(-1.,3.12260288952466E-46,-4.72515227845561E-31)) ;
#77744=DIRECTION('ref_axis',(-4.72515227845561E-31,0.,1.)) ;
#77745=DIRECTION('',(-1.97633094273713E-47,1.,7.02672800395669E-16)) ;
#77746=DIRECTION('',(-4.72515227845561E-31,-7.02672800395669E-16,1.)) ;
#77747=DIRECTION('',(1.97633094273713E-47,-1.,-7.02672800395669E-16)) ;
#77748=DIRECTION('',(4.72515227845561E-31,7.02672800395669E-16,-1.)) ;
#77749=DIRECTION('center_axis',(0.,-1.,-7.02672800395669E-16)) ;
#77750=DIRECTION('ref_axis',(0.,7.02672800395669E-16,-1.)) ;
#77751=DIRECTION('',(1.,-3.32023598379838E-46,4.72515227845561E-31)) ;
#77752=DIRECTION('',(4.72515227845561E-31,7.02672800395669E-16,-1.)) ;
#77753=DIRECTION('',(-1.,3.32023598379838E-46,-4.72515227845561E-31)) ;
#77754=DIRECTION('',(-4.72515227845561E-31,-7.02672800395669E-16,1.)) ;
#77755=DIRECTION('center_axis',(1.,-3.46944695195361E-16,2.28726627290214E-31)) ;
#77756=DIRECTION('ref_axis',(3.46944695195361E-16,1.,1.5484195688691E-63)) ;
#77757=DIRECTION('',(-3.46944695195361E-16,-1.,-7.02672800395669E-16)) ;
#77758=DIRECTION('',(-4.72515227845561E-31,-7.02672800395669E-16,1.)) ;
#77759=DIRECTION('',(3.46944695195361E-16,1.,7.02672800395669E-16)) ;
#77760=DIRECTION('',(4.72515227845561E-31,7.02672800395669E-16,-1.)) ;
#77761=DIRECTION('center_axis',(0.,1.,7.02672800395669E-16)) ;
#77762=DIRECTION('ref_axis',(0.,-7.02672800395669E-16,1.)) ;
#77763=DIRECTION('',(1.,-3.32023598379838E-46,4.72515227845561E-31)) ;
#77764=DIRECTION('',(-4.72515227845561E-31,-7.02672800395669E-16,1.)) ;
#77765=DIRECTION('',(-1.,3.32023598379838E-46,-4.72515227845561E-31)) ;
#77766=DIRECTION('',(4.72515227845561E-31,7.02672800395669E-16,-1.)) ;
#77767=DIRECTION('center_axis',(-1.,1.73472347597681E-16,-3.50620927567887E-31)) ;
#77768=DIRECTION('ref_axis',(-1.73472347597681E-16,-1.,-1.0604312475688E-64)) ;
#77769=DIRECTION('',(1.73472347597681E-16,1.,7.02672800395669E-16)) ;
#77770=DIRECTION('',(-4.72515227845561E-31,-7.02672800395669E-16,1.)) ;
#77771=DIRECTION('',(-1.73472347597681E-16,-1.,-7.02672800395669E-16)) ;
#77772=DIRECTION('',(4.72515227845561E-31,7.02672800395669E-16,-1.)) ;
#77773=DIRECTION('center_axis',(-1.,8.67361737988404E-17,-4.11568077706724E-31)) ;
#77774=DIRECTION('ref_axis',(-8.67361737988404E-17,-1.,1.5859151899932E-63)) ;
#77775=DIRECTION('',(8.67361737988404E-17,1.,7.02672800395669E-16)) ;
#77776=DIRECTION('',(-4.72515227845561E-31,-7.02672800395669E-16,1.)) ;
#77777=DIRECTION('',(-8.67361737988404E-17,-1.,-7.02672800395669E-16)) ;
#77778=DIRECTION('',(4.72515227845561E-31,7.02672800395669E-16,-1.)) ;
#77779=DIRECTION('center_axis',(0.,-1.,-7.02672800395669E-16)) ;
#77780=DIRECTION('ref_axis',(0.,7.02672800395669E-16,-1.)) ;
#77781=DIRECTION('',(-1.,3.32023598379838E-46,-4.72515227845561E-31)) ;
#77782=DIRECTION('',(-4.72515227845561E-31,-7.02672800395669E-16,1.)) ;
#77783=DIRECTION('',(1.,-3.32023598379838E-46,4.72515227845561E-31)) ;
#77784=DIRECTION('',(4.72515227845561E-31,7.02672800395669E-16,-1.)) ;
#77785=DIRECTION('center_axis',(1.,-1.73472347597681E-16,3.50620927567887E-31)) ;
#77786=DIRECTION('ref_axis',(1.73472347597681E-16,1.,1.0604312475688E-64)) ;
#77787=DIRECTION('',(-1.73472347597681E-16,-1.,-7.02672800395669E-16)) ;
#77788=DIRECTION('',(-4.72515227845561E-31,-7.02672800395669E-16,1.)) ;
#77789=DIRECTION('',(1.73472347597681E-16,1.,7.02672800395669E-16)) ;
#77790=DIRECTION('',(4.72515227845561E-31,7.02672800395669E-16,-1.)) ;
#77791=DIRECTION('center_axis',(0.,1.,7.02672800395669E-16)) ;
#77792=DIRECTION('ref_axis',(0.,-7.02672800395669E-16,1.)) ;
#77793=DIRECTION('',(-1.,3.32023598379838E-46,-4.72515227845561E-31)) ;
#77794=DIRECTION('',(4.72515227845561E-31,7.02672800395669E-16,-1.)) ;
#77795=DIRECTION('',(1.,-3.32023598379838E-46,4.72515227845561E-31)) ;
#77796=DIRECTION('',(-4.72515227845561E-31,-7.02672800395669E-16,1.)) ;
#77797=DIRECTION('center_axis',(6.7286639138916E-31,2.80136910081258E-45,
-1.)) ;
#77798=DIRECTION('ref_axis',(-1.,1.16708558817391E-91,-6.7286639138916E-31)) ;
#77799=DIRECTION('',(-1.,-3.65204942310907E-15,-6.7286639138916E-31)) ;
#77800=DIRECTION('',(3.65204942310907E-15,-1.,-3.44027784310316E-46)) ;
#77801=DIRECTION('',(1.,3.65204942310907E-15,6.7286639138916E-31)) ;
#77802=DIRECTION('',(-3.65204942310907E-15,1.,3.44027784310316E-46)) ;
#77803=DIRECTION('center_axis',(3.65204942310907E-15,-1.,0.)) ;
#77804=DIRECTION('ref_axis',(1.,3.65204942310907E-15,0.)) ;
#77805=DIRECTION('',(6.7286639138916E-31,2.45734131650226E-45,-1.)) ;
#77806=DIRECTION('',(-1.,-3.65204942310907E-15,-6.7286639138916E-31)) ;
#77807=DIRECTION('',(-6.7286639138916E-31,-2.45734131650226E-45,1.)) ;
#77808=DIRECTION('',(1.,3.65204942310907E-15,6.7286639138916E-31)) ;
#77809=DIRECTION('center_axis',(-6.7286639138916E-31,-2.80136910081258E-45,
1.)) ;
#77810=DIRECTION('ref_axis',(1.,-1.16708558817391E-91,6.7286639138916E-31)) ;
#77811=DIRECTION('',(-1.,-3.65204942310907E-15,-6.7286639138916E-31)) ;
#77812=DIRECTION('',(-3.65204942310907E-15,1.,3.44027784310316E-46)) ;
#77813=DIRECTION('',(1.,3.65204942310907E-15,6.7286639138916E-31)) ;
#77814=DIRECTION('',(3.65204942310907E-15,-1.,-3.44027784310316E-46)) ;
#77815=DIRECTION('center_axis',(-3.65204942310907E-15,1.,0.)) ;
#77816=DIRECTION('ref_axis',(-1.,-3.65204942310907E-15,0.)) ;
#77817=DIRECTION('',(6.7286639138916E-31,2.45734131650226E-45,-1.)) ;
#77818=DIRECTION('',(1.,3.65204942310907E-15,6.7286639138916E-31)) ;
#77819=DIRECTION('',(-6.7286639138916E-31,-2.45734131650226E-45,1.)) ;
#77820=DIRECTION('',(-1.,-3.65204942310907E-15,-6.7286639138916E-31)) ;
#77821=DIRECTION('center_axis',(3.49501116159781E-15,-1.,-7.02672800395669E-16)) ;
#77822=DIRECTION('ref_axis',(1.,3.49501116159781E-15,-4.6242849322719E-44)) ;
#77823=DIRECTION('center_axis',(0.,-1.,0.)) ;
#77824=DIRECTION('ref_axis',(0.,0.,-1.)) ;
#77825=DIRECTION('center_axis',(-2.42270293935615E-13,0.707106781186481,
0.707106781186614)) ;
#77826=DIRECTION('ref_axis',(5.46329954747089E-13,-0.707106781186614,0.707106781186481)) ;
#77827=DIRECTION('center_axis',(2.94996816089511E-31,-8.67361737988403E-16,
1.)) ;
#77828=DIRECTION('ref_axis',(-2.55868951104443E-46,-1.,-8.67361737988403E-16)) ;
#77829=DIRECTION('center_axis',(-1.88071505525119E-14,-0.707106781186579,
0.707106781186516)) ;
#77830=DIRECTION('ref_axis',(-5.62922653036698E-12,-0.707106781186516,-0.707106781186579)) ;
#77831=DIRECTION('center_axis',(0.,1.,0.)) ;
#77832=DIRECTION('ref_axis',(1.,0.,0.)) ;
#77833=DIRECTION('center_axis',(-1.,0.,0.)) ;
#77834=DIRECTION('ref_axis',(0.,0.,-1.)) ;
#77835=DIRECTION('center_axis',(0.,0.,1.)) ;
#77836=DIRECTION('ref_axis',(-1.,0.,0.)) ;
#77837=DIRECTION('center_axis',(-3.49501116159781E-15,1.,7.02672800395669E-16)) ;
#77838=DIRECTION('ref_axis',(-1.,-3.49501116159781E-15,-2.45584928033405E-30)) ;
#77839=DIRECTION('center_axis',(0.,-1.,0.)) ;
#77840=DIRECTION('ref_axis',(0.,0.,-1.)) ;
#77841=DIRECTION('center_axis',(-2.73644213932283E-30,1.14565880617704E-60,
1.)) ;
#77842=DIRECTION('ref_axis',(1.,3.13502903450913E-90,2.73644213932283E-30)) ;
#77843=DIRECTION('center_axis',(0.,0.,1.)) ;
#77844=DIRECTION('ref_axis',(1.,0.,0.)) ;
#77845=DIRECTION('center_axis',(-1.,4.18667286880966E-31,-4.7251522784556E-31)) ;
#77846=DIRECTION('ref_axis',(-4.7251522784556E-31,1.97826668452042E-61,
1.)) ;
#77847=DIRECTION('center_axis',(-1.,0.,0.)) ;
#77848=DIRECTION('ref_axis',(0.,0.,1.)) ;
#77849=DIRECTION('center_axis',(0.,1.,0.)) ;
#77850=DIRECTION('ref_axis',(1.,0.,0.)) ;
#77851=DIRECTION('center_axis',(-1.,0.,0.)) ;
#77852=DIRECTION('ref_axis',(0.,0.,-1.)) ;
#77853=DIRECTION('center_axis',(0.,1.,0.)) ;
#77854=DIRECTION('ref_axis',(1.,0.,0.)) ;
#77855=DIRECTION('center_axis',(0.,1.,0.)) ;
#77856=DIRECTION('ref_axis',(0.,0.,-1.)) ;
#77857=DIRECTION('center_axis',(0.,0.,1.)) ;
#77858=DIRECTION('ref_axis',(-1.,0.,0.)) ;
#77859=DIRECTION('center_axis',(1.,-4.18667286880966E-31,4.7251522784556E-31)) ;
#77860=DIRECTION('ref_axis',(4.7251522784556E-31,-1.97826668452042E-61,
-1.)) ;
#77861=DIRECTION('center_axis',(-1.,0.,-1.75279351218493E-14)) ;
#77862=DIRECTION('ref_axis',(-1.75279351218493E-14,0.,1.)) ;
#77863=DIRECTION('center_axis',(-8.21355058201474E-31,3.43874493783169E-61,
-1.)) ;
#77864=DIRECTION('ref_axis',(-1.,-2.82443054855277E-91,8.21355058201474E-31)) ;
#77865=DIRECTION('center_axis',(0.,0.,1.)) ;
#77866=DIRECTION('ref_axis',(1.,0.,0.)) ;
#77867=DIRECTION('center_axis',(-7.43707788821665E-32,1.,7.02672800395669E-16)) ;
#77868=DIRECTION('ref_axis',(5.2258323464739E-47,-7.02672800395669E-16,
1.)) ;
#77869=DIRECTION('center_axis',(0.,1.,0.)) ;
#77870=DIRECTION('ref_axis',(0.,0.,1.)) ;
#77871=DIRECTION('center_axis',(0.,1.,0.)) ;
#77872=DIRECTION('ref_axis',(1.,0.,0.)) ;
#77873=DIRECTION('center_axis',(0.,1.,0.)) ;
#77874=DIRECTION('ref_axis',(0.,0.,-1.)) ;
#77875=DIRECTION('center_axis',(4.72515227845561E-31,7.02672800395669E-16,
-1.)) ;
#77876=DIRECTION('ref_axis',(0.,1.,0.)) ;
#77877=DIRECTION('center_axis',(4.72515227845561E-31,7.02672800395669E-16,
-1.)) ;
#77878=DIRECTION('ref_axis',(-3.32023598379838E-46,1.,7.02672800395669E-16)) ;
#77879=DIRECTION('center_axis',(-1.,0.,0.)) ;
#77880=DIRECTION('ref_axis',(0.,0.,-1.)) ;
#77881=DIRECTION('center_axis',(7.43707788821665E-32,-1.,-7.02672800395669E-16)) ;
#77882=DIRECTION('ref_axis',(8.2037222863304E-61,7.02672800395669E-16,-1.)) ;
#77883=DIRECTION('center_axis',(0.,1.,0.)) ;
#77884=DIRECTION('ref_axis',(0.,0.,1.)) ;
#77885=DIRECTION('center_axis',(8.21355058201474E-31,-3.43874493783169E-61,
1.)) ;
#77886=DIRECTION('ref_axis',(1.,2.82443054855277E-91,-8.21355058201474E-31)) ;
#77887=DIRECTION('center_axis',(4.72515227845561E-31,7.02672800395669E-16,
-1.)) ;
#77888=DIRECTION('ref_axis',(-3.32023598379838E-46,1.,7.02672800395669E-16)) ;
#77889=DIRECTION('center_axis',(-1.,4.18667286880966E-31,-4.7251522784556E-31)) ;
#77890=DIRECTION('ref_axis',(-4.7251522784556E-31,1.97826668452042E-61,
1.)) ;
#77891=DIRECTION('center_axis',(-1.,0.,0.)) ;
#77892=DIRECTION('ref_axis',(0.,0.,1.)) ;
#77893=DIRECTION('center_axis',(4.72515227845561E-31,7.02672800395669E-16,
-1.)) ;
#77894=DIRECTION('ref_axis',(0.,1.,0.)) ;
#77895=DIRECTION('center_axis',(-1.,0.,0.)) ;
#77896=DIRECTION('ref_axis',(0.,0.,-1.)) ;
#77897=DIRECTION('center_axis',(0.,1.,0.)) ;
#77898=DIRECTION('ref_axis',(1.,0.,0.)) ;
#77899=DIRECTION('center_axis',(0.,1.,0.)) ;
#77900=DIRECTION('ref_axis',(0.,0.,-1.)) ;
#77901=DIRECTION('center_axis',(4.62592926927149E-14,0.,1.)) ;
#77902=DIRECTION('ref_axis',(-1.,0.,4.62592926927149E-14)) ;
#77903=DIRECTION('center_axis',(1.,-4.18667286880966E-31,4.7251522784556E-31)) ;
#77904=DIRECTION('ref_axis',(4.7251522784556E-31,-1.97826668452042E-61,
-1.)) ;
#77905=DIRECTION('center_axis',(-1.,0.,-1.01192202765316E-14)) ;
#77906=DIRECTION('ref_axis',(-1.01192202765316E-14,0.,1.)) ;
#77907=DIRECTION('center_axis',(-5.76147612141446E-31,2.41214157618207E-61,
-1.)) ;
#77908=DIRECTION('ref_axis',(-1.,-1.3897496092644E-91,5.76147612141446E-31)) ;
#77909=DIRECTION('center_axis',(0.,-4.62592926927149E-14,1.)) ;
#77910=DIRECTION('ref_axis',(0.,-1.,-4.62592926927149E-14)) ;
#77911=DIRECTION('center_axis',(-2.16840434497101E-16,1.,7.02672800395669E-16)) ;
#77912=DIRECTION('ref_axis',(1.52367875347092E-31,-7.02672800395669E-16,
1.)) ;
#77913=DIRECTION('center_axis',(0.,1.,0.)) ;
#77914=DIRECTION('ref_axis',(0.,0.,1.)) ;
#77915=DIRECTION('center_axis',(0.,1.,0.)) ;
#77916=DIRECTION('ref_axis',(1.,0.,0.)) ;
#77917=DIRECTION('center_axis',(0.,1.,0.)) ;
#77918=DIRECTION('ref_axis',(0.,0.,-1.)) ;
#77919=DIRECTION('center_axis',(0.,1.,0.)) ;
#77920=DIRECTION('ref_axis',(1.,0.,0.)) ;
#77921=DIRECTION('center_axis',(1.,0.,0.)) ;
#77922=DIRECTION('ref_axis',(0.,0.,1.)) ;
#77923=DIRECTION('center_axis',(0.,4.62592926927149E-14,1.)) ;
#77924=DIRECTION('ref_axis',(0.,1.,-4.62592926927149E-14)) ;
#77925=DIRECTION('center_axis',(2.16840434497101E-16,-1.,-7.02672800395669E-16)) ;
#77926=DIRECTION('ref_axis',(3.47941294872983E-45,7.02672800395669E-16,
-1.)) ;
#77927=DIRECTION('center_axis',(0.,1.,0.)) ;
#77928=DIRECTION('ref_axis',(0.,0.,1.)) ;
#77929=DIRECTION('center_axis',(-5.76147612141446E-31,2.41214157618207E-61,
-1.)) ;
#77930=DIRECTION('ref_axis',(-1.,-1.3897496092644E-91,5.76147612141446E-31)) ;
#77931=DIRECTION('center_axis',(0.,0.,1.)) ;
#77932=DIRECTION('ref_axis',(1.,0.,0.)) ;
#77933=DIRECTION('center_axis',(1.,-4.18667286880966E-31,4.7251522784556E-31)) ;
#77934=DIRECTION('ref_axis',(4.7251522784556E-31,-1.97826668452042E-61,
-1.)) ;
#77935=DIRECTION('center_axis',(1.,0.,0.)) ;
#77936=DIRECTION('ref_axis',(0.,0.,-1.)) ;
#77937=DIRECTION('center_axis',(-3.49247269410375E-15,1.,-1.72192198183147E-46)) ;
#77938=DIRECTION('ref_axis',(-1.,-3.49247269410375E-15,6.01376550292341E-61)) ;
#77939=DIRECTION('center_axis',(-2.16795153641756E-13,0.707106781186498,
-0.707106781186597)) ;
#77940=DIRECTION('ref_axis',(8.90474808132134E-13,0.707106781186597,0.707106781186498)) ;
#77941=DIRECTION('center_axis',(0.,-1.,0.)) ;
#77942=DIRECTION('ref_axis',(0.,0.,-1.)) ;
#77943=DIRECTION('center_axis',(0.,1.,0.)) ;
#77944=DIRECTION('ref_axis',(1.,0.,0.)) ;
#77945=DIRECTION('center_axis',(1.,-1.01192202765314E-14,0.)) ;
#77946=DIRECTION('ref_axis',(-1.01192202765314E-14,-1.,0.)) ;
#77947=DIRECTION('center_axis',(4.72515227845561E-31,7.02672800395669E-16,
-1.)) ;
#77948=DIRECTION('ref_axis',(0.,1.,0.)) ;
#77949=DIRECTION('center_axis',(4.72515227845561E-31,7.02672800395669E-16,
-1.)) ;
#77950=DIRECTION('ref_axis',(-3.32023598379838E-46,1.,7.02672800395669E-16)) ;
#77951=DIRECTION('center_axis',(0.,1.,0.)) ;
#77952=DIRECTION('ref_axis',(0.,0.,-1.)) ;
#77953=DIRECTION('center_axis',(0.,1.,0.)) ;
#77954=DIRECTION('ref_axis',(1.,0.,0.)) ;
#77955=DIRECTION('center_axis',(0.,0.,-1.)) ;
#77956=DIRECTION('ref_axis',(1.,0.,0.)) ;
#77957=DIRECTION('center_axis',(-1.,0.,0.)) ;
#77958=DIRECTION('ref_axis',(0.,0.,-1.)) ;
#77959=DIRECTION('center_axis',(1.08370143847609E-30,-2.89120579329467E-16,
-1.)) ;
#77960=DIRECTION('ref_axis',(3.13320387712385E-46,1.,-2.89120579329467E-16)) ;
#77961=DIRECTION('center_axis',(-5.66779128014443E-14,-0.707106781186571,
-0.707106781186524)) ;
#77962=DIRECTION('ref_axis',(2.75100792174159E-12,0.707106781186524,-0.707106781186571)) ;
#77963=DIRECTION('center_axis',(-1.,4.18667286880966E-31,-4.7251522784556E-31)) ;
#77964=DIRECTION('ref_axis',(-4.7251522784556E-31,1.97826668452042E-61,
1.)) ;
#77965=DIRECTION('center_axis',(1.,0.,0.)) ;
#77966=DIRECTION('ref_axis',(0.,0.,-1.)) ;
#77967=DIRECTION('center_axis',(8.21355058201474E-31,-3.43874493783169E-61,
1.)) ;
#77968=DIRECTION('ref_axis',(1.,2.82443054855277E-91,-8.21355058201474E-31)) ;
#77969=DIRECTION('center_axis',(4.72515227845561E-31,7.02672800395669E-16,
-1.)) ;
#77970=DIRECTION('ref_axis',(-3.32023598379838E-46,1.,7.02672800395669E-16)) ;
#77971=DIRECTION('center_axis',(-7.43707788821665E-32,1.,7.02672800395669E-16)) ;
#77972=DIRECTION('ref_axis',(5.2258323464739E-47,-7.02672800395669E-16,
1.)) ;
#77973=DIRECTION('center_axis',(4.91504984860095E-14,1.,0.)) ;
#77974=DIRECTION('ref_axis',(-1.,4.91504984860095E-14,0.)) ;
#77975=DIRECTION('center_axis',(-1.,4.27339674608665E-31,-4.93038065763132E-32)) ;
#77976=DIRECTION('ref_axis',(-4.27339674608665E-31,-1.,-2.10694726592902E-62)) ;
#77977=DIRECTION('center_axis',(-1.,0.,0.)) ;
#77978=DIRECTION('ref_axis',(0.,0.,1.)) ;
#77979=DIRECTION('center_axis',(7.39557098644695E-32,9.86076131526265E-32,
-1.)) ;
#77980=DIRECTION('ref_axis',(-7.29259602874349E-63,1.,9.86076131526265E-32)) ;
#77981=DIRECTION('center_axis',(0.,0.,-1.)) ;
#77982=DIRECTION('ref_axis',(-1.,0.,0.)) ;
#77983=DIRECTION('center_axis',(3.49247269410375E-15,-1.,1.72192198183147E-46)) ;
#77984=DIRECTION('ref_axis',(1.,3.49247269410375E-15,-6.01376550292341E-61)) ;
#77985=DIRECTION('center_axis',(0.,-1.,0.)) ;
#77986=DIRECTION('ref_axis',(0.,0.,-1.)) ;
#77987=DIRECTION('center_axis',(4.72515227845561E-31,7.02672800395669E-16,
-1.)) ;
#77988=DIRECTION('ref_axis',(0.,1.,0.)) ;
#77989=DIRECTION('center_axis',(0.,1.,0.)) ;
#77990=DIRECTION('ref_axis',(0.,0.,-1.)) ;
#77991=DIRECTION('center_axis',(-1.,5.06932053596301E-14,2.51253409742467E-28)) ;
#77992=DIRECTION('ref_axis',(-5.06896112386E-14,-1.,0.)) ;
#77993=DIRECTION('center_axis',(0.,0.,1.)) ;
#77994=DIRECTION('ref_axis',(1.,0.,0.)) ;
#77995=DIRECTION('center_axis',(0.,1.,0.)) ;
#77996=DIRECTION('ref_axis',(1.,0.,0.)) ;
#77997=DIRECTION('center_axis',(0.,0.,-1.)) ;
#77998=DIRECTION('ref_axis',(1.,0.,0.)) ;
#77999=DIRECTION('center_axis',(0.,1.,0.)) ;
#78000=DIRECTION('ref_axis',(0.,0.,-1.)) ;
#78001=DIRECTION('center_axis',(0.,1.,0.)) ;
#78002=DIRECTION('ref_axis',(1.,0.,0.)) ;
#78003=DIRECTION('center_axis',(-1.,0.,0.)) ;
#78004=DIRECTION('ref_axis',(0.,0.,-1.)) ;
#78005=DIRECTION('center_axis',(7.43707788821665E-32,-1.,-7.02672800395669E-16)) ;
#78006=DIRECTION('ref_axis',(8.2037222863304E-61,7.02672800395669E-16,-1.)) ;
#78007=DIRECTION('center_axis',(0.,1.,4.7704895589363E-14)) ;
#78008=DIRECTION('ref_axis',(0.,-4.7704895589363E-14,1.)) ;
#78009=DIRECTION('center_axis',(-6.04532600737121E-48,1.83697019872103E-16,
-1.)) ;
#78010=DIRECTION('ref_axis',(1.11050837170941E-63,1.,1.83697019872103E-16)) ;
#78011=DIRECTION('center_axis',(0.,0.,1.)) ;
#78012=DIRECTION('ref_axis',(1.,0.,0.)) ;
#78013=DIRECTION('center_axis',(-4.27339674608664E-31,1.,-2.10694726592902E-62)) ;
#78014=DIRECTION('ref_axis',(-1.,-4.27339674608664E-31,9.00382159039722E-93)) ;
#78015=DIRECTION('center_axis',(0.,1.,0.)) ;
#78016=DIRECTION('ref_axis',(0.,0.,1.)) ;
#78017=DIRECTION('center_axis',(-8.13512808509168E-31,-9.86076131526265E-32,
1.)) ;
#78018=DIRECTION('ref_axis',(1.,-8.02185563161788E-62,8.13512808509168E-31)) ;
#78019=DIRECTION('center_axis',(0.,0.,-1.)) ;
#78020=DIRECTION('ref_axis',(-1.,0.,0.)) ;
#78021=DIRECTION('center_axis',(1.,-4.27339674608665E-31,4.93038065763132E-32)) ;
#78022=DIRECTION('ref_axis',(4.27339674608665E-31,1.,2.10694726592902E-62)) ;
#78023=DIRECTION('center_axis',(-1.,-1.75279351218489E-14,0.)) ;
#78024=DIRECTION('ref_axis',(1.75279351218489E-14,-1.,0.)) ;
#78025=DIRECTION('center_axis',(-1.,5.06932053596301E-14,2.51253409742467E-28)) ;
#78026=DIRECTION('ref_axis',(-5.06859511626947E-14,-1.,0.)) ;
#78027=DIRECTION('center_axis',(0.,0.,1.)) ;
#78028=DIRECTION('ref_axis',(1.,0.,0.)) ;
#78029=DIRECTION('center_axis',(-4.15069017696469E-34,1.,1.83697019872103E-16)) ;
#78030=DIRECTION('ref_axis',(0.,-1.85037170770859E-16,1.)) ;
#78031=DIRECTION('center_axis',(-4.15069017696469E-34,1.,1.83697019872103E-16)) ;
#78032=DIRECTION('ref_axis',(1.24381980576027E-51,-1.83697019872103E-16,
1.)) ;
#78033=DIRECTION('center_axis',(-1.,0.,0.)) ;
#78034=DIRECTION('ref_axis',(0.,-9.03501810404582E-16,-1.)) ;
#78035=DIRECTION('center_axis',(-4.93038065763132E-32,0.,1.)) ;
#78036=DIRECTION('ref_axis',(1.,0.,0.)) ;
#78037=DIRECTION('center_axis',(-1.,0.,0.)) ;
#78038=DIRECTION('ref_axis',(0.,0.,-1.)) ;
#78039=DIRECTION('center_axis',(-4.93038065763132E-32,0.,1.)) ;
#78040=DIRECTION('ref_axis',(1.,0.,4.93038065763132E-32)) ;
#78041=DIRECTION('center_axis',(0.,1.,0.)) ;
#78042=DIRECTION('ref_axis',(1.,0.,0.)) ;
#78043=DIRECTION('center_axis',(0.,1.,0.)) ;
#78044=DIRECTION('ref_axis',(-1.77086354839302E-14,0.,-1.)) ;
#78045=DIRECTION('center_axis',(6.04532600737121E-48,-1.83697019872103E-16,
1.)) ;
#78046=DIRECTION('ref_axis',(-1.11050837170941E-63,-1.,-1.83697019872103E-16)) ;
#78047=DIRECTION('center_axis',(0.,0.,1.)) ;
#78048=DIRECTION('ref_axis',(1.,0.,0.)) ;
#78049=DIRECTION('center_axis',(3.29092219981587E-32,-1.,-1.83697019872103E-16)) ;
#78050=DIRECTION('ref_axis',(-6.04532600737121E-48,1.83697019872103E-16,
-1.)) ;
#78051=DIRECTION('center_axis',(-4.15069017696469E-34,1.,1.83697019872103E-16)) ;
#78052=DIRECTION('ref_axis',(7.62469415920825E-50,-1.83697019872103E-16,
1.)) ;
#78053=DIRECTION('center_axis',(-1.,-4.15069017696469E-34,-7.62469415920825E-50)) ;
#78054=DIRECTION('ref_axis',(4.15069017696469E-34,-1.,3.16477431489857E-83)) ;
#78055=DIRECTION('center_axis',(-1.,0.,-1.73472347597682E-14)) ;
#78056=DIRECTION('ref_axis',(-1.73472347597682E-14,0.,1.)) ;
#78057=DIRECTION('center_axis',(1.,-4.27339674608665E-31,4.93038065763132E-32)) ;
#78058=DIRECTION('ref_axis',(4.27339674608665E-31,1.,2.10694726592902E-62)) ;
#78059=DIRECTION('center_axis',(-1.,0.,-3.90312782094789E-14)) ;
#78060=DIRECTION('ref_axis',(-3.90312782094789E-14,0.,1.)) ;
#78061=DIRECTION('center_axis',(8.13512808509168E-31,9.86076131526265E-32,
-1.)) ;
#78062=DIRECTION('ref_axis',(-1.,8.02185563161788E-62,-8.13512808509168E-31)) ;
#78063=DIRECTION('center_axis',(-4.93038065763132E-32,0.,1.)) ;
#78064=DIRECTION('ref_axis',(1.,0.,4.93038065763132E-32)) ;
#78065=DIRECTION('center_axis',(4.27339674608664E-31,-1.,2.10694726592902E-62)) ;
#78066=DIRECTION('ref_axis',(1.,4.27339674608664E-31,-9.00382159039724E-93)) ;
#78067=DIRECTION('center_axis',(0.,1.,0.)) ;
#78068=DIRECTION('ref_axis',(0.,0.,1.)) ;
#78069=DIRECTION('center_axis',(-4.15069017696469E-34,1.,1.83697019872103E-16)) ;
#78070=DIRECTION('ref_axis',(0.,0.,1.)) ;
#78071=DIRECTION('center_axis',(-1.,0.,0.)) ;
#78072=DIRECTION('ref_axis',(0.,0.,-1.)) ;
#78073=DIRECTION('center_axis',(0.,1.,0.)) ;
#78074=DIRECTION('ref_axis',(1.,0.,0.)) ;
#78075=DIRECTION('center_axis',(0.,1.15648231731787E-14,1.)) ;
#78076=DIRECTION('ref_axis',(-1.73472347597681E-14,1.,-1.15648231731787E-14)) ;
#78077=DIRECTION('center_axis',(0.,-1.,-1.80700362080916E-16)) ;
#78078=DIRECTION('ref_axis',(0.,-1.80700362080916E-16,1.)) ;
#78079=DIRECTION('center_axis',(0.,1.,0.)) ;
#78080=DIRECTION('ref_axis',(1.,0.,0.)) ;
#78081=DIRECTION('center_axis',(0.,0.,-1.)) ;
#78082=DIRECTION('ref_axis',(1.,0.,0.)) ;
#78083=DIRECTION('center_axis',(-5.78241158658958E-15,1.,0.)) ;
#78084=DIRECTION('ref_axis',(1.,5.78241158658958E-15,0.)) ;
#78085=DIRECTION('center_axis',(-4.93038065763132E-32,0.,1.)) ;
#78086=DIRECTION('ref_axis',(1.,0.,0.)) ;
#78087=DIRECTION('center_axis',(-1.,0.,0.)) ;
#78088=DIRECTION('ref_axis',(0.,0.,-1.)) ;
#78089=DIRECTION('center_axis',(1.,4.15069017696469E-34,7.62469415920825E-50)) ;
#78090=DIRECTION('ref_axis',(-4.15069017696469E-34,1.,-3.16477431489857E-83)) ;
#78091=DIRECTION('center_axis',(-1.,0.,0.)) ;
#78092=DIRECTION('ref_axis',(0.,0.,1.)) ;
#78093=DIRECTION('center_axis',(-3.29092219981587E-32,1.,1.83697019872103E-16)) ;
#78094=DIRECTION('ref_axis',(6.04532600737121E-48,-1.83697019872103E-16,
1.)) ;
#78095=DIRECTION('center_axis',(0.,-1.,0.)) ;
#78096=DIRECTION('ref_axis',(0.,0.,-1.)) ;
#78097=DIRECTION('center_axis',(6.04532600737121E-48,-1.83697019872103E-16,
1.)) ;
#78098=DIRECTION('ref_axis',(-1.11050837170941E-63,-1.,-1.83697019872103E-16)) ;
#78099=DIRECTION('center_axis',(-1.15648231731789E-14,0.,1.)) ;
#78100=DIRECTION('ref_axis',(1.,0.,1.15648231731789E-14)) ;
#78101=DIRECTION('center_axis',(2.16840434497101E-16,-1.,1.06910588403688E-47)) ;
#78102=DIRECTION('ref_axis',(1.,2.16840434497101E-16,-2.31825384417965E-63)) ;
#78103=DIRECTION('center_axis',(0.,1.,5.78241158658946E-15)) ;
#78104=DIRECTION('ref_axis',(0.,-5.78241158658946E-15,1.)) ;
#78105=DIRECTION('center_axis',(-7.39557098644699E-31,-9.86076131526265E-32,
1.)) ;
#78106=DIRECTION('ref_axis',(1.,-7.29259602874353E-62,7.39557098644699E-31)) ;
#78107=DIRECTION('center_axis',(0.,0.,-1.)) ;
#78108=DIRECTION('ref_axis',(-1.,0.,0.)) ;
#78109=DIRECTION('center_axis',(-1.,4.27339674608665E-31,-4.93038065763132E-32)) ;
#78110=DIRECTION('ref_axis',(-4.27339674608665E-31,-1.,-2.10694726592902E-62)) ;
#78111=DIRECTION('center_axis',(-1.,0.,0.)) ;
#78112=DIRECTION('ref_axis',(0.,0.,1.)) ;
#78113=DIRECTION('center_axis',(0.,1.,0.)) ;
#78114=DIRECTION('ref_axis',(1.,0.,0.)) ;
#78115=DIRECTION('center_axis',(0.,0.,1.)) ;
#78116=DIRECTION('ref_axis',(-1.,0.,0.)) ;
#78117=DIRECTION('center_axis',(0.,1.,0.)) ;
#78118=DIRECTION('ref_axis',(1.,0.,0.)) ;
#78119=DIRECTION('center_axis',(1.,1.73472347597681E-14,3.13465160219275E-30)) ;
#78120=DIRECTION('ref_axis',(1.73472347597681E-14,-1.,-6.13284536654788E-60)) ;
#78121=DIRECTION('center_axis',(0.,-1.,-1.80700362080916E-16)) ;
#78122=DIRECTION('ref_axis',(0.,-1.80700362080916E-16,1.)) ;
#78123=DIRECTION('center_axis',(-1.,-3.29092219981587E-32,0.)) ;
#78124=DIRECTION('ref_axis',(0.,-1.,0.)) ;
#78125=DIRECTION('center_axis',(-5.34873071759516E-14,-1.,7.22801448323682E-15)) ;
#78126=DIRECTION('ref_axis',(1.,-5.34873071759516E-14,2.24207754291971E-43)) ;
#78127=DIRECTION('center_axis',(0.,0.,-1.)) ;
#78128=DIRECTION('ref_axis',(-1.,0.,0.)) ;
#78129=DIRECTION('center_axis',(0.,1.,0.)) ;
#78130=DIRECTION('ref_axis',(1.,0.,0.)) ;
#78131=DIRECTION('center_axis',(0.,0.,-1.)) ;
#78132=DIRECTION('ref_axis',(1.,0.,0.)) ;
#78133=DIRECTION('center_axis',(1.,-3.90312782094779E-14,0.)) ;
#78134=DIRECTION('ref_axis',(-3.90312782094779E-14,-1.,0.)) ;
#78135=DIRECTION('center_axis',(0.,1.,0.)) ;
#78136=DIRECTION('ref_axis',(1.,0.,0.)) ;
#78137=DIRECTION('center_axis',(0.,1.,0.)) ;
#78138=DIRECTION('ref_axis',(0.,0.,-1.)) ;
#78139=DIRECTION('center_axis',(-6.04532600737121E-48,1.83697019872103E-16,
-1.)) ;
#78140=DIRECTION('ref_axis',(1.11050837170941E-63,1.,1.83697019872103E-16)) ;
#78141=DIRECTION('center_axis',(0.,0.,1.)) ;
#78142=DIRECTION('ref_axis',(1.,0.,0.)) ;
#78143=DIRECTION('center_axis',(-3.29092219981587E-32,1.,1.83697019872103E-16)) ;
#78144=DIRECTION('ref_axis',(6.04532600737121E-48,-1.83697019872103E-16,
1.)) ;
#78145=DIRECTION('center_axis',(0.,-1.,0.)) ;
#78146=DIRECTION('ref_axis',(0.,0.,-1.)) ;
#78147=DIRECTION('center_axis',(1.,4.15069017696469E-34,7.62469415920825E-50)) ;
#78148=DIRECTION('ref_axis',(-4.15069017696469E-34,1.,-3.16477431489857E-83)) ;
#78149=DIRECTION('center_axis',(1.,0.,0.)) ;
#78150=DIRECTION('ref_axis',(0.,0.,-1.)) ;
#78151=DIRECTION('center_axis',(-6.04532600737121E-48,1.83697019872103E-16,
-1.)) ;
#78152=DIRECTION('ref_axis',(1.11050837170941E-63,1.,1.83697019872103E-16)) ;
#78153=DIRECTION('center_axis',(0.,0.,-1.)) ;
#78154=DIRECTION('ref_axis',(-1.,0.,0.)) ;
#78155=DIRECTION('center_axis',(-4.27339674608664E-31,1.,-2.10694726592902E-62)) ;
#78156=DIRECTION('ref_axis',(-1.,-4.27339674608664E-31,9.00382159039722E-93)) ;
#78157=DIRECTION('center_axis',(0.,-1.,0.)) ;
#78158=DIRECTION('ref_axis',(0.,0.,-1.)) ;
#78159=DIRECTION('center_axis',(-1.,4.27339674608665E-31,-4.93038065763132E-32)) ;
#78160=DIRECTION('ref_axis',(-4.27339674608665E-31,-1.,-2.10694726592902E-62)) ;
#78161=DIRECTION('center_axis',(1.,0.,0.)) ;
#78162=DIRECTION('ref_axis',(0.,0.,-1.)) ;
#78163=DIRECTION('center_axis',(-7.39557098644699E-31,-9.86076131526265E-32,
1.)) ;
#78164=DIRECTION('ref_axis',(1.,-7.29259602874353E-62,7.39557098644699E-31)) ;
#78165=DIRECTION('center_axis',(0.,0.,-1.)) ;
#78166=DIRECTION('ref_axis',(-1.,0.,0.)) ;
#78167=DIRECTION('center_axis',(-2.16840434497101E-16,1.,-1.06910588403688E-47)) ;
#78168=DIRECTION('ref_axis',(-1.,-2.16840434497101E-16,2.31825384417965E-63)) ;
#78169=DIRECTION('center_axis',(0.,1.,0.)) ;
#78170=DIRECTION('ref_axis',(0.,0.,1.)) ;
#78171=DIRECTION('center_axis',(0.,1.,0.)) ;
#78172=DIRECTION('ref_axis',(1.,0.,0.)) ;
#78173=DIRECTION('center_axis',(1.,0.,0.)) ;
#78174=DIRECTION('ref_axis',(0.,0.,1.)) ;
#78175=DIRECTION('center_axis',(-4.15069017696469E-34,1.,1.83697019872103E-16)) ;
#78176=DIRECTION('ref_axis',(0.,-1.85037170770859E-16,1.)) ;
#78177=DIRECTION('center_axis',(-4.15069017696469E-34,1.,1.83697019872103E-16)) ;
#78178=DIRECTION('ref_axis',(1.24381980576027E-51,-1.83697019872103E-16,
1.)) ;
#78179=DIRECTION('center_axis',(-4.93038065763132E-32,0.,1.)) ;
#78180=DIRECTION('ref_axis',(1.,0.,0.)) ;
#78181=DIRECTION('center_axis',(-4.93038065763132E-32,0.,1.)) ;
#78182=DIRECTION('ref_axis',(1.,0.,4.93038065763132E-32)) ;
#78183=DIRECTION('center_axis',(0.,1.,0.)) ;
#78184=DIRECTION('ref_axis',(1.,0.,0.)) ;
#78185=DIRECTION('center_axis',(1.,0.,0.)) ;
#78186=DIRECTION('ref_axis',(0.,0.,1.)) ;
#78187=DIRECTION('center_axis',(-1.,-4.15069017696469E-34,-7.62469415920825E-50)) ;
#78188=DIRECTION('ref_axis',(4.15069017696469E-34,-1.,3.16477431489857E-83)) ;
#78189=DIRECTION('center_axis',(1.,0.,0.)) ;
#78190=DIRECTION('ref_axis',(0.,0.,-1.)) ;
#78191=DIRECTION('center_axis',(3.29092219981587E-32,-1.,-1.83697019872103E-16)) ;
#78192=DIRECTION('ref_axis',(-6.04532600737121E-48,1.83697019872103E-16,
-1.)) ;
#78193=DIRECTION('center_axis',(-4.15069017696469E-34,1.,1.83697019872103E-16)) ;
#78194=DIRECTION('ref_axis',(7.62469415920825E-50,-1.83697019872103E-16,
1.)) ;
#78195=DIRECTION('center_axis',(8.13512808509168E-31,9.86076131526265E-32,
-1.)) ;
#78196=DIRECTION('ref_axis',(-1.,8.02185563161788E-62,-8.13512808509168E-31)) ;
#78197=DIRECTION('center_axis',(-4.93038065763132E-32,0.,1.)) ;
#78198=DIRECTION('ref_axis',(1.,0.,4.93038065763132E-32)) ;
#78199=DIRECTION('center_axis',(1.,-4.27339674608665E-31,4.93038065763132E-32)) ;
#78200=DIRECTION('ref_axis',(4.27339674608665E-31,1.,2.10694726592902E-62)) ;
#78201=DIRECTION('center_axis',(1.,0.,0.)) ;
#78202=DIRECTION('ref_axis',(0.,0.,-1.)) ;
#78203=DIRECTION('center_axis',(-4.15069017696469E-34,1.,1.83697019872103E-16)) ;
#78204=DIRECTION('ref_axis',(0.,0.,1.)) ;
#78205=DIRECTION('center_axis',(0.,0.,1.)) ;
#78206=DIRECTION('ref_axis',(-1.,0.,0.)) ;
#78207=DIRECTION('center_axis',(-4.93038065763132E-32,0.,1.)) ;
#78208=DIRECTION('ref_axis',(1.,0.,0.)) ;
#78209=DIRECTION('center_axis',(0.,1.,0.)) ;
#78210=DIRECTION('ref_axis',(-1.77086354839302E-14,0.,-1.)) ;
#78211=DIRECTION('center_axis',(6.04532600737121E-48,-1.83697019872103E-16,
1.)) ;
#78212=DIRECTION('ref_axis',(-1.11050837170941E-63,-1.,-1.83697019872103E-16)) ;
#78213=DIRECTION('center_axis',(0.,0.,1.)) ;
#78214=DIRECTION('ref_axis',(1.,0.,0.)) ;
#78215=DIRECTION('center_axis',(4.27339674608664E-31,-1.,2.10694726592902E-62)) ;
#78216=DIRECTION('ref_axis',(1.,4.27339674608664E-31,-9.00382159039724E-93)) ;
#78217=DIRECTION('center_axis',(4.48136897960683E-14,1.,0.)) ;
#78218=DIRECTION('ref_axis',(-1.,4.48136897960683E-14,0.)) ;
#78219=DIRECTION('center_axis',(-1.,-3.29092219981587E-32,0.)) ;
#78220=DIRECTION('ref_axis',(0.,-1.,0.)) ;
#78221=DIRECTION('center_axis',(-1.,3.32023598379838E-46,-4.72515227845561E-31)) ;
#78222=DIRECTION('ref_axis',(-4.72515227845561E-31,1.56886206238552E-76,
1.)) ;
#78223=DIRECTION('center_axis',(-1.,0.,0.)) ;
#78224=DIRECTION('ref_axis',(0.,0.,1.)) ;
#78225=DIRECTION('center_axis',(1.,0.,0.)) ;
#78226=DIRECTION('ref_axis',(0.,0.,-1.)) ;
#78227=DIRECTION('center_axis',(4.72515227845561E-31,7.02672800395669E-16,
-1.)) ;
#78228=DIRECTION('ref_axis',(0.,1.,0.)) ;
#78229=DIRECTION('center_axis',(4.72515227845561E-31,7.02672800395669E-16,
-1.)) ;
#78230=DIRECTION('ref_axis',(-3.32023598379838E-46,1.,7.02672800395669E-16)) ;
#78231=DIRECTION('center_axis',(0.,-1.,0.)) ;
#78232=DIRECTION('ref_axis',(0.,0.,1.)) ;
#78233=DIRECTION('center_axis',(4.72515227845561E-31,7.02672800395669E-16,
-1.)) ;
#78234=DIRECTION('ref_axis',(0.,1.,0.)) ;
#78235=DIRECTION('center_axis',(0.,-1.,0.)) ;
#78236=DIRECTION('ref_axis',(0.,0.,1.)) ;
#78237=DIRECTION('center_axis',(4.72515227845561E-31,7.02672800395669E-16,
-1.)) ;
#78238=DIRECTION('ref_axis',(-3.32023598379838E-46,1.,7.02672800395669E-16)) ;
#78239=DIRECTION('center_axis',(-4.72515227845561E-31,-7.02672800395669E-16,
1.)) ;
#78240=DIRECTION('ref_axis',(3.32023598379838E-46,-1.,-7.02672800395669E-16)) ;
#78241=DIRECTION('center_axis',(4.72515227845561E-31,7.02672800395669E-16,
-1.)) ;
#78242=DIRECTION('ref_axis',(-3.32023598379838E-46,1.,7.02672800395669E-16)) ;
#78243=DIRECTION('center_axis',(-8.67361737988404E-17,-1.,-7.02672800395669E-16)) ;
#78244=DIRECTION('ref_axis',(6.09471501388366E-32,7.02672800395669E-16,
-1.)) ;
#78245=DIRECTION('center_axis',(0.,-1.,0.)) ;
#78246=DIRECTION('ref_axis',(0.,0.,-1.)) ;
#78247=DIRECTION('center_axis',(1.,-3.32023598379838E-46,4.72515227845561E-31)) ;
#78248=DIRECTION('ref_axis',(4.72515227845561E-31,-1.56886206238552E-76,
-1.)) ;
#78249=DIRECTION('center_axis',(1.,0.,0.)) ;
#78250=DIRECTION('ref_axis',(0.,0.,-1.)) ;
#78251=DIRECTION('center_axis',(-1.,0.,0.)) ;
#78252=DIRECTION('ref_axis',(0.,0.,1.)) ;
#78253=DIRECTION('center_axis',(1.73472347597681E-16,1.,7.02672800395669E-16)) ;
#78254=DIRECTION('ref_axis',(-1.21894300277673E-31,-7.02672800395669E-16,
1.)) ;
#78255=DIRECTION('center_axis',(0.,-1.,0.)) ;
#78256=DIRECTION('ref_axis',(0.,0.,-1.)) ;
#78257=DIRECTION('center_axis',(-4.72515227845561E-31,-7.02672800395669E-16,
1.)) ;
#78258=DIRECTION('ref_axis',(3.32023598379838E-46,-1.,-7.02672800395669E-16)) ;
#78259=DIRECTION('center_axis',(4.72515227845561E-31,7.02672800395669E-16,
-1.)) ;
#78260=DIRECTION('ref_axis',(-3.32023598379838E-46,1.,7.02672800395669E-16)) ;
#78261=DIRECTION('center_axis',(-1.,3.32023598379838E-46,-4.72515227845561E-31)) ;
#78262=DIRECTION('ref_axis',(-4.72515227845561E-31,1.56886206238552E-76,
1.)) ;
#78263=DIRECTION('center_axis',(1.,0.,0.)) ;
#78264=DIRECTION('ref_axis',(0.,0.,-1.)) ;
#78265=DIRECTION('center_axis',(-1.,0.,0.)) ;
#78266=DIRECTION('ref_axis',(0.,0.,1.)) ;
#78267=DIRECTION('center_axis',(4.72515227845561E-31,7.02672800395669E-16,
-1.)) ;
#78268=DIRECTION('ref_axis',(0.,1.,0.)) ;
#78269=DIRECTION('center_axis',(0.,-1.,0.)) ;
#78270=DIRECTION('ref_axis',(0.,0.,1.)) ;
#78271=DIRECTION('center_axis',(4.72515227845561E-31,7.02672800395669E-16,
-1.)) ;
#78272=DIRECTION('ref_axis',(0.,1.,0.)) ;
#78273=DIRECTION('center_axis',(4.72515227845561E-31,7.02672800395669E-16,
-1.)) ;
#78274=DIRECTION('ref_axis',(-3.32023598379837E-46,1.,7.02672800395669E-16)) ;
#78275=DIRECTION('center_axis',(4.72515227845561E-31,7.02672800395669E-16,
-1.)) ;
#78276=DIRECTION('ref_axis',(0.,1.,0.)) ;
#78277=DIRECTION('center_axis',(4.72515227845561E-31,7.02672800395669E-16,
-1.)) ;
#78278=DIRECTION('ref_axis',(-3.32023598379837E-46,1.,7.02672800395669E-16)) ;
#78279=DIRECTION('center_axis',(4.72515227845561E-31,7.02672800395669E-16,
-1.)) ;
#78280=DIRECTION('ref_axis',(0.,1.,0.)) ;
#78281=DIRECTION('center_axis',(0.,-1.,0.)) ;
#78282=DIRECTION('ref_axis',(0.,0.,1.)) ;
#78283=DIRECTION('center_axis',(-8.67361737988404E-17,-1.,-7.02672800395669E-16)) ;
#78284=DIRECTION('ref_axis',(6.09471501388366E-32,7.02672800395669E-16,
-1.)) ;
#78285=DIRECTION('center_axis',(0.,-1.,0.)) ;
#78286=DIRECTION('ref_axis',(0.,0.,-1.)) ;
#78287=DIRECTION('center_axis',(-4.72515227845561E-31,-7.02672800395669E-16,
1.)) ;
#78288=DIRECTION('ref_axis',(3.32023598379837E-46,-1.,-7.02672800395669E-16)) ;
#78289=DIRECTION('center_axis',(4.72515227845561E-31,7.02672800395669E-16,
-1.)) ;
#78290=DIRECTION('ref_axis',(-3.32023598379837E-46,1.,7.02672800395669E-16)) ;
#78291=DIRECTION('center_axis',(-4.72515227845561E-31,-7.02672800395669E-16,
1.)) ;
#78292=DIRECTION('ref_axis',(3.32023598379837E-46,-1.,-7.02672800395669E-16)) ;
#78293=DIRECTION('center_axis',(4.72515227845561E-31,7.02672800395669E-16,
-1.)) ;
#78294=DIRECTION('ref_axis',(-3.32023598379837E-46,1.,7.02672800395669E-16)) ;
#78295=DIRECTION('center_axis',(1.73472347597681E-16,1.,7.02672800395669E-16)) ;
#78296=DIRECTION('ref_axis',(-1.21894300277673E-31,-7.02672800395669E-16,
1.)) ;
#78297=DIRECTION('center_axis',(0.,-1.,0.)) ;
#78298=DIRECTION('ref_axis',(0.,0.,-1.)) ;
#78299=DIRECTION('center_axis',(4.72515227845561E-31,7.02672800395669E-16,
-1.)) ;
#78300=DIRECTION('ref_axis',(0.,1.,0.)) ;
#78301=DIRECTION('center_axis',(1.,0.,0.)) ;
#78302=DIRECTION('ref_axis',(0.,0.,1.)) ;
#78303=DIRECTION('center_axis',(4.72515227845561E-31,7.02672800395669E-16,
-1.)) ;
#78304=DIRECTION('ref_axis',(0.,1.,0.)) ;
#78305=DIRECTION('center_axis',(-1.,0.,0.)) ;
#78306=DIRECTION('ref_axis',(0.,0.,-1.)) ;
#78307=DIRECTION('center_axis',(1.,-3.32023598379838E-46,4.72515227845561E-31)) ;
#78308=DIRECTION('ref_axis',(4.72515227845561E-31,-1.56886206238552E-76,
-1.)) ;
#78309=DIRECTION('center_axis',(1.,-3.32023598379838E-46,4.72515227845561E-31)) ;
#78310=DIRECTION('ref_axis',(4.72515227845561E-31,-1.56886206238552E-76,
-1.)) ;
#78311=DIRECTION('center_axis',(1.,0.,0.)) ;
#78312=DIRECTION('ref_axis',(0.,0.,-1.)) ;
#78313=DIRECTION('center_axis',(-1.,0.,0.)) ;
#78314=DIRECTION('ref_axis',(0.,0.,1.)) ;
#78315=DIRECTION('center_axis',(4.72515227845561E-31,7.02672800395669E-16,
-1.)) ;
#78316=DIRECTION('ref_axis',(0.,1.,0.)) ;
#78317=DIRECTION('center_axis',(4.72515227845561E-31,7.02672800395669E-16,
-1.)) ;
#78318=DIRECTION('ref_axis',(-3.32023598379837E-46,1.,7.02672800395669E-16)) ;
#78319=DIRECTION('center_axis',(0.,1.,0.)) ;
#78320=DIRECTION('ref_axis',(0.,0.,-1.)) ;
#78321=DIRECTION('center_axis',(4.72515227845561E-31,7.02672800395669E-16,
-1.)) ;
#78322=DIRECTION('ref_axis',(0.,1.,0.)) ;
#78323=DIRECTION('center_axis',(0.,1.,0.)) ;
#78324=DIRECTION('ref_axis',(0.,0.,-1.)) ;
#78325=DIRECTION('center_axis',(4.72515227845561E-31,7.02672800395669E-16,
-1.)) ;
#78326=DIRECTION('ref_axis',(-3.32023598379837E-46,1.,7.02672800395669E-16)) ;
#78327=DIRECTION('center_axis',(-4.72515227845561E-31,-7.02672800395669E-16,
1.)) ;
#78328=DIRECTION('ref_axis',(3.32023598379837E-46,-1.,-7.02672800395669E-16)) ;
#78329=DIRECTION('center_axis',(4.72515227845561E-31,7.02672800395669E-16,
-1.)) ;
#78330=DIRECTION('ref_axis',(-3.32023598379837E-46,1.,7.02672800395669E-16)) ;
#78331=DIRECTION('center_axis',(3.46944695195361E-16,1.,7.02672800395669E-16)) ;
#78332=DIRECTION('ref_axis',(-2.43788600555346E-31,-7.02672800395669E-16,
1.)) ;
#78333=DIRECTION('center_axis',(0.,1.,0.)) ;
#78334=DIRECTION('ref_axis',(0.,0.,1.)) ;
#78335=DIRECTION('center_axis',(-1.,3.32023598379838E-46,-4.72515227845561E-31)) ;
#78336=DIRECTION('ref_axis',(-4.72515227845561E-31,1.56886206238552E-76,
1.)) ;
#78337=DIRECTION('center_axis',(-1.,0.,0.)) ;
#78338=DIRECTION('ref_axis',(0.,0.,1.)) ;
#78339=DIRECTION('center_axis',(1.,0.,0.)) ;
#78340=DIRECTION('ref_axis',(0.,0.,-1.)) ;
#78341=DIRECTION('center_axis',(-1.73472347597681E-16,-1.,-7.02672800395669E-16)) ;
#78342=DIRECTION('ref_axis',(1.21894300277673E-31,7.02672800395669E-16,
-1.)) ;
#78343=DIRECTION('center_axis',(0.,1.,0.)) ;
#78344=DIRECTION('ref_axis',(0.,0.,1.)) ;
#78345=DIRECTION('center_axis',(-4.72515227845561E-31,-7.02672800395669E-16,
1.)) ;
#78346=DIRECTION('ref_axis',(3.32023598379837E-46,-1.,-7.02672800395669E-16)) ;
#78347=DIRECTION('center_axis',(4.72515227845561E-31,7.02672800395669E-16,
-1.)) ;
#78348=DIRECTION('ref_axis',(-3.32023598379837E-46,1.,7.02672800395669E-16)) ;
#78349=DIRECTION('center_axis',(1.,-3.32023598379838E-46,4.72515227845561E-31)) ;
#78350=DIRECTION('ref_axis',(4.72515227845561E-31,-1.56886206238552E-76,
-1.)) ;
#78351=DIRECTION('center_axis',(-1.,0.,0.)) ;
#78352=DIRECTION('ref_axis',(0.,0.,1.)) ;
#78353=DIRECTION('center_axis',(1.,0.,0.)) ;
#78354=DIRECTION('ref_axis',(0.,0.,-1.)) ;
#78355=DIRECTION('center_axis',(4.72515227845561E-31,7.02672800395669E-16,
-1.)) ;
#78356=DIRECTION('ref_axis',(0.,1.,0.)) ;
#78357=DIRECTION('center_axis',(0.,1.,0.)) ;
#78358=DIRECTION('ref_axis',(0.,0.,-1.)) ;
#78359=DIRECTION('center_axis',(4.72515227845561E-31,7.02672800395669E-16,
-1.)) ;
#78360=DIRECTION('ref_axis',(0.,1.,0.)) ;
#78361=DIRECTION('center_axis',(4.72515227845561E-31,7.02672800395669E-16,
-1.)) ;
#78362=DIRECTION('ref_axis',(-3.32023598379838E-46,1.,7.02672800395669E-16)) ;
#78363=DIRECTION('center_axis',(4.72515227845561E-31,7.02672800395669E-16,
-1.)) ;
#78364=DIRECTION('ref_axis',(0.,1.,0.)) ;
#78365=DIRECTION('center_axis',(4.72515227845561E-31,7.02672800395669E-16,
-1.)) ;
#78366=DIRECTION('ref_axis',(-3.32023598379838E-46,1.,7.02672800395669E-16)) ;
#78367=DIRECTION('center_axis',(4.72515227845561E-31,7.02672800395669E-16,
-1.)) ;
#78368=DIRECTION('ref_axis',(0.,1.,0.)) ;
#78369=DIRECTION('center_axis',(0.,1.,0.)) ;
#78370=DIRECTION('ref_axis',(0.,0.,-1.)) ;
#78371=DIRECTION('center_axis',(3.46944695195361E-16,1.,7.02672800395669E-16)) ;
#78372=DIRECTION('ref_axis',(-2.43788600555346E-31,-7.02672800395669E-16,
1.)) ;
#78373=DIRECTION('center_axis',(0.,1.,0.)) ;
#78374=DIRECTION('ref_axis',(0.,0.,1.)) ;
#78375=DIRECTION('center_axis',(-4.72515227845561E-31,-7.02672800395669E-16,
1.)) ;
#78376=DIRECTION('ref_axis',(3.32023598379838E-46,-1.,-7.02672800395669E-16)) ;
#78377=DIRECTION('center_axis',(4.72515227845561E-31,7.02672800395669E-16,
-1.)) ;
#78378=DIRECTION('ref_axis',(-3.32023598379838E-46,1.,7.02672800395669E-16)) ;
#78379=DIRECTION('center_axis',(-4.72515227845561E-31,-7.02672800395669E-16,
1.)) ;
#78380=DIRECTION('ref_axis',(3.32023598379838E-46,-1.,-7.02672800395669E-16)) ;
#78381=DIRECTION('center_axis',(4.72515227845561E-31,7.02672800395669E-16,
-1.)) ;
#78382=DIRECTION('ref_axis',(-3.32023598379838E-46,1.,7.02672800395669E-16)) ;
#78383=DIRECTION('center_axis',(-1.73472347597681E-16,-1.,-7.02672800395669E-16)) ;
#78384=DIRECTION('ref_axis',(1.21894300277673E-31,7.02672800395669E-16,
-1.)) ;
#78385=DIRECTION('center_axis',(0.,1.,0.)) ;
#78386=DIRECTION('ref_axis',(0.,0.,1.)) ;
#78387=DIRECTION('center_axis',(4.72515227845561E-31,7.02672800395669E-16,
-1.)) ;
#78388=DIRECTION('ref_axis',(0.,1.,0.)) ;
#78389=DIRECTION('center_axis',(-1.,0.,0.)) ;
#78390=DIRECTION('ref_axis',(0.,0.,-1.)) ;
#78391=DIRECTION('center_axis',(4.72515227845561E-31,7.02672800395669E-16,
-1.)) ;
#78392=DIRECTION('ref_axis',(0.,1.,0.)) ;
#78393=DIRECTION('center_axis',(1.,0.,0.)) ;
#78394=DIRECTION('ref_axis',(0.,0.,1.)) ;
#78395=DIRECTION('center_axis',(-1.,3.32023598379838E-46,-4.72515227845561E-31)) ;
#78396=DIRECTION('ref_axis',(-4.72515227845561E-31,1.56886206238552E-76,
1.)) ;
#78397=DIRECTION('center_axis',(-1.,3.32023598379838E-46,-4.72515227845561E-31)) ;
#78398=DIRECTION('ref_axis',(-4.72515227845561E-31,1.56886206238552E-76,
1.)) ;
#78399=DIRECTION('center_axis',(-1.,0.,0.)) ;
#78400=DIRECTION('ref_axis',(0.,0.,1.)) ;
#78401=DIRECTION('center_axis',(1.,0.,0.)) ;
#78402=DIRECTION('ref_axis',(0.,0.,-1.)) ;
#78403=DIRECTION('center_axis',(4.72515227845561E-31,7.02672800395669E-16,
-1.)) ;
#78404=DIRECTION('ref_axis',(0.,1.,0.)) ;
#78405=DIRECTION('center_axis',(4.72515227845561E-31,7.02672800395669E-16,
-1.)) ;
#78406=DIRECTION('ref_axis',(-3.32023598379838E-46,1.,7.02672800395669E-16)) ;
#78407=DIRECTION('center_axis',(0.,-1.,0.)) ;
#78408=DIRECTION('ref_axis',(0.,0.,1.)) ;
#78409=DIRECTION('center_axis',(4.72515227845561E-31,7.02672800395669E-16,
-1.)) ;
#78410=DIRECTION('ref_axis',(0.,1.,0.)) ;
#78411=DIRECTION('center_axis',(0.,-1.,0.)) ;
#78412=DIRECTION('ref_axis',(0.,0.,1.)) ;
#78413=DIRECTION('center_axis',(4.72515227845561E-31,7.02672800395669E-16,
-1.)) ;
#78414=DIRECTION('ref_axis',(-3.32023598379838E-46,1.,7.02672800395669E-16)) ;
#78415=DIRECTION('center_axis',(-4.72515227845561E-31,-7.02672800395669E-16,
1.)) ;
#78416=DIRECTION('ref_axis',(3.32023598379838E-46,-1.,-7.02672800395669E-16)) ;
#78417=DIRECTION('center_axis',(4.72515227845561E-31,7.02672800395669E-16,
-1.)) ;
#78418=DIRECTION('ref_axis',(-3.32023598379838E-46,1.,7.02672800395669E-16)) ;
#78419=DIRECTION('center_axis',(1.97633094273713E-47,-1.,-7.02672800395669E-16)) ;
#78420=DIRECTION('ref_axis',(-1.38871399804171E-62,7.02672800395669E-16,
-1.)) ;
#78421=DIRECTION('center_axis',(0.,-1.,0.)) ;
#78422=DIRECTION('ref_axis',(0.,0.,-1.)) ;
#78423=DIRECTION('center_axis',(1.,-3.32023598379838E-46,4.72515227845561E-31)) ;
#78424=DIRECTION('ref_axis',(4.72515227845561E-31,-1.56886206238552E-76,
-1.)) ;
#78425=DIRECTION('center_axis',(1.,0.,0.)) ;
#78426=DIRECTION('ref_axis',(0.,0.,-1.)) ;
#78427=DIRECTION('center_axis',(-1.,0.,0.)) ;
#78428=DIRECTION('ref_axis',(0.,0.,1.)) ;
#78429=DIRECTION('center_axis',(-1.97633094273713E-47,1.,7.02672800395669E-16)) ;
#78430=DIRECTION('ref_axis',(1.38871399804171E-62,-7.02672800395669E-16,
1.)) ;
#78431=DIRECTION('center_axis',(0.,-1.,0.)) ;
#78432=DIRECTION('ref_axis',(0.,0.,-1.)) ;
#78433=DIRECTION('center_axis',(-4.72515227845561E-31,-7.02672800395669E-16,
1.)) ;
#78434=DIRECTION('ref_axis',(3.32023598379838E-46,-1.,-7.02672800395669E-16)) ;
#78435=DIRECTION('center_axis',(4.72515227845561E-31,7.02672800395669E-16,
-1.)) ;
#78436=DIRECTION('ref_axis',(-3.32023598379838E-46,1.,7.02672800395669E-16)) ;
#78437=DIRECTION('center_axis',(-1.,3.32023598379838E-46,-4.72515227845561E-31)) ;
#78438=DIRECTION('ref_axis',(-4.72515227845561E-31,1.56886206238552E-76,
1.)) ;
#78439=DIRECTION('center_axis',(1.,0.,0.)) ;
#78440=DIRECTION('ref_axis',(0.,0.,-1.)) ;
#78441=DIRECTION('center_axis',(-1.,0.,0.)) ;
#78442=DIRECTION('ref_axis',(0.,0.,1.)) ;
#78443=DIRECTION('center_axis',(4.72515227845561E-31,7.02672800395669E-16,
-1.)) ;
#78444=DIRECTION('ref_axis',(0.,1.,0.)) ;
#78445=DIRECTION('center_axis',(0.,-1.,0.)) ;
#78446=DIRECTION('ref_axis',(0.,0.,1.)) ;
#78447=DIRECTION('center_axis',(4.72515227845561E-31,7.02672800395669E-16,
-1.)) ;
#78448=DIRECTION('ref_axis',(0.,1.,0.)) ;
#78449=DIRECTION('center_axis',(4.72515227845561E-31,7.02672800395669E-16,
-1.)) ;
#78450=DIRECTION('ref_axis',(-3.32023598379837E-46,1.,7.02672800395669E-16)) ;
#78451=DIRECTION('center_axis',(4.72515227845561E-31,7.02672800395669E-16,
-1.)) ;
#78452=DIRECTION('ref_axis',(0.,1.,0.)) ;
#78453=DIRECTION('center_axis',(4.72515227845561E-31,7.02672800395669E-16,
-1.)) ;
#78454=DIRECTION('ref_axis',(-3.32023598379837E-46,1.,7.02672800395669E-16)) ;
#78455=DIRECTION('center_axis',(4.72515227845561E-31,7.02672800395669E-16,
-1.)) ;
#78456=DIRECTION('ref_axis',(0.,1.,0.)) ;
#78457=DIRECTION('center_axis',(0.,-1.,0.)) ;
#78458=DIRECTION('ref_axis',(0.,0.,1.)) ;
#78459=DIRECTION('center_axis',(1.97633094273713E-47,-1.,-7.02672800395669E-16)) ;
#78460=DIRECTION('ref_axis',(-1.38871399804171E-62,7.02672800395669E-16,
-1.)) ;
#78461=DIRECTION('center_axis',(0.,-1.,0.)) ;
#78462=DIRECTION('ref_axis',(0.,0.,-1.)) ;
#78463=DIRECTION('center_axis',(-4.72515227845561E-31,-7.02672800395669E-16,
1.)) ;
#78464=DIRECTION('ref_axis',(3.32023598379837E-46,-1.,-7.02672800395669E-16)) ;
#78465=DIRECTION('center_axis',(4.72515227845561E-31,7.02672800395669E-16,
-1.)) ;
#78466=DIRECTION('ref_axis',(-3.32023598379837E-46,1.,7.02672800395669E-16)) ;
#78467=DIRECTION('center_axis',(-4.72515227845561E-31,-7.02672800395669E-16,
1.)) ;
#78468=DIRECTION('ref_axis',(3.32023598379837E-46,-1.,-7.02672800395669E-16)) ;
#78469=DIRECTION('center_axis',(4.72515227845561E-31,7.02672800395669E-16,
-1.)) ;
#78470=DIRECTION('ref_axis',(-3.32023598379837E-46,1.,7.02672800395669E-16)) ;
#78471=DIRECTION('center_axis',(-1.97633094273713E-47,1.,7.02672800395669E-16)) ;
#78472=DIRECTION('ref_axis',(1.38871399804171E-62,-7.02672800395669E-16,
1.)) ;
#78473=DIRECTION('center_axis',(0.,-1.,0.)) ;
#78474=DIRECTION('ref_axis',(0.,0.,-1.)) ;
#78475=DIRECTION('center_axis',(4.72515227845561E-31,7.02672800395669E-16,
-1.)) ;
#78476=DIRECTION('ref_axis',(0.,1.,0.)) ;
#78477=DIRECTION('center_axis',(1.,0.,0.)) ;
#78478=DIRECTION('ref_axis',(0.,0.,1.)) ;
#78479=DIRECTION('center_axis',(4.72515227845561E-31,7.02672800395669E-16,
-1.)) ;
#78480=DIRECTION('ref_axis',(0.,1.,0.)) ;
#78481=DIRECTION('center_axis',(-1.,0.,0.)) ;
#78482=DIRECTION('ref_axis',(0.,0.,-1.)) ;
#78483=DIRECTION('center_axis',(1.,-3.32023598379838E-46,4.72515227845561E-31)) ;
#78484=DIRECTION('ref_axis',(4.72515227845561E-31,-1.56886206238552E-76,
-1.)) ;
#78485=DIRECTION('center_axis',(1.,-3.32023598379838E-46,4.72515227845561E-31)) ;
#78486=DIRECTION('ref_axis',(4.72515227845561E-31,-1.56886206238552E-76,
-1.)) ;
#78487=DIRECTION('center_axis',(1.,0.,0.)) ;
#78488=DIRECTION('ref_axis',(0.,0.,-1.)) ;
#78489=DIRECTION('center_axis',(-1.,0.,0.)) ;
#78490=DIRECTION('ref_axis',(0.,0.,1.)) ;
#78491=DIRECTION('center_axis',(4.72515227845561E-31,7.02672800395669E-16,
-1.)) ;
#78492=DIRECTION('ref_axis',(0.,1.,0.)) ;
#78493=DIRECTION('center_axis',(4.72515227845561E-31,7.02672800395669E-16,
-1.)) ;
#78494=DIRECTION('ref_axis',(-3.32023598379837E-46,1.,7.02672800395669E-16)) ;
#78495=DIRECTION('center_axis',(0.,1.,0.)) ;
#78496=DIRECTION('ref_axis',(0.,0.,-1.)) ;
#78497=DIRECTION('center_axis',(4.72515227845561E-31,7.02672800395669E-16,
-1.)) ;
#78498=DIRECTION('ref_axis',(0.,1.,0.)) ;
#78499=DIRECTION('center_axis',(0.,1.,0.)) ;
#78500=DIRECTION('ref_axis',(0.,0.,-1.)) ;
#78501=DIRECTION('center_axis',(4.72515227845561E-31,7.02672800395669E-16,
-1.)) ;
#78502=DIRECTION('ref_axis',(-3.32023598379837E-46,1.,7.02672800395669E-16)) ;
#78503=DIRECTION('center_axis',(-4.72515227845561E-31,-7.02672800395669E-16,
1.)) ;
#78504=DIRECTION('ref_axis',(3.32023598379837E-46,-1.,-7.02672800395669E-16)) ;
#78505=DIRECTION('center_axis',(4.72515227845561E-31,7.02672800395669E-16,
-1.)) ;
#78506=DIRECTION('ref_axis',(-3.32023598379837E-46,1.,7.02672800395669E-16)) ;
#78507=DIRECTION('center_axis',(6.93889390390723E-16,1.,7.02672800395669E-16)) ;
#78508=DIRECTION('ref_axis',(-4.87577201110693E-31,-7.02672800395669E-16,
1.)) ;
#78509=DIRECTION('center_axis',(0.,1.,0.)) ;
#78510=DIRECTION('ref_axis',(0.,0.,1.)) ;
#78511=DIRECTION('center_axis',(-1.,3.32023598379838E-46,-4.72515227845561E-31)) ;
#78512=DIRECTION('ref_axis',(-4.72515227845561E-31,1.56886206238552E-76,
1.)) ;
#78513=DIRECTION('center_axis',(-1.,0.,0.)) ;
#78514=DIRECTION('ref_axis',(0.,0.,1.)) ;
#78515=DIRECTION('center_axis',(1.,0.,0.)) ;
#78516=DIRECTION('ref_axis',(0.,0.,-1.)) ;
#78517=DIRECTION('center_axis',(4.15029497974802E-48,-1.,-7.02672800395669E-16)) ;
#78518=DIRECTION('ref_axis',(-2.91629939588763E-63,7.02672800395669E-16,
-1.)) ;
#78519=DIRECTION('center_axis',(0.,1.,0.)) ;
#78520=DIRECTION('ref_axis',(0.,0.,1.)) ;
#78521=DIRECTION('center_axis',(-4.72515227845561E-31,-7.02672800395669E-16,
1.)) ;
#78522=DIRECTION('ref_axis',(3.32023598379837E-46,-1.,-7.02672800395669E-16)) ;
#78523=DIRECTION('center_axis',(4.72515227845561E-31,7.02672800395669E-16,
-1.)) ;
#78524=DIRECTION('ref_axis',(-3.32023598379837E-46,1.,7.02672800395669E-16)) ;
#78525=DIRECTION('center_axis',(1.,-3.32023598379838E-46,4.72515227845561E-31)) ;
#78526=DIRECTION('ref_axis',(4.72515227845561E-31,-1.56886206238552E-76,
-1.)) ;
#78527=DIRECTION('center_axis',(-1.,0.,0.)) ;
#78528=DIRECTION('ref_axis',(0.,0.,1.)) ;
#78529=DIRECTION('center_axis',(1.,0.,0.)) ;
#78530=DIRECTION('ref_axis',(0.,0.,-1.)) ;
#78531=DIRECTION('center_axis',(4.72515227845561E-31,7.02672800395669E-16,
-1.)) ;
#78532=DIRECTION('ref_axis',(0.,1.,0.)) ;
#78533=DIRECTION('center_axis',(0.,1.,0.)) ;
#78534=DIRECTION('ref_axis',(0.,0.,-1.)) ;
#78535=DIRECTION('center_axis',(4.72515227845561E-31,7.02672800395669E-16,
-1.)) ;
#78536=DIRECTION('ref_axis',(0.,1.,0.)) ;
#78537=DIRECTION('center_axis',(4.72515227845561E-31,7.02672800395669E-16,
-1.)) ;
#78538=DIRECTION('ref_axis',(-3.32023598379838E-46,1.,7.02672800395669E-16)) ;
#78539=DIRECTION('center_axis',(4.72515227845561E-31,7.02672800395669E-16,
-1.)) ;
#78540=DIRECTION('ref_axis',(0.,1.,0.)) ;
#78541=DIRECTION('center_axis',(4.72515227845561E-31,7.02672800395669E-16,
-1.)) ;
#78542=DIRECTION('ref_axis',(-3.32023598379838E-46,1.,7.02672800395669E-16)) ;
#78543=DIRECTION('center_axis',(4.72515227845561E-31,7.02672800395669E-16,
-1.)) ;
#78544=DIRECTION('ref_axis',(0.,1.,0.)) ;
#78545=DIRECTION('center_axis',(0.,1.,0.)) ;
#78546=DIRECTION('ref_axis',(0.,0.,-1.)) ;
#78547=DIRECTION('center_axis',(6.93889390390723E-16,1.,7.02672800395669E-16)) ;
#78548=DIRECTION('ref_axis',(-4.87577201110693E-31,-7.02672800395669E-16,
1.)) ;
#78549=DIRECTION('center_axis',(0.,1.,0.)) ;
#78550=DIRECTION('ref_axis',(0.,0.,1.)) ;
#78551=DIRECTION('center_axis',(-4.72515227845561E-31,-7.02672800395669E-16,
1.)) ;
#78552=DIRECTION('ref_axis',(3.32023598379838E-46,-1.,-7.02672800395669E-16)) ;
#78553=DIRECTION('center_axis',(4.72515227845561E-31,7.02672800395669E-16,
-1.)) ;
#78554=DIRECTION('ref_axis',(-3.32023598379838E-46,1.,7.02672800395669E-16)) ;
#78555=DIRECTION('center_axis',(-4.72515227845561E-31,-7.02672800395669E-16,
1.)) ;
#78556=DIRECTION('ref_axis',(3.32023598379838E-46,-1.,-7.02672800395669E-16)) ;
#78557=DIRECTION('center_axis',(4.72515227845561E-31,7.02672800395669E-16,
-1.)) ;
#78558=DIRECTION('ref_axis',(-3.32023598379838E-46,1.,7.02672800395669E-16)) ;
#78559=DIRECTION('center_axis',(4.15029497974802E-48,-1.,-7.02672800395669E-16)) ;
#78560=DIRECTION('ref_axis',(-2.91629939588763E-63,7.02672800395669E-16,
-1.)) ;
#78561=DIRECTION('center_axis',(0.,1.,0.)) ;
#78562=DIRECTION('ref_axis',(0.,0.,1.)) ;
#78563=DIRECTION('center_axis',(4.72515227845561E-31,7.02672800395669E-16,
-1.)) ;
#78564=DIRECTION('ref_axis',(0.,1.,0.)) ;
#78565=DIRECTION('center_axis',(-1.,0.,0.)) ;
#78566=DIRECTION('ref_axis',(0.,0.,-1.)) ;
#78567=DIRECTION('center_axis',(4.72515227845561E-31,7.02672800395669E-16,
-1.)) ;
#78568=DIRECTION('ref_axis',(0.,1.,0.)) ;
#78569=DIRECTION('center_axis',(1.,0.,0.)) ;
#78570=DIRECTION('ref_axis',(0.,0.,1.)) ;
#78571=DIRECTION('center_axis',(-1.,3.32023598379838E-46,-4.72515227845561E-31)) ;
#78572=DIRECTION('ref_axis',(-4.72515227845561E-31,1.56886206238552E-76,
1.)) ;
#78573=DIRECTION('center_axis',(6.7286639138916E-31,2.45734131650226E-45,
-1.)) ;
#78574=DIRECTION('ref_axis',(-1.,1.65346238404636E-75,-6.7286639138916E-31)) ;
#78575=DIRECTION('center_axis',(0.,0.,1.)) ;
#78576=DIRECTION('ref_axis',(1.,0.,0.)) ;
#78577=DIRECTION('center_axis',(0.,0.,-1.)) ;
#78578=DIRECTION('ref_axis',(-1.,0.,0.)) ;
#78579=DIRECTION('center_axis',(-1.,-3.65204942310907E-15,-6.7286639138916E-31)) ;
#78580=DIRECTION('ref_axis',(0.,-1.,0.)) ;
#78581=DIRECTION('center_axis',(0.,1.,0.)) ;
#78582=DIRECTION('ref_axis',(0.,0.,-1.)) ;
#78583=DIRECTION('center_axis',(1.,3.65204942310907E-15,6.7286639138916E-31)) ;
#78584=DIRECTION('ref_axis',(3.65204942310907E-15,-1.,2.45734131650226E-45)) ;
#78585=DIRECTION('center_axis',(-1.,-3.65204942310907E-15,-6.7286639138916E-31)) ;
#78586=DIRECTION('ref_axis',(0.,-1.,0.)) ;
#78587=DIRECTION('center_axis',(1.,3.65204942310907E-15,6.7286639138916E-31)) ;
#78588=DIRECTION('ref_axis',(3.65204942310907E-15,-1.,2.45734131650226E-45)) ;
#78589=DIRECTION('center_axis',(0.,1.,0.)) ;
#78590=DIRECTION('ref_axis',(0.,0.,-1.)) ;
#78591=DIRECTION('center_axis',(-3.65204942310907E-15,1.,3.44027784310316E-46)) ;
#78592=DIRECTION('ref_axis',(-1.,-3.65204942310907E-15,7.32903774880691E-61)) ;
#78593=DIRECTION('center_axis',(-5.78241158658946E-15,1.,0.)) ;
#78594=DIRECTION('ref_axis',(-1.,-5.78241158658946E-15,0.)) ;
#78595=DIRECTION('center_axis',(-1.,-3.65204942310907E-15,-6.7286639138916E-31)) ;
#78596=DIRECTION('ref_axis',(3.65204942310907E-15,-1.,5.11946107604649E-46)) ;
#78597=DIRECTION('center_axis',(1.,3.65204942310907E-15,6.7286639138916E-31)) ;
#78598=DIRECTION('ref_axis',(3.65204942310907E-15,-1.,2.45734131650226E-45)) ;
#78599=DIRECTION('center_axis',(-6.7286639138916E-31,-2.45734131650226E-45,
1.)) ;
#78600=DIRECTION('ref_axis',(1.,6.11909198179539E-89,6.7286639138916E-31)) ;
#78601=DIRECTION('center_axis',(0.,0.,1.)) ;
#78602=DIRECTION('ref_axis',(1.,0.,0.)) ;
#78603=DIRECTION('center_axis',(0.,0.,-1.)) ;
#78604=DIRECTION('ref_axis',(-1.,0.,0.)) ;
#78605=DIRECTION('center_axis',(-1.,-3.65204942310907E-15,-6.7286639138916E-31)) ;
#78606=DIRECTION('ref_axis',(3.65204942310907E-15,-1.,5.11946107604649E-46)) ;
#78607=DIRECTION('center_axis',(1.,3.65204942310907E-15,6.7286639138916E-31)) ;
#78608=DIRECTION('ref_axis',(3.65204942310907E-15,-1.,2.45734131650226E-45)) ;
#78609=DIRECTION('center_axis',(3.65204942310907E-15,-1.,-3.44027784310316E-46)) ;
#78610=DIRECTION('ref_axis',(1.,3.65204942310907E-15,-7.32903774880691E-61)) ;
#78611=DIRECTION('center_axis',(-5.78241158658946E-15,1.,0.)) ;
#78612=DIRECTION('ref_axis',(-1.,-5.78241158658946E-15,0.)) ;
#78613=DIRECTION('center_axis',(-6.7286639138916E-31,-2.45734131650226E-45,
1.)) ;
#78614=DIRECTION('ref_axis',(1.,-1.65346238404636E-75,6.7286639138916E-31)) ;
#78615=DIRECTION('center_axis',(0.,0.,-1.)) ;
#78616=DIRECTION('ref_axis',(-1.,0.,0.)) ;
#78617=DIRECTION('center_axis',(0.,0.,1.)) ;
#78618=DIRECTION('ref_axis',(1.,0.,0.)) ;
#78619=DIRECTION('center_axis',(-1.,-3.65204942310907E-15,-6.7286639138916E-31)) ;
#78620=DIRECTION('ref_axis',(0.,-1.,0.)) ;
#78621=DIRECTION('center_axis',(1.,3.65204942310907E-15,6.7286639138916E-31)) ;
#78622=DIRECTION('ref_axis',(3.65204942310907E-15,-1.,2.45734131650226E-45)) ;
#78623=DIRECTION('center_axis',(-1.,-3.65204942310907E-15,-6.7286639138916E-31)) ;
#78624=DIRECTION('ref_axis',(0.,-1.,0.)) ;
#78625=DIRECTION('center_axis',(0.,1.,0.)) ;
#78626=DIRECTION('ref_axis',(0.,0.,-1.)) ;
#78627=DIRECTION('center_axis',(-1.,-3.65204942310907E-15,-6.7286639138916E-31)) ;
#78628=DIRECTION('ref_axis',(0.,-1.,0.)) ;
#78629=DIRECTION('center_axis',(0.,1.,0.)) ;
#78630=DIRECTION('ref_axis',(0.,0.,-1.)) ;
#78631=DIRECTION('center_axis',(-1.,-3.65204942310907E-15,-6.7286639138916E-31)) ;
#78632=DIRECTION('ref_axis',(0.,-1.,0.)) ;
#78633=DIRECTION('center_axis',(1.,3.65204942310907E-15,6.7286639138916E-31)) ;
#78634=DIRECTION('ref_axis',(3.65204942310907E-15,-1.,2.45734131650226E-45)) ;
#78635=DIRECTION('center_axis',(-1.,-3.65204942310907E-15,-6.7286639138916E-31)) ;
#78636=DIRECTION('ref_axis',(3.65204942310907E-15,-1.,5.11946107604637E-46)) ;
#78637=DIRECTION('center_axis',(1.,3.65204942310907E-15,6.7286639138916E-31)) ;
#78638=DIRECTION('ref_axis',(3.65204942310907E-15,-1.,2.45734131650226E-45)) ;
#78639=DIRECTION('center_axis',(3.65204942310907E-15,-1.,-3.44027784310316E-46)) ;
#78640=DIRECTION('ref_axis',(1.,3.65204942310907E-15,-1.10542957505209E-75)) ;
#78641=DIRECTION('center_axis',(-5.78241158658946E-15,1.,2.67490270053792E-28)) ;
#78642=DIRECTION('ref_axis',(-1.,-5.78241158658946E-15,3.1861838222649E-58)) ;
#78643=DIRECTION('center_axis',(-3.65204942310907E-15,1.,3.44027784310316E-46)) ;
#78644=DIRECTION('ref_axis',(-1.,-3.65204942310907E-15,1.10542957505209E-75)) ;
#78645=DIRECTION('center_axis',(-5.78241158658946E-15,1.,0.)) ;
#78646=DIRECTION('ref_axis',(-1.,-5.78241158658946E-15,0.)) ;
#78647=DIRECTION('center_axis',(-1.,-3.65204942310907E-15,-6.7286639138916E-31)) ;
#78648=DIRECTION('ref_axis',(3.65204942310907E-15,-1.,5.11946107604637E-46)) ;
#78649=DIRECTION('center_axis',(1.,3.65204942310907E-15,6.7286639138916E-31)) ;
#78650=DIRECTION('ref_axis',(3.65204942310907E-15,-1.,2.45734131650226E-45)) ;
#78651=DIRECTION('center_axis',(-1.,-3.65204942310907E-15,-6.7286639138916E-31)) ;
#78652=DIRECTION('ref_axis',(0.,-1.,0.)) ;
#78653=DIRECTION('center_axis',(0.,0.,1.)) ;
#78654=DIRECTION('ref_axis',(-1.,-5.78241158658946E-15,0.)) ;
#78655=DIRECTION('center_axis',(-1.,-3.65204942310907E-15,-6.7286639138916E-31)) ;
#78656=DIRECTION('ref_axis',(0.,-1.,0.)) ;
#78657=DIRECTION('center_axis',(0.,0.,-1.)) ;
#78658=DIRECTION('ref_axis',(1.,0.,0.)) ;
#78659=DIRECTION('center_axis',(6.7286639138916E-31,2.45734131650226E-45,
-1.)) ;
#78660=DIRECTION('ref_axis',(-1.,-6.11909198179539E-89,-6.7286639138916E-31)) ;
#78661=DIRECTION('center_axis',(1.,0.,4.93038065763132E-32)) ;
#78662=DIRECTION('ref_axis',(4.93038065763132E-32,0.,-1.)) ;
#78663=DIRECTION('center_axis',(1.,0.,0.)) ;
#78664=DIRECTION('ref_axis',(0.,0.,-1.)) ;
#78665=DIRECTION('center_axis',(-1.,0.,0.)) ;
#78666=DIRECTION('ref_axis',(0.,0.,1.)) ;
#78667=DIRECTION('center_axis',(-4.93038065763132E-32,0.,1.)) ;
#78668=DIRECTION('ref_axis',(1.,0.,0.)) ;
#78669=DIRECTION('center_axis',(-4.93038065763132E-32,0.,1.)) ;
#78670=DIRECTION('ref_axis',(1.,0.,4.93038065763132E-32)) ;
#78671=DIRECTION('center_axis',(0.,-1.,0.)) ;
#78672=DIRECTION('ref_axis',(0.,0.,1.)) ;
#78673=DIRECTION('center_axis',(-4.93038065763132E-32,0.,1.)) ;
#78674=DIRECTION('ref_axis',(1.,0.,0.)) ;
#78675=DIRECTION('center_axis',(0.,-1.,0.)) ;
#78676=DIRECTION('ref_axis',(0.,0.,1.)) ;
#78677=DIRECTION('center_axis',(-4.93038065763132E-32,0.,1.)) ;
#78678=DIRECTION('ref_axis',(1.,0.,4.93038065763132E-32)) ;
#78679=DIRECTION('center_axis',(0.,0.,-1.)) ;
#78680=DIRECTION('ref_axis',(-1.,0.,0.)) ;
#78681=DIRECTION('center_axis',(-4.93038065763132E-32,0.,1.)) ;
#78682=DIRECTION('ref_axis',(1.,0.,4.93038065763132E-32)) ;
#78683=DIRECTION('center_axis',(0.,-1.,0.)) ;
#78684=DIRECTION('ref_axis',(0.,0.,-1.)) ;
#78685=DIRECTION('center_axis',(0.,-1.,0.)) ;
#78686=DIRECTION('ref_axis',(0.,0.,-1.)) ;
#78687=DIRECTION('center_axis',(-1.,0.,-4.93038065763132E-32)) ;
#78688=DIRECTION('ref_axis',(-4.93038065763132E-32,0.,1.)) ;
#78689=DIRECTION('center_axis',(-1.,0.,0.)) ;
#78690=DIRECTION('ref_axis',(0.,0.,1.)) ;
#78691=DIRECTION('center_axis',(1.,0.,0.)) ;
#78692=DIRECTION('ref_axis',(0.,0.,-1.)) ;
#78693=DIRECTION('center_axis',(0.,1.,0.)) ;
#78694=DIRECTION('ref_axis',(0.,0.,1.)) ;
#78695=DIRECTION('center_axis',(0.,-1.,0.)) ;
#78696=DIRECTION('ref_axis',(0.,0.,-1.)) ;
#78697=DIRECTION('center_axis',(0.,0.,-1.)) ;
#78698=DIRECTION('ref_axis',(-1.,0.,0.)) ;
#78699=DIRECTION('center_axis',(-4.93038065763132E-32,0.,1.)) ;
#78700=DIRECTION('ref_axis',(1.,0.,4.93038065763132E-32)) ;
#78701=DIRECTION('center_axis',(1.,0.,4.93038065763132E-32)) ;
#78702=DIRECTION('ref_axis',(4.93038065763132E-32,0.,-1.)) ;
#78703=DIRECTION('center_axis',(-1.,0.,0.)) ;
#78704=DIRECTION('ref_axis',(0.,0.,1.)) ;
#78705=DIRECTION('center_axis',(1.,0.,0.)) ;
#78706=DIRECTION('ref_axis',(0.,0.,-1.)) ;
#78707=DIRECTION('center_axis',(-4.93038065763132E-32,0.,1.)) ;
#78708=DIRECTION('ref_axis',(1.,0.,0.)) ;
#78709=DIRECTION('center_axis',(0.,-1.,0.)) ;
#78710=DIRECTION('ref_axis',(0.,0.,1.)) ;
#78711=DIRECTION('center_axis',(-4.93038065763132E-32,0.,1.)) ;
#78712=DIRECTION('ref_axis',(1.,0.,0.)) ;
#78713=DIRECTION('center_axis',(-4.93038065763132E-32,0.,1.)) ;
#78714=DIRECTION('ref_axis',(1.,0.,4.93038065763132E-32)) ;
#78715=DIRECTION('center_axis',(-4.93038065763132E-32,0.,1.)) ;
#78716=DIRECTION('ref_axis',(1.,0.,0.)) ;
#78717=DIRECTION('center_axis',(-4.93038065763132E-32,0.,1.)) ;
#78718=DIRECTION('ref_axis',(1.,0.,4.93038065763132E-32)) ;
#78719=DIRECTION('center_axis',(-4.93038065763132E-32,0.,1.)) ;
#78720=DIRECTION('ref_axis',(1.,0.,0.)) ;
#78721=DIRECTION('center_axis',(0.,-1.,0.)) ;
#78722=DIRECTION('ref_axis',(0.,0.,1.)) ;
#78723=DIRECTION('center_axis',(0.,-1.,0.)) ;
#78724=DIRECTION('ref_axis',(0.,0.,-1.)) ;
#78725=DIRECTION('center_axis',(0.,-1.,0.)) ;
#78726=DIRECTION('ref_axis',(0.,0.,-1.)) ;
#78727=DIRECTION('center_axis',(0.,0.,-1.)) ;
#78728=DIRECTION('ref_axis',(-1.,0.,0.)) ;
#78729=DIRECTION('center_axis',(-4.93038065763132E-32,0.,1.)) ;
#78730=DIRECTION('ref_axis',(1.,0.,4.93038065763132E-32)) ;
#78731=DIRECTION('center_axis',(0.,0.,-1.)) ;
#78732=DIRECTION('ref_axis',(-1.,0.,0.)) ;
#78733=DIRECTION('center_axis',(-4.93038065763132E-32,0.,1.)) ;
#78734=DIRECTION('ref_axis',(1.,0.,4.93038065763132E-32)) ;
#78735=DIRECTION('center_axis',(0.,1.,0.)) ;
#78736=DIRECTION('ref_axis',(0.,0.,1.)) ;
#78737=DIRECTION('center_axis',(0.,-1.,0.)) ;
#78738=DIRECTION('ref_axis',(0.,0.,-1.)) ;
#78739=DIRECTION('center_axis',(-4.93038065763132E-32,0.,1.)) ;
#78740=DIRECTION('ref_axis',(1.,0.,0.)) ;
#78741=DIRECTION('center_axis',(-1.,0.,0.)) ;
#78742=DIRECTION('ref_axis',(0.,0.,-1.)) ;
#78743=DIRECTION('center_axis',(-4.93038065763132E-32,0.,1.)) ;
#78744=DIRECTION('ref_axis',(1.,0.,0.)) ;
#78745=DIRECTION('center_axis',(1.,0.,0.)) ;
#78746=DIRECTION('ref_axis',(0.,0.,1.)) ;
#78747=DIRECTION('center_axis',(-1.,0.,-4.93038065763132E-32)) ;
#78748=DIRECTION('ref_axis',(-4.93038065763132E-32,0.,1.)) ;
#78749=DIRECTION('center_axis',(1.,0.,4.93038065763132E-32)) ;
#78750=DIRECTION('ref_axis',(4.93038065763132E-32,0.,-1.)) ;
#78751=DIRECTION('center_axis',(1.,0.,0.)) ;
#78752=DIRECTION('ref_axis',(0.,0.,-1.)) ;
#78753=DIRECTION('center_axis',(-1.,0.,0.)) ;
#78754=DIRECTION('ref_axis',(0.,0.,1.)) ;
#78755=DIRECTION('center_axis',(-4.93038065763132E-32,0.,1.)) ;
#78756=DIRECTION('ref_axis',(1.,0.,0.)) ;
#78757=DIRECTION('center_axis',(-4.93038065763132E-32,0.,1.)) ;
#78758=DIRECTION('ref_axis',(1.,0.,4.93038065763132E-32)) ;
#78759=DIRECTION('center_axis',(0.,-1.,0.)) ;
#78760=DIRECTION('ref_axis',(0.,0.,1.)) ;
#78761=DIRECTION('center_axis',(-4.93038065763132E-32,0.,1.)) ;
#78762=DIRECTION('ref_axis',(1.,0.,0.)) ;
#78763=DIRECTION('center_axis',(0.,-1.,0.)) ;
#78764=DIRECTION('ref_axis',(0.,0.,1.)) ;
#78765=DIRECTION('center_axis',(-4.93038065763132E-32,0.,1.)) ;
#78766=DIRECTION('ref_axis',(1.,0.,4.93038065763132E-32)) ;
#78767=DIRECTION('center_axis',(0.,0.,-1.)) ;
#78768=DIRECTION('ref_axis',(-1.,0.,0.)) ;
#78769=DIRECTION('center_axis',(-4.93038065763132E-32,0.,1.)) ;
#78770=DIRECTION('ref_axis',(1.,0.,4.93038065763132E-32)) ;
#78771=DIRECTION('center_axis',(0.,-1.,0.)) ;
#78772=DIRECTION('ref_axis',(0.,0.,-1.)) ;
#78773=DIRECTION('center_axis',(0.,-1.,0.)) ;
#78774=DIRECTION('ref_axis',(0.,0.,-1.)) ;
#78775=DIRECTION('center_axis',(-1.,0.,-4.93038065763132E-32)) ;
#78776=DIRECTION('ref_axis',(-4.93038065763132E-32,0.,1.)) ;
#78777=DIRECTION('center_axis',(-1.,0.,0.)) ;
#78778=DIRECTION('ref_axis',(0.,0.,1.)) ;
#78779=DIRECTION('center_axis',(1.,0.,0.)) ;
#78780=DIRECTION('ref_axis',(0.,0.,-1.)) ;
#78781=DIRECTION('center_axis',(0.,1.,0.)) ;
#78782=DIRECTION('ref_axis',(0.,0.,1.)) ;
#78783=DIRECTION('center_axis',(0.,-1.,0.)) ;
#78784=DIRECTION('ref_axis',(0.,0.,-1.)) ;
#78785=DIRECTION('center_axis',(0.,0.,-1.)) ;
#78786=DIRECTION('ref_axis',(-1.,0.,0.)) ;
#78787=DIRECTION('center_axis',(-4.93038065763132E-32,0.,1.)) ;
#78788=DIRECTION('ref_axis',(1.,0.,4.93038065763132E-32)) ;
#78789=DIRECTION('center_axis',(1.,0.,4.93038065763132E-32)) ;
#78790=DIRECTION('ref_axis',(4.93038065763132E-32,0.,-1.)) ;
#78791=DIRECTION('center_axis',(-1.,0.,0.)) ;
#78792=DIRECTION('ref_axis',(0.,0.,1.)) ;
#78793=DIRECTION('center_axis',(1.,0.,0.)) ;
#78794=DIRECTION('ref_axis',(0.,0.,-1.)) ;
#78795=DIRECTION('center_axis',(-4.93038065763132E-32,0.,1.)) ;
#78796=DIRECTION('ref_axis',(1.,0.,0.)) ;
#78797=DIRECTION('center_axis',(0.,-1.,0.)) ;
#78798=DIRECTION('ref_axis',(0.,0.,1.)) ;
#78799=DIRECTION('center_axis',(-4.93038065763132E-32,0.,1.)) ;
#78800=DIRECTION('ref_axis',(1.,0.,0.)) ;
#78801=DIRECTION('center_axis',(-4.93038065763132E-32,0.,1.)) ;
#78802=DIRECTION('ref_axis',(1.,0.,4.93038065763132E-32)) ;
#78803=DIRECTION('center_axis',(-4.93038065763132E-32,0.,1.)) ;
#78804=DIRECTION('ref_axis',(1.,0.,0.)) ;
#78805=DIRECTION('center_axis',(-4.93038065763132E-32,0.,1.)) ;
#78806=DIRECTION('ref_axis',(1.,0.,4.93038065763132E-32)) ;
#78807=DIRECTION('center_axis',(-4.93038065763132E-32,0.,1.)) ;
#78808=DIRECTION('ref_axis',(1.,0.,0.)) ;
#78809=DIRECTION('center_axis',(0.,-1.,0.)) ;
#78810=DIRECTION('ref_axis',(0.,0.,1.)) ;
#78811=DIRECTION('center_axis',(0.,-1.,0.)) ;
#78812=DIRECTION('ref_axis',(0.,0.,-1.)) ;
#78813=DIRECTION('center_axis',(0.,-1.,0.)) ;
#78814=DIRECTION('ref_axis',(0.,0.,-1.)) ;
#78815=DIRECTION('center_axis',(0.,0.,-1.)) ;
#78816=DIRECTION('ref_axis',(-1.,0.,0.)) ;
#78817=DIRECTION('center_axis',(-4.93038065763132E-32,0.,1.)) ;
#78818=DIRECTION('ref_axis',(1.,0.,4.93038065763132E-32)) ;
#78819=DIRECTION('center_axis',(0.,0.,-1.)) ;
#78820=DIRECTION('ref_axis',(-1.,0.,0.)) ;
#78821=DIRECTION('center_axis',(-4.93038065763132E-32,0.,1.)) ;
#78822=DIRECTION('ref_axis',(1.,0.,4.93038065763132E-32)) ;
#78823=DIRECTION('center_axis',(0.,1.,0.)) ;
#78824=DIRECTION('ref_axis',(0.,0.,1.)) ;
#78825=DIRECTION('center_axis',(0.,-1.,0.)) ;
#78826=DIRECTION('ref_axis',(0.,0.,-1.)) ;
#78827=DIRECTION('center_axis',(-4.93038065763132E-32,0.,1.)) ;
#78828=DIRECTION('ref_axis',(1.,0.,0.)) ;
#78829=DIRECTION('center_axis',(-1.,0.,0.)) ;
#78830=DIRECTION('ref_axis',(0.,0.,-1.)) ;
#78831=DIRECTION('center_axis',(-4.93038065763132E-32,0.,1.)) ;
#78832=DIRECTION('ref_axis',(1.,0.,0.)) ;
#78833=DIRECTION('center_axis',(1.,0.,0.)) ;
#78834=DIRECTION('ref_axis',(0.,0.,1.)) ;
#78835=DIRECTION('center_axis',(-1.,0.,-4.93038065763132E-32)) ;
#78836=DIRECTION('ref_axis',(-4.93038065763132E-32,0.,1.)) ;
#78837=DIRECTION('center_axis',(1.,0.,4.93038065763132E-32)) ;
#78838=DIRECTION('ref_axis',(4.93038065763132E-32,0.,-1.)) ;
#78839=DIRECTION('center_axis',(1.,0.,0.)) ;
#78840=DIRECTION('ref_axis',(0.,0.,-1.)) ;
#78841=DIRECTION('center_axis',(-1.,0.,0.)) ;
#78842=DIRECTION('ref_axis',(0.,0.,1.)) ;
#78843=DIRECTION('center_axis',(-4.93038065763132E-32,0.,1.)) ;
#78844=DIRECTION('ref_axis',(1.,0.,0.)) ;
#78845=DIRECTION('center_axis',(-4.93038065763132E-32,0.,1.)) ;
#78846=DIRECTION('ref_axis',(1.,0.,4.93038065763132E-32)) ;
#78847=DIRECTION('center_axis',(0.,-1.,0.)) ;
#78848=DIRECTION('ref_axis',(0.,0.,1.)) ;
#78849=DIRECTION('center_axis',(-4.93038065763132E-32,0.,1.)) ;
#78850=DIRECTION('ref_axis',(1.,0.,0.)) ;
#78851=DIRECTION('center_axis',(0.,-1.,0.)) ;
#78852=DIRECTION('ref_axis',(0.,0.,1.)) ;
#78853=DIRECTION('center_axis',(-4.93038065763132E-32,0.,1.)) ;
#78854=DIRECTION('ref_axis',(1.,0.,4.93038065763132E-32)) ;
#78855=DIRECTION('center_axis',(0.,0.,-1.)) ;
#78856=DIRECTION('ref_axis',(-1.,0.,0.)) ;
#78857=DIRECTION('center_axis',(-4.93038065763132E-32,0.,1.)) ;
#78858=DIRECTION('ref_axis',(1.,0.,4.93038065763132E-32)) ;
#78859=DIRECTION('center_axis',(6.93889390390723E-16,-1.,3.42113882891801E-47)) ;
#78860=DIRECTION('ref_axis',(1.,6.93889390390723E-16,-2.37389193643995E-62)) ;
#78861=DIRECTION('center_axis',(0.,-1.,0.)) ;
#78862=DIRECTION('ref_axis',(0.,0.,-1.)) ;
#78863=DIRECTION('center_axis',(-1.,0.,-4.93038065763132E-32)) ;
#78864=DIRECTION('ref_axis',(-4.93038065763132E-32,0.,1.)) ;
#78865=DIRECTION('center_axis',(-1.,0.,0.)) ;
#78866=DIRECTION('ref_axis',(0.,0.,1.)) ;
#78867=DIRECTION('center_axis',(1.,0.,0.)) ;
#78868=DIRECTION('ref_axis',(0.,0.,-1.)) ;
#78869=DIRECTION('center_axis',(0.,1.,0.)) ;
#78870=DIRECTION('ref_axis',(0.,0.,1.)) ;
#78871=DIRECTION('center_axis',(0.,-1.,0.)) ;
#78872=DIRECTION('ref_axis',(0.,0.,-1.)) ;
#78873=DIRECTION('center_axis',(0.,0.,-1.)) ;
#78874=DIRECTION('ref_axis',(-1.,0.,0.)) ;
#78875=DIRECTION('center_axis',(-4.93038065763132E-32,0.,1.)) ;
#78876=DIRECTION('ref_axis',(1.,0.,4.93038065763132E-32)) ;
#78877=DIRECTION('center_axis',(1.,0.,4.93038065763132E-32)) ;
#78878=DIRECTION('ref_axis',(4.93038065763132E-32,0.,-1.)) ;
#78879=DIRECTION('center_axis',(-1.,0.,0.)) ;
#78880=DIRECTION('ref_axis',(0.,0.,1.)) ;
#78881=DIRECTION('center_axis',(1.,0.,0.)) ;
#78882=DIRECTION('ref_axis',(0.,0.,-1.)) ;
#78883=DIRECTION('center_axis',(-4.93038065763132E-32,0.,1.)) ;
#78884=DIRECTION('ref_axis',(1.,0.,0.)) ;
#78885=DIRECTION('center_axis',(0.,-1.,0.)) ;
#78886=DIRECTION('ref_axis',(0.,0.,1.)) ;
#78887=DIRECTION('center_axis',(-4.93038065763132E-32,0.,1.)) ;
#78888=DIRECTION('ref_axis',(1.,0.,0.)) ;
#78889=DIRECTION('center_axis',(-4.93038065763132E-32,0.,1.)) ;
#78890=DIRECTION('ref_axis',(1.,0.,4.93038065763132E-32)) ;
#78891=DIRECTION('center_axis',(-4.93038065763132E-32,0.,1.)) ;
#78892=DIRECTION('ref_axis',(1.,0.,0.)) ;
#78893=DIRECTION('center_axis',(-4.93038065763132E-32,0.,1.)) ;
#78894=DIRECTION('ref_axis',(1.,0.,4.93038065763132E-32)) ;
#78895=DIRECTION('center_axis',(-4.93038065763132E-32,0.,1.)) ;
#78896=DIRECTION('ref_axis',(1.,0.,0.)) ;
#78897=DIRECTION('center_axis',(0.,-1.,0.)) ;
#78898=DIRECTION('ref_axis',(0.,0.,1.)) ;
#78899=DIRECTION('center_axis',(6.93889390390723E-16,-1.,3.42113882891801E-47)) ;
#78900=DIRECTION('ref_axis',(1.,6.93889390390723E-16,-2.37389193643995E-62)) ;
#78901=DIRECTION('center_axis',(0.,-1.,0.)) ;
#78902=DIRECTION('ref_axis',(0.,0.,-1.)) ;
#78903=DIRECTION('center_axis',(0.,0.,-1.)) ;
#78904=DIRECTION('ref_axis',(-1.,0.,0.)) ;
#78905=DIRECTION('center_axis',(-4.93038065763132E-32,0.,1.)) ;
#78906=DIRECTION('ref_axis',(1.,0.,4.93038065763132E-32)) ;
#78907=DIRECTION('center_axis',(0.,0.,-1.)) ;
#78908=DIRECTION('ref_axis',(-1.,0.,0.)) ;
#78909=DIRECTION('center_axis',(-4.93038065763132E-32,0.,1.)) ;
#78910=DIRECTION('ref_axis',(1.,0.,4.93038065763132E-32)) ;
#78911=DIRECTION('center_axis',(0.,1.,0.)) ;
#78912=DIRECTION('ref_axis',(0.,0.,1.)) ;
#78913=DIRECTION('center_axis',(0.,-1.,0.)) ;
#78914=DIRECTION('ref_axis',(0.,0.,-1.)) ;
#78915=DIRECTION('center_axis',(-4.93038065763132E-32,0.,1.)) ;
#78916=DIRECTION('ref_axis',(1.,0.,0.)) ;
#78917=DIRECTION('center_axis',(-1.,0.,0.)) ;
#78918=DIRECTION('ref_axis',(0.,0.,-1.)) ;
#78919=DIRECTION('center_axis',(-4.93038065763132E-32,0.,1.)) ;
#78920=DIRECTION('ref_axis',(1.,0.,0.)) ;
#78921=DIRECTION('center_axis',(1.,0.,0.)) ;
#78922=DIRECTION('ref_axis',(0.,0.,1.)) ;
#78923=DIRECTION('center_axis',(-1.,0.,-4.93038065763132E-32)) ;
#78924=DIRECTION('ref_axis',(-4.93038065763132E-32,0.,1.)) ;
#78925=DIRECTION('center_axis',(1.,0.,4.93038065763132E-32)) ;
#78926=DIRECTION('ref_axis',(4.93038065763132E-32,0.,-1.)) ;
#78927=DIRECTION('center_axis',(1.,0.,0.)) ;
#78928=DIRECTION('ref_axis',(0.,0.,-1.)) ;
#78929=DIRECTION('center_axis',(-1.,0.,0.)) ;
#78930=DIRECTION('ref_axis',(0.,0.,1.)) ;
#78931=DIRECTION('center_axis',(-4.93038065763132E-32,0.,1.)) ;
#78932=DIRECTION('ref_axis',(1.,0.,0.)) ;
#78933=DIRECTION('center_axis',(-4.93038065763132E-32,0.,1.)) ;
#78934=DIRECTION('ref_axis',(1.,0.,4.93038065763132E-32)) ;
#78935=DIRECTION('center_axis',(0.,-1.,0.)) ;
#78936=DIRECTION('ref_axis',(0.,0.,1.)) ;
#78937=DIRECTION('center_axis',(-4.93038065763132E-32,0.,1.)) ;
#78938=DIRECTION('ref_axis',(1.,0.,0.)) ;
#78939=DIRECTION('center_axis',(0.,-1.,0.)) ;
#78940=DIRECTION('ref_axis',(0.,0.,1.)) ;
#78941=DIRECTION('center_axis',(-4.93038065763132E-32,0.,1.)) ;
#78942=DIRECTION('ref_axis',(1.,0.,4.93038065763132E-32)) ;
#78943=DIRECTION('center_axis',(0.,0.,-1.)) ;
#78944=DIRECTION('ref_axis',(-1.,0.,0.)) ;
#78945=DIRECTION('center_axis',(-4.93038065763132E-32,0.,1.)) ;
#78946=DIRECTION('ref_axis',(1.,0.,4.93038065763132E-32)) ;
#78947=DIRECTION('center_axis',(3.46944695195361E-16,-1.,1.71056941445901E-47)) ;
#78948=DIRECTION('ref_axis',(1.,3.46944695195361E-16,-5.93472984109987E-63)) ;
#78949=DIRECTION('center_axis',(0.,-1.,0.)) ;
#78950=DIRECTION('ref_axis',(0.,0.,-1.)) ;
#78951=DIRECTION('center_axis',(-1.,0.,-4.93038065763132E-32)) ;
#78952=DIRECTION('ref_axis',(-4.93038065763132E-32,0.,1.)) ;
#78953=DIRECTION('center_axis',(-1.,0.,0.)) ;
#78954=DIRECTION('ref_axis',(0.,0.,1.)) ;
#78955=DIRECTION('center_axis',(1.,0.,0.)) ;
#78956=DIRECTION('ref_axis',(0.,0.,-1.)) ;
#78957=DIRECTION('center_axis',(0.,1.,0.)) ;
#78958=DIRECTION('ref_axis',(0.,0.,1.)) ;
#78959=DIRECTION('center_axis',(0.,-1.,0.)) ;
#78960=DIRECTION('ref_axis',(0.,0.,-1.)) ;
#78961=DIRECTION('center_axis',(0.,0.,-1.)) ;
#78962=DIRECTION('ref_axis',(-1.,0.,0.)) ;
#78963=DIRECTION('center_axis',(-4.93038065763132E-32,0.,1.)) ;
#78964=DIRECTION('ref_axis',(1.,0.,4.93038065763132E-32)) ;
#78965=DIRECTION('center_axis',(1.,0.,4.93038065763132E-32)) ;
#78966=DIRECTION('ref_axis',(4.93038065763132E-32,0.,-1.)) ;
#78967=DIRECTION('center_axis',(-1.,0.,0.)) ;
#78968=DIRECTION('ref_axis',(0.,0.,1.)) ;
#78969=DIRECTION('center_axis',(1.,0.,0.)) ;
#78970=DIRECTION('ref_axis',(0.,0.,-1.)) ;
#78971=DIRECTION('center_axis',(-4.93038065763132E-32,0.,1.)) ;
#78972=DIRECTION('ref_axis',(1.,0.,0.)) ;
#78973=DIRECTION('center_axis',(0.,-1.,0.)) ;
#78974=DIRECTION('ref_axis',(0.,0.,1.)) ;
#78975=DIRECTION('center_axis',(-4.93038065763132E-32,0.,1.)) ;
#78976=DIRECTION('ref_axis',(1.,0.,0.)) ;
#78977=DIRECTION('center_axis',(-4.93038065763132E-32,0.,1.)) ;
#78978=DIRECTION('ref_axis',(1.,0.,4.93038065763132E-32)) ;
#78979=DIRECTION('center_axis',(-4.93038065763132E-32,0.,1.)) ;
#78980=DIRECTION('ref_axis',(1.,0.,0.)) ;
#78981=DIRECTION('center_axis',(-4.93038065763132E-32,0.,1.)) ;
#78982=DIRECTION('ref_axis',(1.,0.,4.93038065763132E-32)) ;
#78983=DIRECTION('center_axis',(-4.93038065763132E-32,0.,1.)) ;
#78984=DIRECTION('ref_axis',(1.,0.,0.)) ;
#78985=DIRECTION('center_axis',(0.,-1.,0.)) ;
#78986=DIRECTION('ref_axis',(0.,0.,1.)) ;
#78987=DIRECTION('center_axis',(3.46944695195361E-16,-1.,1.71056941445901E-47)) ;
#78988=DIRECTION('ref_axis',(1.,3.46944695195361E-16,-5.93472984109987E-63)) ;
#78989=DIRECTION('center_axis',(0.,-1.,0.)) ;
#78990=DIRECTION('ref_axis',(0.,0.,-1.)) ;
#78991=DIRECTION('center_axis',(0.,0.,-1.)) ;
#78992=DIRECTION('ref_axis',(-1.,0.,0.)) ;
#78993=DIRECTION('center_axis',(-4.93038065763132E-32,0.,1.)) ;
#78994=DIRECTION('ref_axis',(1.,0.,4.93038065763132E-32)) ;
#78995=DIRECTION('center_axis',(0.,0.,-1.)) ;
#78996=DIRECTION('ref_axis',(-1.,0.,0.)) ;
#78997=DIRECTION('center_axis',(-4.93038065763132E-32,0.,1.)) ;
#78998=DIRECTION('ref_axis',(1.,0.,4.93038065763132E-32)) ;
#78999=DIRECTION('center_axis',(0.,1.,0.)) ;
#79000=DIRECTION('ref_axis',(0.,0.,1.)) ;
#79001=DIRECTION('center_axis',(0.,-1.,0.)) ;
#79002=DIRECTION('ref_axis',(0.,0.,-1.)) ;
#79003=DIRECTION('center_axis',(-4.93038065763132E-32,0.,1.)) ;
#79004=DIRECTION('ref_axis',(1.,0.,0.)) ;
#79005=DIRECTION('center_axis',(-1.,0.,0.)) ;
#79006=DIRECTION('ref_axis',(0.,0.,-1.)) ;
#79007=DIRECTION('center_axis',(-4.93038065763132E-32,0.,1.)) ;
#79008=DIRECTION('ref_axis',(1.,0.,0.)) ;
#79009=DIRECTION('center_axis',(1.,0.,0.)) ;
#79010=DIRECTION('ref_axis',(0.,0.,1.)) ;
#79011=DIRECTION('center_axis',(-1.,0.,-4.93038065763132E-32)) ;
#79012=DIRECTION('ref_axis',(-4.93038065763132E-32,0.,1.)) ;
#79013=DIRECTION('center_axis',(1.,0.,4.93038065763132E-32)) ;
#79014=DIRECTION('ref_axis',(4.93038065763132E-32,0.,-1.)) ;
#79015=DIRECTION('center_axis',(1.,0.,0.)) ;
#79016=DIRECTION('ref_axis',(0.,0.,-1.)) ;
#79017=DIRECTION('center_axis',(-1.,0.,0.)) ;
#79018=DIRECTION('ref_axis',(0.,0.,1.)) ;
#79019=DIRECTION('center_axis',(-4.93038065763132E-32,0.,1.)) ;
#79020=DIRECTION('ref_axis',(1.,0.,0.)) ;
#79021=DIRECTION('center_axis',(-4.93038065763132E-32,0.,1.)) ;
#79022=DIRECTION('ref_axis',(1.,0.,4.93038065763132E-32)) ;
#79023=DIRECTION('center_axis',(0.,-1.,0.)) ;
#79024=DIRECTION('ref_axis',(0.,0.,1.)) ;
#79025=DIRECTION('center_axis',(-4.93038065763132E-32,0.,1.)) ;
#79026=DIRECTION('ref_axis',(1.,0.,0.)) ;
#79027=DIRECTION('center_axis',(0.,-1.,0.)) ;
#79028=DIRECTION('ref_axis',(0.,0.,1.)) ;
#79029=DIRECTION('center_axis',(-4.93038065763132E-32,0.,1.)) ;
#79030=DIRECTION('ref_axis',(1.,0.,4.93038065763132E-32)) ;
#79031=DIRECTION('center_axis',(0.,0.,-1.)) ;
#79032=DIRECTION('ref_axis',(-1.,0.,0.)) ;
#79033=DIRECTION('center_axis',(-4.93038065763132E-32,0.,1.)) ;
#79034=DIRECTION('ref_axis',(1.,0.,4.93038065763132E-32)) ;
#79035=DIRECTION('center_axis',(0.,-1.,0.)) ;
#79036=DIRECTION('ref_axis',(0.,0.,-1.)) ;
#79037=DIRECTION('center_axis',(0.,-1.,0.)) ;
#79038=DIRECTION('ref_axis',(0.,0.,-1.)) ;
#79039=DIRECTION('center_axis',(-1.,0.,-4.93038065763132E-32)) ;
#79040=DIRECTION('ref_axis',(-4.93038065763132E-32,0.,1.)) ;
#79041=DIRECTION('center_axis',(-1.,0.,0.)) ;
#79042=DIRECTION('ref_axis',(0.,0.,1.)) ;
#79043=DIRECTION('center_axis',(1.,0.,0.)) ;
#79044=DIRECTION('ref_axis',(0.,0.,-1.)) ;
#79045=DIRECTION('center_axis',(-3.46944695195361E-16,1.,-1.71056941445901E-47)) ;
#79046=DIRECTION('ref_axis',(-1.,-3.46944695195361E-16,5.93472984109987E-63)) ;
#79047=DIRECTION('center_axis',(0.,-1.,0.)) ;
#79048=DIRECTION('ref_axis',(0.,0.,-1.)) ;
#79049=DIRECTION('center_axis',(0.,0.,-1.)) ;
#79050=DIRECTION('ref_axis',(-1.,0.,0.)) ;
#79051=DIRECTION('center_axis',(-4.93038065763132E-32,0.,1.)) ;
#79052=DIRECTION('ref_axis',(1.,0.,4.93038065763132E-32)) ;
#79053=DIRECTION('center_axis',(1.,0.,4.93038065763132E-32)) ;
#79054=DIRECTION('ref_axis',(4.93038065763132E-32,0.,-1.)) ;
#79055=DIRECTION('center_axis',(-1.,0.,0.)) ;
#79056=DIRECTION('ref_axis',(0.,0.,1.)) ;
#79057=DIRECTION('center_axis',(1.,0.,0.)) ;
#79058=DIRECTION('ref_axis',(0.,0.,-1.)) ;
#79059=DIRECTION('center_axis',(-4.93038065763132E-32,0.,1.)) ;
#79060=DIRECTION('ref_axis',(1.,0.,0.)) ;
#79061=DIRECTION('center_axis',(0.,-1.,0.)) ;
#79062=DIRECTION('ref_axis',(0.,0.,1.)) ;
#79063=DIRECTION('center_axis',(-4.93038065763132E-32,0.,1.)) ;
#79064=DIRECTION('ref_axis',(1.,0.,0.)) ;
#79065=DIRECTION('center_axis',(-4.93038065763132E-32,0.,1.)) ;
#79066=DIRECTION('ref_axis',(1.,0.,4.93038065763132E-32)) ;
#79067=DIRECTION('center_axis',(-4.93038065763132E-32,0.,1.)) ;
#79068=DIRECTION('ref_axis',(1.,0.,0.)) ;
#79069=DIRECTION('center_axis',(-4.93038065763132E-32,0.,1.)) ;
#79070=DIRECTION('ref_axis',(1.,0.,4.93038065763132E-32)) ;
#79071=DIRECTION('center_axis',(-4.93038065763132E-32,0.,1.)) ;
#79072=DIRECTION('ref_axis',(1.,0.,0.)) ;
#79073=DIRECTION('center_axis',(0.,-1.,0.)) ;
#79074=DIRECTION('ref_axis',(0.,0.,1.)) ;
#79075=DIRECTION('center_axis',(0.,-1.,0.)) ;
#79076=DIRECTION('ref_axis',(0.,0.,-1.)) ;
#79077=DIRECTION('center_axis',(0.,-1.,0.)) ;
#79078=DIRECTION('ref_axis',(0.,0.,-1.)) ;
#79079=DIRECTION('center_axis',(0.,0.,-1.)) ;
#79080=DIRECTION('ref_axis',(-1.,0.,0.)) ;
#79081=DIRECTION('center_axis',(-4.93038065763132E-32,0.,1.)) ;
#79082=DIRECTION('ref_axis',(1.,0.,4.93038065763132E-32)) ;
#79083=DIRECTION('center_axis',(0.,0.,-1.)) ;
#79084=DIRECTION('ref_axis',(-1.,0.,0.)) ;
#79085=DIRECTION('center_axis',(-4.93038065763132E-32,0.,1.)) ;
#79086=DIRECTION('ref_axis',(1.,0.,4.93038065763132E-32)) ;
#79087=DIRECTION('center_axis',(-3.46944695195361E-16,1.,-1.71056941445901E-47)) ;
#79088=DIRECTION('ref_axis',(-1.,-3.46944695195361E-16,5.93472984109987E-63)) ;
#79089=DIRECTION('center_axis',(0.,-1.,0.)) ;
#79090=DIRECTION('ref_axis',(0.,0.,-1.)) ;
#79091=DIRECTION('center_axis',(-4.93038065763132E-32,0.,1.)) ;
#79092=DIRECTION('ref_axis',(1.,0.,0.)) ;
#79093=DIRECTION('center_axis',(-1.,0.,0.)) ;
#79094=DIRECTION('ref_axis',(0.,0.,-1.)) ;
#79095=DIRECTION('center_axis',(-4.93038065763132E-32,0.,1.)) ;
#79096=DIRECTION('ref_axis',(1.,0.,0.)) ;
#79097=DIRECTION('center_axis',(1.,0.,0.)) ;
#79098=DIRECTION('ref_axis',(0.,0.,1.)) ;
#79099=DIRECTION('center_axis',(-1.,0.,-4.93038065763132E-32)) ;
#79100=DIRECTION('ref_axis',(-4.93038065763132E-32,0.,1.)) ;
#79101=DIRECTION('center_axis',(-1.,0.,-4.93038065763132E-32)) ;
#79102=DIRECTION('ref_axis',(-4.93038065763132E-32,0.,1.)) ;
#79103=DIRECTION('center_axis',(-1.,0.,0.)) ;
#79104=DIRECTION('ref_axis',(0.,0.,1.)) ;
#79105=DIRECTION('center_axis',(1.,0.,0.)) ;
#79106=DIRECTION('ref_axis',(0.,0.,-1.)) ;
#79107=DIRECTION('center_axis',(-4.93038065763132E-32,0.,1.)) ;
#79108=DIRECTION('ref_axis',(1.,0.,0.)) ;
#79109=DIRECTION('center_axis',(-4.93038065763132E-32,0.,1.)) ;
#79110=DIRECTION('ref_axis',(1.,0.,4.93038065763132E-32)) ;
#79111=DIRECTION('center_axis',(0.,1.,0.)) ;
#79112=DIRECTION('ref_axis',(0.,0.,-1.)) ;
#79113=DIRECTION('center_axis',(-4.93038065763132E-32,0.,1.)) ;
#79114=DIRECTION('ref_axis',(1.,0.,0.)) ;
#79115=DIRECTION('center_axis',(0.,1.,0.)) ;
#79116=DIRECTION('ref_axis',(0.,0.,-1.)) ;
#79117=DIRECTION('center_axis',(-4.93038065763132E-32,0.,1.)) ;
#79118=DIRECTION('ref_axis',(1.,0.,4.93038065763132E-32)) ;
#79119=DIRECTION('center_axis',(0.,0.,-1.)) ;
#79120=DIRECTION('ref_axis',(-1.,0.,0.)) ;
#79121=DIRECTION('center_axis',(-4.93038065763132E-32,0.,1.)) ;
#79122=DIRECTION('ref_axis',(1.,0.,4.93038065763132E-32)) ;
#79123=DIRECTION('center_axis',(-3.46944695195361E-16,1.,-1.71056941445901E-47)) ;
#79124=DIRECTION('ref_axis',(-1.,-3.46944695195361E-16,5.93472984109987E-63)) ;
#79125=DIRECTION('center_axis',(0.,1.,0.)) ;
#79126=DIRECTION('ref_axis',(0.,0.,1.)) ;
#79127=DIRECTION('center_axis',(1.,0.,4.93038065763132E-32)) ;
#79128=DIRECTION('ref_axis',(4.93038065763132E-32,0.,-1.)) ;
#79129=DIRECTION('center_axis',(1.,0.,0.)) ;
#79130=DIRECTION('ref_axis',(0.,0.,-1.)) ;
#79131=DIRECTION('center_axis',(-1.,0.,0.)) ;
#79132=DIRECTION('ref_axis',(0.,0.,1.)) ;
#79133=DIRECTION('center_axis',(0.,-1.,0.)) ;
#79134=DIRECTION('ref_axis',(0.,0.,-1.)) ;
#79135=DIRECTION('center_axis',(0.,1.,0.)) ;
#79136=DIRECTION('ref_axis',(0.,0.,1.)) ;
#79137=DIRECTION('center_axis',(0.,0.,-1.)) ;
#79138=DIRECTION('ref_axis',(-1.,0.,0.)) ;
#79139=DIRECTION('center_axis',(-4.93038065763132E-32,0.,1.)) ;
#79140=DIRECTION('ref_axis',(1.,0.,4.93038065763132E-32)) ;
#79141=DIRECTION('center_axis',(-1.,0.,-4.93038065763132E-32)) ;
#79142=DIRECTION('ref_axis',(-4.93038065763132E-32,0.,1.)) ;
#79143=DIRECTION('center_axis',(1.,0.,0.)) ;
#79144=DIRECTION('ref_axis',(0.,0.,-1.)) ;
#79145=DIRECTION('center_axis',(-1.,0.,0.)) ;
#79146=DIRECTION('ref_axis',(0.,0.,1.)) ;
#79147=DIRECTION('center_axis',(-4.93038065763132E-32,0.,1.)) ;
#79148=DIRECTION('ref_axis',(1.,0.,0.)) ;
#79149=DIRECTION('center_axis',(0.,1.,0.)) ;
#79150=DIRECTION('ref_axis',(0.,0.,-1.)) ;
#79151=DIRECTION('center_axis',(-4.93038065763132E-32,0.,1.)) ;
#79152=DIRECTION('ref_axis',(1.,0.,0.)) ;
#79153=DIRECTION('center_axis',(-4.93038065763132E-32,0.,1.)) ;
#79154=DIRECTION('ref_axis',(1.,0.,4.93038065763132E-32)) ;
#79155=DIRECTION('center_axis',(-4.93038065763132E-32,0.,1.)) ;
#79156=DIRECTION('ref_axis',(1.,0.,0.)) ;
#79157=DIRECTION('center_axis',(-4.93038065763132E-32,0.,1.)) ;
#79158=DIRECTION('ref_axis',(1.,0.,4.93038065763132E-32)) ;
#79159=DIRECTION('center_axis',(-4.93038065763132E-32,0.,1.)) ;
#79160=DIRECTION('ref_axis',(1.,0.,0.)) ;
#79161=DIRECTION('center_axis',(0.,1.,0.)) ;
#79162=DIRECTION('ref_axis',(0.,0.,-1.)) ;
#79163=DIRECTION('center_axis',(-3.46944695195361E-16,1.,-1.71056941445901E-47)) ;
#79164=DIRECTION('ref_axis',(-1.,-3.46944695195361E-16,5.93472984109987E-63)) ;
#79165=DIRECTION('center_axis',(0.,1.,0.)) ;
#79166=DIRECTION('ref_axis',(0.,0.,1.)) ;
#79167=DIRECTION('center_axis',(0.,0.,-1.)) ;
#79168=DIRECTION('ref_axis',(-1.,0.,0.)) ;
#79169=DIRECTION('center_axis',(-4.93038065763132E-32,0.,1.)) ;
#79170=DIRECTION('ref_axis',(1.,0.,4.93038065763132E-32)) ;
#79171=DIRECTION('center_axis',(0.,0.,-1.)) ;
#79172=DIRECTION('ref_axis',(-1.,0.,0.)) ;
#79173=DIRECTION('center_axis',(-4.93038065763132E-32,0.,1.)) ;
#79174=DIRECTION('ref_axis',(1.,0.,4.93038065763132E-32)) ;
#79175=DIRECTION('center_axis',(0.,-1.,0.)) ;
#79176=DIRECTION('ref_axis',(0.,0.,-1.)) ;
#79177=DIRECTION('center_axis',(0.,1.,0.)) ;
#79178=DIRECTION('ref_axis',(0.,0.,1.)) ;
#79179=DIRECTION('center_axis',(-4.93038065763132E-32,0.,1.)) ;
#79180=DIRECTION('ref_axis',(1.,0.,0.)) ;
#79181=DIRECTION('center_axis',(1.,0.,0.)) ;
#79182=DIRECTION('ref_axis',(0.,0.,1.)) ;
#79183=DIRECTION('center_axis',(-4.93038065763132E-32,0.,1.)) ;
#79184=DIRECTION('ref_axis',(1.,0.,0.)) ;
#79185=DIRECTION('center_axis',(-1.,0.,0.)) ;
#79186=DIRECTION('ref_axis',(0.,0.,-1.)) ;
#79187=DIRECTION('center_axis',(1.,0.,4.93038065763132E-32)) ;
#79188=DIRECTION('ref_axis',(4.93038065763132E-32,0.,-1.)) ;
#79189=DIRECTION('center_axis',(1.,0.,4.93038065763132E-32)) ;
#79190=DIRECTION('ref_axis',(4.93038065763132E-32,0.,-1.)) ;
#79191=DIRECTION('center_axis',(1.,0.,0.)) ;
#79192=DIRECTION('ref_axis',(0.,0.,-1.)) ;
#79193=DIRECTION('center_axis',(-1.,0.,0.)) ;
#79194=DIRECTION('ref_axis',(0.,0.,1.)) ;
#79195=DIRECTION('center_axis',(-4.93038065763132E-32,0.,1.)) ;
#79196=DIRECTION('ref_axis',(1.,0.,0.)) ;
#79197=DIRECTION('center_axis',(-4.93038065763132E-32,0.,1.)) ;
#79198=DIRECTION('ref_axis',(1.,0.,4.93038065763132E-32)) ;
#79199=DIRECTION('center_axis',(0.,-1.,0.)) ;
#79200=DIRECTION('ref_axis',(0.,0.,1.)) ;
#79201=DIRECTION('center_axis',(-4.93038065763132E-32,0.,1.)) ;
#79202=DIRECTION('ref_axis',(1.,0.,0.)) ;
#79203=DIRECTION('center_axis',(0.,-1.,0.)) ;
#79204=DIRECTION('ref_axis',(0.,0.,1.)) ;
#79205=DIRECTION('center_axis',(-4.93038065763132E-32,0.,1.)) ;
#79206=DIRECTION('ref_axis',(1.,0.,4.93038065763132E-32)) ;
#79207=DIRECTION('center_axis',(0.,0.,-1.)) ;
#79208=DIRECTION('ref_axis',(-1.,0.,0.)) ;
#79209=DIRECTION('center_axis',(-4.93038065763132E-32,0.,1.)) ;
#79210=DIRECTION('ref_axis',(1.,0.,4.93038065763132E-32)) ;
#79211=DIRECTION('center_axis',(1.73472347597681E-16,-1.,8.55284707229503E-48)) ;
#79212=DIRECTION('ref_axis',(1.,1.73472347597681E-16,-1.48368246027497E-63)) ;
#79213=DIRECTION('center_axis',(0.,-1.,0.)) ;
#79214=DIRECTION('ref_axis',(0.,0.,-1.)) ;
#79215=DIRECTION('center_axis',(-1.,0.,-4.93038065763132E-32)) ;
#79216=DIRECTION('ref_axis',(-4.93038065763132E-32,0.,1.)) ;
#79217=DIRECTION('center_axis',(-1.,0.,0.)) ;
#79218=DIRECTION('ref_axis',(0.,0.,1.)) ;
#79219=DIRECTION('center_axis',(1.,0.,0.)) ;
#79220=DIRECTION('ref_axis',(0.,0.,-1.)) ;
#79221=DIRECTION('center_axis',(-2.60208521396521E-16,1.,-1.28292706084425E-47)) ;
#79222=DIRECTION('ref_axis',(-1.,-2.60208521396521E-16,3.33828553561868E-63)) ;
#79223=DIRECTION('center_axis',(0.,-1.,0.)) ;
#79224=DIRECTION('ref_axis',(0.,0.,-1.)) ;
#79225=DIRECTION('center_axis',(0.,0.,-1.)) ;
#79226=DIRECTION('ref_axis',(-1.,0.,0.)) ;
#79227=DIRECTION('center_axis',(-4.93038065763132E-32,0.,1.)) ;
#79228=DIRECTION('ref_axis',(1.,0.,4.93038065763132E-32)) ;
#79229=DIRECTION('center_axis',(1.,0.,4.93038065763132E-32)) ;
#79230=DIRECTION('ref_axis',(4.93038065763132E-32,0.,-1.)) ;
#79231=DIRECTION('center_axis',(-1.,0.,0.)) ;
#79232=DIRECTION('ref_axis',(0.,0.,1.)) ;
#79233=DIRECTION('center_axis',(1.,0.,0.)) ;
#79234=DIRECTION('ref_axis',(0.,0.,-1.)) ;
#79235=DIRECTION('center_axis',(-4.93038065763132E-32,0.,1.)) ;
#79236=DIRECTION('ref_axis',(1.,0.,0.)) ;
#79237=DIRECTION('center_axis',(0.,-1.,0.)) ;
#79238=DIRECTION('ref_axis',(0.,0.,1.)) ;
#79239=DIRECTION('center_axis',(-4.93038065763132E-32,0.,1.)) ;
#79240=DIRECTION('ref_axis',(1.,0.,0.)) ;
#79241=DIRECTION('center_axis',(-4.93038065763132E-32,0.,1.)) ;
#79242=DIRECTION('ref_axis',(1.,0.,4.93038065763132E-32)) ;
#79243=DIRECTION('center_axis',(-4.93038065763132E-32,0.,1.)) ;
#79244=DIRECTION('ref_axis',(1.,0.,0.)) ;
#79245=DIRECTION('center_axis',(-4.93038065763132E-32,0.,1.)) ;
#79246=DIRECTION('ref_axis',(1.,0.,4.93038065763132E-32)) ;
#79247=DIRECTION('center_axis',(-4.93038065763132E-32,0.,1.)) ;
#79248=DIRECTION('ref_axis',(1.,0.,0.)) ;
#79249=DIRECTION('center_axis',(0.,-1.,0.)) ;
#79250=DIRECTION('ref_axis',(0.,0.,1.)) ;
#79251=DIRECTION('center_axis',(1.73472347597681E-16,-1.,8.55284707229503E-48)) ;
#79252=DIRECTION('ref_axis',(1.,1.73472347597681E-16,-1.48368246027497E-63)) ;
#79253=DIRECTION('center_axis',(0.,-1.,0.)) ;
#79254=DIRECTION('ref_axis',(0.,0.,-1.)) ;
#79255=DIRECTION('center_axis',(0.,0.,-1.)) ;
#79256=DIRECTION('ref_axis',(-1.,0.,0.)) ;
#79257=DIRECTION('center_axis',(-4.93038065763132E-32,0.,1.)) ;
#79258=DIRECTION('ref_axis',(1.,0.,4.93038065763132E-32)) ;
#79259=DIRECTION('center_axis',(0.,0.,-1.)) ;
#79260=DIRECTION('ref_axis',(-1.,0.,0.)) ;
#79261=DIRECTION('center_axis',(-4.93038065763132E-32,0.,1.)) ;
#79262=DIRECTION('ref_axis',(1.,0.,4.93038065763132E-32)) ;
#79263=DIRECTION('center_axis',(-2.60208521396521E-16,1.,-1.28292706084425E-47)) ;
#79264=DIRECTION('ref_axis',(-1.,-2.60208521396521E-16,3.33828553561868E-63)) ;
#79265=DIRECTION('center_axis',(0.,-1.,0.)) ;
#79266=DIRECTION('ref_axis',(0.,0.,-1.)) ;
#79267=DIRECTION('center_axis',(-4.93038065763132E-32,0.,1.)) ;
#79268=DIRECTION('ref_axis',(1.,0.,0.)) ;
#79269=DIRECTION('center_axis',(-1.,0.,0.)) ;
#79270=DIRECTION('ref_axis',(0.,0.,-1.)) ;
#79271=DIRECTION('center_axis',(-4.93038065763132E-32,0.,1.)) ;
#79272=DIRECTION('ref_axis',(1.,0.,0.)) ;
#79273=DIRECTION('center_axis',(1.,0.,0.)) ;
#79274=DIRECTION('ref_axis',(0.,0.,1.)) ;
#79275=DIRECTION('center_axis',(-1.,0.,-4.93038065763132E-32)) ;
#79276=DIRECTION('ref_axis',(-4.93038065763132E-32,0.,1.)) ;
#79277=DIRECTION('center_axis',(-3.65204942310907E-15,1.,-1.22867065825113E-46)) ;
#79278=DIRECTION('ref_axis',(-1.,-3.65204942310907E-15,-8.41343619123299E-62)) ;
#79279=DIRECTION('center_axis',(0.707106781186535,0.70710678118656,3.59045601457188E-14)) ;
#79280=DIRECTION('ref_axis',(0.70710678118656,-0.707106781186535,-1.32030231652671E-12)) ;
#79281=DIRECTION('center_axis',(0.,-1.,0.)) ;
#79282=DIRECTION('ref_axis',(0.,0.,-1.)) ;
#79283=DIRECTION('center_axis',(3.65204942310907E-15,-1.,-7.70988211545247E-16)) ;
#79284=DIRECTION('ref_axis',(1.,3.65204942310907E-15,-1.29620107950046E-43)) ;
#79285=DIRECTION('center_axis',(0.,-1.,0.)) ;
#79286=DIRECTION('ref_axis',(0.,0.,-1.)) ;
#79287=DIRECTION('center_axis',(0.707106781186586,0.707106781186509,6.51411305500852E-14)) ;
#79288=DIRECTION('ref_axis',(0.707106781186509,-0.707106781186586,-4.14202338982266E-13)) ;
#79289=DIRECTION('center_axis',(-1.03517906367563E-32,-1.81408990951823E-16,
1.)) ;
#79290=DIRECTION('ref_axis',(1.87790789395849E-48,-1.,-1.81408990951823E-16)) ;
#79291=DIRECTION('center_axis',(0.,-4.62592926927146E-14,1.)) ;
#79292=DIRECTION('ref_axis',(0.,-1.,-4.62592926927146E-14)) ;
#79293=DIRECTION('center_axis',(0.,0.,-1.)) ;
#79294=DIRECTION('ref_axis',(-1.,0.,0.)) ;
#79295=DIRECTION('center_axis',(0.,1.,0.)) ;
#79296=DIRECTION('ref_axis',(1.,0.,0.)) ;
#79297=DIRECTION('center_axis',(1.,0.,0.)) ;
#79298=DIRECTION('ref_axis',(0.,0.,1.)) ;
#79299=DIRECTION('center_axis',(-1.,-3.65204942310907E-15,-6.7286639138916E-31)) ;
#79300=DIRECTION('ref_axis',(3.65204942310907E-15,-1.,2.45734131650226E-45)) ;
#79301=DIRECTION('center_axis',(0.707106781186584,-0.707106781186511,5.62504775616304E-14)) ;
#79302=DIRECTION('ref_axis',(0.707106781186511,0.707106781186584,-5.62770983609062E-12)) ;
#79303=DIRECTION('center_axis',(-1.,-3.65204942310907E-15,-6.72866391389159E-31)) ;
#79304=DIRECTION('ref_axis',(3.65204942310907E-15,-1.,2.45734131650226E-45)) ;
#79305=DIRECTION('center_axis',(0.707106781186529,-0.707106781186566,5.43697625063671E-14)) ;
#79306=DIRECTION('ref_axis',(0.707106781186566,0.707106781186529,-3.4443471035871E-13)) ;
#79307=DIRECTION('center_axis',(0.,1.,0.)) ;
#79308=DIRECTION('ref_axis',(1.,0.,0.)) ;
#79309=DIRECTION('center_axis',(1.,0.,0.)) ;
#79310=DIRECTION('ref_axis',(0.,0.,1.)) ;
#79311=DIRECTION('center_axis',(-1.,-3.49148133884313E-15,-6.7286639138916E-31)) ;
#79312=DIRECTION('ref_axis',(3.49148133884313E-15,-1.,2.34930044906997E-45)) ;
#79313=DIRECTION('center_axis',(1.,0.,0.)) ;
#79314=DIRECTION('ref_axis',(0.,0.,-1.)) ;
#79315=DIRECTION('center_axis',(3.65204942310907E-15,-1.,1.22867065825113E-46)) ;
#79316=DIRECTION('ref_axis',(1.,3.65204942310907E-15,3.45446742203778E-76)) ;
#79317=DIRECTION('center_axis',(0.,-1.,0.)) ;
#79318=DIRECTION('ref_axis',(0.,0.,-1.)) ;
#79319=DIRECTION('center_axis',(-3.65204942310907E-15,1.,7.70988211545247E-16)) ;
#79320=DIRECTION('ref_axis',(-1.,-3.65204942310907E-15,5.2794132247463E-31)) ;
#79321=DIRECTION('center_axis',(0.,-1.,0.)) ;
#79322=DIRECTION('ref_axis',(0.,0.,-1.)) ;
#79323=DIRECTION('center_axis',(1.,3.49148133884313E-15,5.4907029126972E-31)) ;
#79324=DIRECTION('ref_axis',(-3.49148133884313E-15,1.,-1.91706867568139E-45)) ;
#79325=DIRECTION('center_axis',(1.,0.,0.)) ;
#79326=DIRECTION('ref_axis',(0.,0.,-1.)) ;
#79327=DIRECTION('center_axis',(0.,1.,0.)) ;
#79328=DIRECTION('ref_axis',(1.,0.,0.)) ;
#79329=DIRECTION('center_axis',(4.62592926927157E-14,0.,-1.)) ;
#79330=DIRECTION('ref_axis',(1.,0.,4.62592926927157E-14)) ;
#79331=DIRECTION('center_axis',(0.,1.,0.)) ;
#79332=DIRECTION('ref_axis',(1.,0.,0.)) ;
#79333=DIRECTION('center_axis',(0.,0.,1.)) ;
#79334=DIRECTION('ref_axis',(-1.,0.,0.)) ;
#79335=DIRECTION('center_axis',(1.03517906367563E-32,1.81408990951823E-16,
-1.)) ;
#79336=DIRECTION('ref_axis',(-1.73199155682659E-62,1.,1.81408990951823E-16)) ;
#99147=CARTESIAN_POINT('',(0.,0.,0.)) ;
#99148=CARTESIAN_POINT('Origin',(53.4,-9.74999999999999,-35.5)) ;
#99149=CARTESIAN_POINT('',(53.4,-11.35,-35.5)) ;
#99150=CARTESIAN_POINT('',(53.4,-8.14999999999999,-35.5)) ;
#99151=CARTESIAN_POINT('Origin',(53.4,-9.74999999999999,-35.5)) ;
#99152=CARTESIAN_POINT('Origin',(53.4,-9.74999999999999,-35.5)) ;
#99153=CARTESIAN_POINT('',(53.25,-8.,-35.5)) ;
#99154=CARTESIAN_POINT('Origin',(53.4,-7.99999999999999,-35.5)) ;
#99155=CARTESIAN_POINT('Origin',(53.25,-9.74999999999999,-35.5)) ;
#99156=CARTESIAN_POINT('Origin',(53.85,-9.74999999999999,-35.5)) ;
#99157=CARTESIAN_POINT('',(54.,-7.99999999999999,-35.5)) ;
#99158=CARTESIAN_POINT('Origin',(54.,-9.74999999999999,-35.5)) ;
#99159=CARTESIAN_POINT('',(53.85,-8.14999999999999,-35.5)) ;
#99160=CARTESIAN_POINT('Origin',(53.85,-7.99999999999999,-35.5)) ;
#99161=CARTESIAN_POINT('',(53.8500000000001,-11.35,-35.5)) ;
#99162=CARTESIAN_POINT('Origin',(53.85,-9.74999999999999,-35.5)) ;
#99163=CARTESIAN_POINT('Origin',(53.85,-9.74999999999999,-35.5)) ;
#99164=CARTESIAN_POINT('Origin',(43.,-0.162132034355965,-34.25)) ;
#99165=CARTESIAN_POINT('',(43.,-0.0560660171779847,-35.793933982822)) ;
#99166=CARTESIAN_POINT('',(43.,-0.0560660171779853,-32.706066017178)) ;
#99167=CARTESIAN_POINT('Origin',(43.,-0.056066017177985,-34.25)) ;
#99168=CARTESIAN_POINT('Origin',(43.,-0.056066017177985,-34.25)) ;
#99169=CARTESIAN_POINT('',(43.,-0.162132034355965,-32.75)) ;
#99170=CARTESIAN_POINT('Origin',(43.,-0.162132034355965,-32.6)) ;
#99171=CARTESIAN_POINT('',(43.,-0.162132034355965,-35.75)) ;
#99172=CARTESIAN_POINT('Origin',(43.,-0.162132034355965,-34.25)) ;
#99173=CARTESIAN_POINT('Origin',(43.,-0.162132034355965,-34.25)) ;
#99174=CARTESIAN_POINT('Origin',(43.,-0.600000000000015,-34.25)) ;
#99175=CARTESIAN_POINT('',(43.,-0.750000000000015,-35.9)) ;
#99176=CARTESIAN_POINT('Origin',(43.,-0.750000000000015,-34.25)) ;
#99177=CARTESIAN_POINT('',(43.,-0.600000000000015,-35.75)) ;
#99178=CARTESIAN_POINT('Origin',(43.,-0.600000000000015,-35.9)) ;
#99179=CARTESIAN_POINT('Origin',(43.,-0.600000000000015,-34.25)) ;
#99180=CARTESIAN_POINT('Origin',(43.,-0.162132034355978,34.25)) ;
#99181=CARTESIAN_POINT('',(43.,-0.0560660171779973,32.706066017178)) ;
#99182=CARTESIAN_POINT('',(43.,-0.0560660171779978,35.793933982822)) ;
#99183=CARTESIAN_POINT('Origin',(43.,-0.0560660171779975,34.25)) ;
#99184=CARTESIAN_POINT('Origin',(43.,-0.0560660171779975,34.25)) ;
#99185=CARTESIAN_POINT('',(43.,-0.162132034355978,35.75)) ;
#99186=CARTESIAN_POINT('Origin',(43.,-0.162132034355978,35.9)) ;
#99187=CARTESIAN_POINT('',(43.,-0.162132034355977,32.75)) ;
#99188=CARTESIAN_POINT('Origin',(43.,-0.162132034355978,34.25)) ;
#99189=CARTESIAN_POINT('Origin',(43.,-0.162132034355978,34.25)) ;
#99190=CARTESIAN_POINT('Origin',(43.,-0.600000000000027,34.25)) ;
#99191=CARTESIAN_POINT('',(43.,-0.750000000000027,32.6)) ;
#99192=CARTESIAN_POINT('Origin',(43.,-0.750000000000027,34.25)) ;
#99193=CARTESIAN_POINT('',(43.,-0.600000000000027,32.75)) ;
#99194=CARTESIAN_POINT('Origin',(43.,-0.600000000000027,32.6)) ;
#99195=CARTESIAN_POINT('Origin',(43.,-0.600000000000027,34.25)) ;
#99196=CARTESIAN_POINT('Origin',(43.,-6.29162293061953E-15,34.25)) ;
#99197=CARTESIAN_POINT('',(43.,-5.82322967106645E-15,32.65)) ;
#99198=CARTESIAN_POINT('',(43.,-5.99770769882417E-15,32.65)) ;
#99199=CARTESIAN_POINT('Origin',(43.,-6.29162293061953E-15,34.25)) ;
#99200=CARTESIAN_POINT('Origin',(43.,-6.29162293061953E-15,34.25)) ;
#99201=CARTESIAN_POINT('',(43.,-6.01607740081138E-15,32.75)) ;
#99202=CARTESIAN_POINT('Origin',(43.,6.29162293061953E-15,-34.25)) ;
#99203=CARTESIAN_POINT('',(43.,6.76001619017261E-15,-35.85)) ;
#99204=CARTESIAN_POINT('',(43.,6.5855381624149E-15,-35.85)) ;
#99205=CARTESIAN_POINT('Origin',(43.,6.29162293061953E-15,-34.25)) ;
#99206=CARTESIAN_POINT('Origin',(43.,6.29162293061953E-15,-34.25)) ;
#99207=CARTESIAN_POINT('',(43.,6.56716846042768E-15,-35.75)) ;
#99208=CARTESIAN_POINT('Origin',(-2.00100000000009,-9.7500000000002,-35.5)) ;
#99209=CARTESIAN_POINT('',(-2.00100000000008,-11.3500000000002,-35.5)) ;
#99210=CARTESIAN_POINT('Origin',(54.,1.9709024278469E-13,3.63163086615829E-29)) ;
#99211=CARTESIAN_POINT('',(54.,-1.74999999999999,38.25)) ;
#99212=CARTESIAN_POINT('',(54.,-1.74999999999999,39.85)) ;
#99213=CARTESIAN_POINT('',(54.,-1.74999999999999,38.25)) ;
#99214=CARTESIAN_POINT('',(54.0000000000001,-19.6,39.85)) ;
#99215=CARTESIAN_POINT('',(54.,1.9709024278469E-13,39.85)) ;
#99216=CARTESIAN_POINT('',(54.0000000000001,-19.6,-39.85)) ;
#99217=CARTESIAN_POINT('',(54.0000000000001,-19.6,-3.55561622265573E-15)) ;
#99218=CARTESIAN_POINT('',(54.,-1.74999999999998,-39.85)) ;
#99219=CARTESIAN_POINT('',(54.,-1.74999999999998,-39.85)) ;
#99220=CARTESIAN_POINT('',(54.,-1.74999999999998,-38.25)) ;
#99221=CARTESIAN_POINT('',(54.,-1.74999999999998,-38.25)) ;
#99222=CARTESIAN_POINT('',(54.,-1.74999999999998,-3.17465734165687E-16)) ;
#99223=CARTESIAN_POINT('',(54.,-4.39999999999999,-32.65)) ;
#99224=CARTESIAN_POINT('',(54.,-4.09999999999999,-32.35)) ;
#99225=CARTESIAN_POINT('Origin',(54.,-4.39999999999999,-32.35)) ;
#99226=CARTESIAN_POINT('',(54.0000000000001,-14.1,-32.65)) ;
#99227=CARTESIAN_POINT('',(54.,1.9709024278469E-13,-32.65)) ;
#99228=CARTESIAN_POINT('',(54.0000000000001,-14.4,-32.35)) ;
#99229=CARTESIAN_POINT('Origin',(54.0000000000001,-14.1,-32.35)) ;
#99230=CARTESIAN_POINT('',(54.0000000000001,-14.4,33.85)) ;
#99231=CARTESIAN_POINT('',(54.0000000000001,-14.4,3.63163086615829E-29)) ;
#99232=CARTESIAN_POINT('',(54.0000000000001,-14.1,34.15)) ;
#99233=CARTESIAN_POINT('Origin',(54.0000000000001,-14.1,33.85)) ;
#99234=CARTESIAN_POINT('',(54.,-4.39999999999999,34.15)) ;
#99235=CARTESIAN_POINT('',(54.,1.9709024278469E-13,34.15)) ;
#99236=CARTESIAN_POINT('',(54.,-4.09999999999999,33.85)) ;
#99237=CARTESIAN_POINT('Origin',(54.,-4.39999999999999,33.85)) ;
#99238=CARTESIAN_POINT('',(54.,-4.09999999999999,3.63163086615829E-29)) ;
#99239=CARTESIAN_POINT('Origin',(53.25,1.94471631780558E-13,3.58301353414727E-29)) ;
#99240=CARTESIAN_POINT('',(53.2500000000001,-19.6,-39.85)) ;
#99241=CARTESIAN_POINT('',(53.2500000000001,-19.6,39.85)) ;
#99242=CARTESIAN_POINT('',(53.2500000000001,-19.6,40.)) ;
#99243=CARTESIAN_POINT('',(53.25,-1.75,39.85)) ;
#99244=CARTESIAN_POINT('',(53.25,-1.75,39.85)) ;
#99245=CARTESIAN_POINT('',(53.25,-1.75,38.25)) ;
#99246=CARTESIAN_POINT('',(53.25,-1.75,38.25)) ;
#99247=CARTESIAN_POINT('',(53.25,-1.74999999999998,-38.25)) ;
#99248=CARTESIAN_POINT('',(53.25,-1.74999999999998,-38.25)) ;
#99249=CARTESIAN_POINT('',(53.25,-1.74999999999998,-39.85)) ;
#99250=CARTESIAN_POINT('',(53.25,-1.74999999999998,-38.25)) ;
#99251=CARTESIAN_POINT('',(53.25,2.25195512010636E-13,-39.85)) ;
#99252=CARTESIAN_POINT('',(53.2500000000001,-14.1,-32.65)) ;
#99253=CARTESIAN_POINT('',(53.2500000000001,-14.4,-32.35)) ;
#99254=CARTESIAN_POINT('Origin',(53.2500000000001,-14.1,-32.35)) ;
#99255=CARTESIAN_POINT('',(53.25,-4.4,-32.65)) ;
#99256=CARTESIAN_POINT('',(53.25,-4.25,-32.65)) ;
#99257=CARTESIAN_POINT('',(53.25,-4.1,-32.35)) ;
#99258=CARTESIAN_POINT('Origin',(53.25,-4.4,-32.35)) ;
#99259=CARTESIAN_POINT('',(53.25,-4.1,33.85)) ;
#99260=CARTESIAN_POINT('',(53.25,-4.1,34.)) ;
#99261=CARTESIAN_POINT('',(53.25,-4.4,34.15)) ;
#99262=CARTESIAN_POINT('Origin',(53.25,-4.4,33.85)) ;
#99263=CARTESIAN_POINT('',(53.2500000000001,-14.1,34.15)) ;
#99264=CARTESIAN_POINT('',(53.2500000000001,-14.2500000000002,34.15)) ;
#99265=CARTESIAN_POINT('',(53.2500000000001,-14.4,33.85)) ;
#99266=CARTESIAN_POINT('Origin',(53.2500000000001,-14.1,33.85)) ;
#99267=CARTESIAN_POINT('',(53.2500000000001,-14.4,-32.5)) ;
#99268=CARTESIAN_POINT('Origin',(53.25,-6.93889390390723E-15,-40.)) ;
#99269=CARTESIAN_POINT('',(0.149999999999965,-4.6,-40.)) ;
#99270=CARTESIAN_POINT('',(-0.150000000000035,-4.9,-40.)) ;
#99271=CARTESIAN_POINT('Origin',(-0.150000000000035,-4.6,-40.)) ;
#99272=CARTESIAN_POINT('',(0.149999999999963,-1.75,-40.)) ;
#99273=CARTESIAN_POINT('',(0.149999999999965,-1.75000000000001,-40.)) ;
#99274=CARTESIAN_POINT('',(52.25,-1.74999999999999,-40.)) ;
#99275=CARTESIAN_POINT('',(53.25,-1.75,-40.)) ;
#99276=CARTESIAN_POINT('',(53.,-1.75,-40.)) ;
#99277=CARTESIAN_POINT('',(53.25,-1.75,-40.)) ;
#99278=CARTESIAN_POINT('',(53.0000000000001,-19.6,-40.)) ;
#99279=CARTESIAN_POINT('',(53.,-7.81264669430658E-15,-40.)) ;
#99280=CARTESIAN_POINT('',(0.149999999999965,-19.6,-40.)) ;
#99281=CARTESIAN_POINT('',(53.25,-19.6,-40.)) ;
#99282=CARTESIAN_POINT('',(0.149999999999965,-6.90000000000001,-40.)) ;
#99283=CARTESIAN_POINT('',(0.149999999999965,-6.75000000000001,-40.)) ;
#99284=CARTESIAN_POINT('',(-0.150000000000035,-6.60000000000001,-40.)) ;
#99285=CARTESIAN_POINT('Origin',(-0.150000000000035,-6.90000000000001,-40.)) ;
#99286=CARTESIAN_POINT('',(-1.85000000000003,-6.60000000000001,-40.)) ;
#99287=CARTESIAN_POINT('',(-2.00000000000004,-6.60000000000001,-40.)) ;
#99288=CARTESIAN_POINT('',(-1.85000000000003,-4.9,-40.)) ;
#99289=CARTESIAN_POINT('',(-1.85000000000003,-4.75000000000001,-40.)) ;
#99290=CARTESIAN_POINT('',(-2.77555756156289E-14,-4.9,-40.)) ;
#99291=CARTESIAN_POINT('',(19.1,-2.90000000000002,-40.)) ;
#99292=CARTESIAN_POINT('',(19.4,-2.60000000000002,-40.)) ;
#99293=CARTESIAN_POINT('Origin',(19.4,-2.90000000000002,-40.)) ;
#99294=CARTESIAN_POINT('',(19.1,-13.1,-40.)) ;
#99295=CARTESIAN_POINT('',(19.1,-13.25,-40.)) ;
#99296=CARTESIAN_POINT('',(19.4,-13.4,-40.)) ;
#99297=CARTESIAN_POINT('Origin',(19.4,-13.1,-40.)) ;
#99298=CARTESIAN_POINT('',(38.1,-13.4,-40.)) ;
#99299=CARTESIAN_POINT('',(38.25,-13.4,-40.)) ;
#99300=CARTESIAN_POINT('',(38.4,-13.1,-40.)) ;
#99301=CARTESIAN_POINT('Origin',(38.1,-13.1,-40.)) ;
#99302=CARTESIAN_POINT('',(38.4,-2.90000000000002,-40.)) ;
#99303=CARTESIAN_POINT('',(38.4,-2.75000000000002,-40.)) ;
#99304=CARTESIAN_POINT('',(38.1,-2.60000000000002,-40.)) ;
#99305=CARTESIAN_POINT('Origin',(38.1,-2.90000000000002,-40.)) ;
#99306=CARTESIAN_POINT('',(19.25,-2.60000000000002,-40.)) ;
#99307=CARTESIAN_POINT('',(7.34999999999997,-5.40000000000002,-40.)) ;
#99308=CARTESIAN_POINT('',(7.64999999999997,-5.10000000000002,-40.)) ;
#99309=CARTESIAN_POINT('Origin',(7.64999999999997,-5.40000000000002,-40.)) ;
#99310=CARTESIAN_POINT('',(7.34999999999996,-15.1,-40.)) ;
#99311=CARTESIAN_POINT('',(7.34999999999996,-15.25,-40.)) ;
#99312=CARTESIAN_POINT('',(7.64999999999996,-15.4,-40.)) ;
#99313=CARTESIAN_POINT('Origin',(7.64999999999996,-15.1,-40.)) ;
#99314=CARTESIAN_POINT('',(10.35,-15.4,-40.)) ;
#99315=CARTESIAN_POINT('',(10.5,-15.4,-40.)) ;
#99316=CARTESIAN_POINT('',(10.65,-15.1,-40.)) ;
#99317=CARTESIAN_POINT('Origin',(10.35,-15.1,-40.)) ;
#99318=CARTESIAN_POINT('',(10.65,-5.40000000000002,-40.)) ;
#99319=CARTESIAN_POINT('',(10.65,-5.25000000000002,-40.)) ;
#99320=CARTESIAN_POINT('',(10.35,-5.10000000000002,-40.)) ;
#99321=CARTESIAN_POINT('Origin',(10.35,-5.40000000000002,-40.)) ;
#99322=CARTESIAN_POINT('',(7.49999999999997,-5.10000000000002,-40.)) ;
#99323=CARTESIAN_POINT('',(16.65,-15.1000000000001,-40.)) ;
#99324=CARTESIAN_POINT('',(16.35,-15.4000000000001,-40.)) ;
#99325=CARTESIAN_POINT('Origin',(16.35,-15.1000000000001,-40.)) ;
#99326=CARTESIAN_POINT('',(16.65,-5.40000000000006,-40.)) ;
#99327=CARTESIAN_POINT('',(16.65,-5.25000000000006,-40.)) ;
#99328=CARTESIAN_POINT('',(16.35,-5.10000000000006,-40.)) ;
#99329=CARTESIAN_POINT('Origin',(16.35,-5.40000000000006,-40.)) ;
#99330=CARTESIAN_POINT('',(13.65,-5.10000000000006,-40.)) ;
#99331=CARTESIAN_POINT('',(13.5,-5.10000000000006,-40.)) ;
#99332=CARTESIAN_POINT('',(13.35,-5.40000000000006,-40.)) ;
#99333=CARTESIAN_POINT('Origin',(13.65,-5.40000000000006,-40.)) ;
#99334=CARTESIAN_POINT('',(13.35,-15.1000000000001,-40.)) ;
#99335=CARTESIAN_POINT('',(13.35,-15.2500000000001,-40.)) ;
#99336=CARTESIAN_POINT('',(13.65,-15.4000000000001,-40.)) ;
#99337=CARTESIAN_POINT('Origin',(13.65,-15.1000000000001,-40.)) ;
#99338=CARTESIAN_POINT('',(16.5,-15.4000000000001,-40.)) ;
#99339=CARTESIAN_POINT('',(46.65,-15.1000000000003,-40.)) ;
#99340=CARTESIAN_POINT('',(46.35,-15.4000000000003,-40.)) ;
#99341=CARTESIAN_POINT('Origin',(46.35,-15.1000000000003,-40.)) ;
#99342=CARTESIAN_POINT('',(46.65,-5.40000000000027,-40.)) ;
#99343=CARTESIAN_POINT('',(46.65,-5.25000000000027,-40.)) ;
#99344=CARTESIAN_POINT('',(46.35,-5.10000000000027,-40.)) ;
#99345=CARTESIAN_POINT('Origin',(46.35,-5.40000000000027,-40.)) ;
#99346=CARTESIAN_POINT('',(43.65,-5.10000000000027,-40.)) ;
#99347=CARTESIAN_POINT('',(43.5,-5.10000000000027,-40.)) ;
#99348=CARTESIAN_POINT('',(43.35,-5.40000000000027,-40.)) ;
#99349=CARTESIAN_POINT('Origin',(43.65,-5.40000000000027,-40.)) ;
#99350=CARTESIAN_POINT('',(43.35,-15.1000000000003,-40.)) ;
#99351=CARTESIAN_POINT('',(43.35,-15.2500000000003,-40.)) ;
#99352=CARTESIAN_POINT('',(43.65,-15.4000000000003,-40.)) ;
#99353=CARTESIAN_POINT('Origin',(43.65,-15.1000000000003,-40.)) ;
#99354=CARTESIAN_POINT('',(46.5,-15.4000000000003,-40.)) ;
#99355=CARTESIAN_POINT('Origin',(53.25,-6.93889390390723E-15,-39.25)) ;
#99356=CARTESIAN_POINT('',(52.25,-1.74999999999999,-39.25)) ;
#99357=CARTESIAN_POINT('',(0.149999999999963,-1.75,-39.25)) ;
#99358=CARTESIAN_POINT('',(53.25,-1.75,-39.25)) ;
#99359=CARTESIAN_POINT('',(0.149999999999963,-4.6,-39.25)) ;
#99360=CARTESIAN_POINT('',(0.149999999999963,-6.93889390390723E-15,-39.25)) ;
#99361=CARTESIAN_POINT('',(-0.150000000000035,-4.9,-39.25)) ;
#99362=CARTESIAN_POINT('Origin',(-0.150000000000035,-4.6,-39.25)) ;
#99363=CARTESIAN_POINT('',(-1.85000000000003,-4.9,-39.25)) ;
#99364=CARTESIAN_POINT('',(53.25,-4.9,-39.25)) ;
#99365=CARTESIAN_POINT('',(-1.85000000000003,-6.60000000000001,-39.25)) ;
#99366=CARTESIAN_POINT('',(-1.85000000000003,-1.88868018446975E-14,-39.25)) ;
#99367=CARTESIAN_POINT('',(-0.150000000000035,-6.60000000000001,-39.25)) ;
#99368=CARTESIAN_POINT('',(53.25,-6.60000000000001,-39.25)) ;
#99369=CARTESIAN_POINT('',(0.149999999999963,-6.90000000000001,-39.25)) ;
#99370=CARTESIAN_POINT('Origin',(-0.150000000000035,-6.90000000000001,-39.25)) ;
#99371=CARTESIAN_POINT('',(0.149999999999963,-19.6,-39.25)) ;
#99372=CARTESIAN_POINT('',(0.149999999999963,-6.93889390390723E-15,-39.25)) ;
#99373=CARTESIAN_POINT('',(53.0000000000001,-19.6,-39.25)) ;
#99374=CARTESIAN_POINT('',(53.15,-19.6,-39.25)) ;
#99375=CARTESIAN_POINT('',(53.,-1.75,-39.25)) ;
#99376=CARTESIAN_POINT('',(53.,-1.75,-39.25)) ;
#99377=CARTESIAN_POINT('',(53.25,-1.75,-39.25)) ;
#99378=CARTESIAN_POINT('',(19.1,-13.1,-39.25)) ;
#99379=CARTESIAN_POINT('',(19.4,-13.4,-39.25)) ;
#99380=CARTESIAN_POINT('Origin',(19.4,-13.1,-39.25)) ;
#99381=CARTESIAN_POINT('',(19.1,-2.90000000000002,-39.25)) ;
#99382=CARTESIAN_POINT('',(19.1,-6.93889390390723E-15,-39.25)) ;
#99383=CARTESIAN_POINT('',(19.4,-2.60000000000002,-39.25)) ;
#99384=CARTESIAN_POINT('Origin',(19.4,-2.90000000000002,-39.25)) ;
#99385=CARTESIAN_POINT('',(38.1,-2.60000000000002,-39.25)) ;
#99386=CARTESIAN_POINT('',(53.25,-2.60000000000002,-39.25)) ;
#99387=CARTESIAN_POINT('',(38.4,-2.90000000000002,-39.25)) ;
#99388=CARTESIAN_POINT('Origin',(38.1,-2.90000000000002,-39.25)) ;
#99389=CARTESIAN_POINT('',(38.4,-13.1,-39.25)) ;
#99390=CARTESIAN_POINT('',(38.4,-6.93889390390723E-15,-39.25)) ;
#99391=CARTESIAN_POINT('',(38.1,-13.4,-39.25)) ;
#99392=CARTESIAN_POINT('Origin',(38.1,-13.1,-39.25)) ;
#99393=CARTESIAN_POINT('',(53.25,-13.4,-39.25)) ;
#99394=CARTESIAN_POINT('',(7.34999999999996,-15.1,-39.25)) ;
#99395=CARTESIAN_POINT('',(7.64999999999996,-15.4,-39.25)) ;
#99396=CARTESIAN_POINT('Origin',(7.64999999999996,-15.1,-39.25)) ;
#99397=CARTESIAN_POINT('',(7.34999999999997,-5.40000000000002,-39.25)) ;
#99398=CARTESIAN_POINT('',(7.34999999999997,-2.95770352654046E-15,-39.25)) ;
#99399=CARTESIAN_POINT('',(7.64999999999997,-5.10000000000002,-39.25)) ;
#99400=CARTESIAN_POINT('Origin',(7.64999999999997,-5.40000000000002,-39.25)) ;
#99401=CARTESIAN_POINT('',(10.35,-5.10000000000002,-39.25)) ;
#99402=CARTESIAN_POINT('',(53.25,-5.10000000000002,-39.25)) ;
#99403=CARTESIAN_POINT('',(10.65,-5.40000000000002,-39.25)) ;
#99404=CARTESIAN_POINT('Origin',(10.35,-5.40000000000002,-39.25)) ;
#99405=CARTESIAN_POINT('',(10.65,-15.1,-39.25)) ;
#99406=CARTESIAN_POINT('',(10.65,4.51028103753969E-16,-39.25)) ;
#99407=CARTESIAN_POINT('',(10.35,-15.4,-39.25)) ;
#99408=CARTESIAN_POINT('Origin',(10.35,-15.1,-39.25)) ;
#99409=CARTESIAN_POINT('',(53.25,-15.4,-39.25)) ;
#99410=CARTESIAN_POINT('',(16.65,-5.40000000000006,-39.25)) ;
#99411=CARTESIAN_POINT('',(16.35,-5.10000000000006,-39.25)) ;
#99412=CARTESIAN_POINT('Origin',(16.35,-5.40000000000006,-39.25)) ;
#99413=CARTESIAN_POINT('',(16.65,-15.1000000000001,-39.25)) ;
#99414=CARTESIAN_POINT('',(16.65,5.759281940243E-15,-39.25)) ;
#99415=CARTESIAN_POINT('',(16.35,-15.4000000000001,-39.25)) ;
#99416=CARTESIAN_POINT('Origin',(16.35,-15.1000000000001,-39.25)) ;
#99417=CARTESIAN_POINT('',(13.65,-15.4000000000001,-39.25)) ;
#99418=CARTESIAN_POINT('',(53.25,-15.4000000000001,-39.25)) ;
#99419=CARTESIAN_POINT('',(13.35,-15.1000000000001,-39.25)) ;
#99420=CARTESIAN_POINT('Origin',(13.65,-15.1000000000001,-39.25)) ;
#99421=CARTESIAN_POINT('',(13.35,-5.40000000000006,-39.25)) ;
#99422=CARTESIAN_POINT('',(13.35,-1.73472347597685E-17,-39.25)) ;
#99423=CARTESIAN_POINT('',(13.65,-5.10000000000006,-39.25)) ;
#99424=CARTESIAN_POINT('Origin',(13.65,-5.40000000000006,-39.25)) ;
#99425=CARTESIAN_POINT('',(53.25,-5.10000000000006,-39.25)) ;
#99426=CARTESIAN_POINT('',(46.65,-5.40000000000027,-39.25)) ;
#99427=CARTESIAN_POINT('',(46.35,-5.10000000000027,-39.25)) ;
#99428=CARTESIAN_POINT('Origin',(46.35,-5.40000000000027,-39.25)) ;
#99429=CARTESIAN_POINT('',(46.65,-15.1000000000003,-39.25)) ;
#99430=CARTESIAN_POINT('',(46.65,-2.35922392732846E-15,-39.25)) ;
#99431=CARTESIAN_POINT('',(46.35,-15.4000000000003,-39.25)) ;
#99432=CARTESIAN_POINT('Origin',(46.35,-15.1000000000003,-39.25)) ;
#99433=CARTESIAN_POINT('',(43.65,-15.4000000000003,-39.25)) ;
#99434=CARTESIAN_POINT('',(53.25,-15.4000000000003,-39.25)) ;
#99435=CARTESIAN_POINT('',(43.35,-15.1000000000003,-39.25)) ;
#99436=CARTESIAN_POINT('Origin',(43.65,-15.1000000000003,-39.25)) ;
#99437=CARTESIAN_POINT('',(43.35,-5.40000000000027,-39.25)) ;
#99438=CARTESIAN_POINT('',(43.35,-6.93889390390723E-15,-39.25)) ;
#99439=CARTESIAN_POINT('',(43.65,-5.10000000000027,-39.25)) ;
#99440=CARTESIAN_POINT('Origin',(43.65,-5.40000000000027,-39.25)) ;
#99441=CARTESIAN_POINT('',(53.25,-5.10000000000027,-39.25)) ;
#99442=CARTESIAN_POINT('Origin',(53.25,-19.75,40.)) ;
#99443=CARTESIAN_POINT('',(52.25,-1.75,40.)) ;
#99444=CARTESIAN_POINT('',(0.14999999999997,-1.75000000000002,40.)) ;
#99445=CARTESIAN_POINT('',(53.25,-1.75000000000002,40.)) ;
#99446=CARTESIAN_POINT('',(0.149999999999972,-4.60000000000001,40.)) ;
#99447=CARTESIAN_POINT('',(0.14999999999997,-19.75,40.)) ;
#99448=CARTESIAN_POINT('',(-0.150000000000028,-4.90000000000001,40.)) ;
#99449=CARTESIAN_POINT('Origin',(-0.150000000000028,-4.60000000000001,40.)) ;
#99450=CARTESIAN_POINT('',(-1.85000000000004,-4.90000000000001,40.)) ;
#99451=CARTESIAN_POINT('',(53.25,-4.90000000000001,40.)) ;
#99452=CARTESIAN_POINT('',(-1.85000000000003,-6.60000000000001,40.)) ;
#99453=CARTESIAN_POINT('',(-1.85000000000003,-19.75,40.)) ;
#99454=CARTESIAN_POINT('',(-0.150000000000028,-6.60000000000001,40.)) ;
#99455=CARTESIAN_POINT('',(53.25,-6.60000000000001,40.)) ;
#99456=CARTESIAN_POINT('',(0.149999999999972,-6.90000000000001,40.)) ;
#99457=CARTESIAN_POINT('Origin',(-0.150000000000028,-6.90000000000001,40.)) ;
#99458=CARTESIAN_POINT('',(0.149999999999972,-19.6,40.)) ;
#99459=CARTESIAN_POINT('',(0.14999999999997,-19.75,40.)) ;
#99460=CARTESIAN_POINT('',(53.,-19.6,40.)) ;
#99461=CARTESIAN_POINT('',(53.25,-19.6,40.)) ;
#99462=CARTESIAN_POINT('',(53.,-1.75000000000002,40.)) ;
#99463=CARTESIAN_POINT('',(53.,-1.75000000000002,40.)) ;
#99464=CARTESIAN_POINT('',(53.25,-1.75000000000002,40.)) ;
#99465=CARTESIAN_POINT('',(10.65,-5.40000000000002,40.)) ;
#99466=CARTESIAN_POINT('',(10.35,-5.10000000000002,40.)) ;
#99467=CARTESIAN_POINT('Origin',(10.35,-5.40000000000002,40.)) ;
#99468=CARTESIAN_POINT('',(10.65,-15.1,40.)) ;
#99469=CARTESIAN_POINT('',(10.65,-15.25,40.)) ;
#99470=CARTESIAN_POINT('',(10.35,-15.4,40.)) ;
#99471=CARTESIAN_POINT('Origin',(10.35,-15.1,40.)) ;
#99472=CARTESIAN_POINT('',(7.64999999999997,-15.4,40.)) ;
#99473=CARTESIAN_POINT('',(7.49999999999997,-15.4,40.)) ;
#99474=CARTESIAN_POINT('',(7.34999999999997,-15.1,40.)) ;
#99475=CARTESIAN_POINT('Origin',(7.64999999999997,-15.1,40.)) ;
#99476=CARTESIAN_POINT('',(7.34999999999996,-5.40000000000002,40.)) ;
#99477=CARTESIAN_POINT('',(7.34999999999996,-5.25000000000002,40.)) ;
#99478=CARTESIAN_POINT('',(7.64999999999996,-5.10000000000002,40.)) ;
#99479=CARTESIAN_POINT('Origin',(7.64999999999996,-5.40000000000002,40.)) ;
#99480=CARTESIAN_POINT('',(10.5,-5.10000000000002,40.)) ;
#99481=CARTESIAN_POINT('',(22.65,-5.40000000000002,40.)) ;
#99482=CARTESIAN_POINT('',(22.35,-5.10000000000002,40.)) ;
#99483=CARTESIAN_POINT('Origin',(22.35,-5.40000000000002,40.)) ;
#99484=CARTESIAN_POINT('',(22.65,-15.1,40.)) ;
#99485=CARTESIAN_POINT('',(22.65,-15.25,40.)) ;
#99486=CARTESIAN_POINT('',(22.35,-15.4,40.)) ;
#99487=CARTESIAN_POINT('Origin',(22.35,-15.1,40.)) ;
#99488=CARTESIAN_POINT('',(19.65,-15.4,40.)) ;
#99489=CARTESIAN_POINT('',(19.5,-15.4,40.)) ;
#99490=CARTESIAN_POINT('',(19.35,-15.1,40.)) ;
#99491=CARTESIAN_POINT('Origin',(19.65,-15.1,40.)) ;
#99492=CARTESIAN_POINT('',(19.35,-5.40000000000002,40.)) ;
#99493=CARTESIAN_POINT('',(19.35,-5.25000000000002,40.)) ;
#99494=CARTESIAN_POINT('',(19.65,-5.10000000000002,40.)) ;
#99495=CARTESIAN_POINT('Origin',(19.65,-5.40000000000002,40.)) ;
#99496=CARTESIAN_POINT('',(22.5,-5.10000000000002,40.)) ;
#99497=CARTESIAN_POINT('',(34.65,-5.40000000000002,40.)) ;
#99498=CARTESIAN_POINT('',(34.35,-5.10000000000002,40.)) ;
#99499=CARTESIAN_POINT('Origin',(34.35,-5.40000000000002,40.)) ;
#99500=CARTESIAN_POINT('',(34.65,-15.1,40.)) ;
#99501=CARTESIAN_POINT('',(34.65,-15.25,40.)) ;
#99502=CARTESIAN_POINT('',(34.35,-15.4,40.)) ;
#99503=CARTESIAN_POINT('Origin',(34.35,-15.1,40.)) ;
#99504=CARTESIAN_POINT('',(31.65,-15.4,40.)) ;
#99505=CARTESIAN_POINT('',(31.5,-15.4,40.)) ;
#99506=CARTESIAN_POINT('',(31.35,-15.1,40.)) ;
#99507=CARTESIAN_POINT('Origin',(31.65,-15.1,40.)) ;
#99508=CARTESIAN_POINT('',(31.35,-5.40000000000002,40.)) ;
#99509=CARTESIAN_POINT('',(31.35,-5.25000000000002,40.)) ;
#99510=CARTESIAN_POINT('',(31.65,-5.10000000000002,40.)) ;
#99511=CARTESIAN_POINT('Origin',(31.65,-5.40000000000002,40.)) ;
#99512=CARTESIAN_POINT('',(34.5,-5.10000000000002,40.)) ;
#99513=CARTESIAN_POINT('',(46.65,-5.40000000000002,40.)) ;
#99514=CARTESIAN_POINT('',(46.35,-5.10000000000002,40.)) ;
#99515=CARTESIAN_POINT('Origin',(46.35,-5.40000000000002,40.)) ;
#99516=CARTESIAN_POINT('',(46.65,-15.1,40.)) ;
#99517=CARTESIAN_POINT('',(46.65,-15.25,40.)) ;
#99518=CARTESIAN_POINT('',(46.35,-15.4,40.)) ;
#99519=CARTESIAN_POINT('Origin',(46.35,-15.1,40.)) ;
#99520=CARTESIAN_POINT('',(43.65,-15.4,40.)) ;
#99521=CARTESIAN_POINT('',(43.5,-15.4,40.)) ;
#99522=CARTESIAN_POINT('',(43.35,-15.1,40.)) ;
#99523=CARTESIAN_POINT('Origin',(43.65,-15.1,40.)) ;
#99524=CARTESIAN_POINT('',(43.35,-5.40000000000002,40.)) ;
#99525=CARTESIAN_POINT('',(43.35,-5.25000000000002,40.)) ;
#99526=CARTESIAN_POINT('',(43.65,-5.10000000000002,40.)) ;
#99527=CARTESIAN_POINT('Origin',(43.65,-5.40000000000002,40.)) ;
#99528=CARTESIAN_POINT('',(46.5,-5.10000000000002,40.)) ;
#99529=CARTESIAN_POINT('',(40.65,-5.40000000000002,40.)) ;
#99530=CARTESIAN_POINT('',(40.35,-5.10000000000002,40.)) ;
#99531=CARTESIAN_POINT('Origin',(40.35,-5.40000000000002,40.)) ;
#99532=CARTESIAN_POINT('',(40.65,-15.1,40.)) ;
#99533=CARTESIAN_POINT('',(40.65,-15.25,40.)) ;
#99534=CARTESIAN_POINT('',(40.35,-15.4,40.)) ;
#99535=CARTESIAN_POINT('Origin',(40.35,-15.1,40.)) ;
#99536=CARTESIAN_POINT('',(37.65,-15.4,40.)) ;
#99537=CARTESIAN_POINT('',(37.5,-15.4,40.)) ;
#99538=CARTESIAN_POINT('',(37.35,-15.1,40.)) ;
#99539=CARTESIAN_POINT('Origin',(37.65,-15.1,40.)) ;
#99540=CARTESIAN_POINT('',(37.35,-5.40000000000002,40.)) ;
#99541=CARTESIAN_POINT('',(37.35,-5.25000000000002,40.)) ;
#99542=CARTESIAN_POINT('',(37.65,-5.10000000000002,40.)) ;
#99543=CARTESIAN_POINT('Origin',(37.65,-5.40000000000002,40.)) ;
#99544=CARTESIAN_POINT('',(40.5,-5.10000000000002,40.)) ;
#99545=CARTESIAN_POINT('',(28.65,-5.40000000000002,40.)) ;
#99546=CARTESIAN_POINT('',(28.35,-5.10000000000002,40.)) ;
#99547=CARTESIAN_POINT('Origin',(28.35,-5.40000000000002,40.)) ;
#99548=CARTESIAN_POINT('',(28.65,-15.1,40.)) ;
#99549=CARTESIAN_POINT('',(28.65,-15.25,40.)) ;
#99550=CARTESIAN_POINT('',(28.35,-15.4,40.)) ;
#99551=CARTESIAN_POINT('Origin',(28.35,-15.1,40.)) ;
#99552=CARTESIAN_POINT('',(25.65,-15.4,40.)) ;
#99553=CARTESIAN_POINT('',(25.5,-15.4,40.)) ;
#99554=CARTESIAN_POINT('',(25.35,-15.1,40.)) ;
#99555=CARTESIAN_POINT('Origin',(25.65,-15.1,40.)) ;
#99556=CARTESIAN_POINT('',(25.35,-5.40000000000002,40.)) ;
#99557=CARTESIAN_POINT('',(25.35,-5.25000000000002,40.)) ;
#99558=CARTESIAN_POINT('',(25.65,-5.10000000000002,40.)) ;
#99559=CARTESIAN_POINT('Origin',(25.65,-5.40000000000002,40.)) ;
#99560=CARTESIAN_POINT('',(28.5,-5.10000000000002,40.)) ;
#99561=CARTESIAN_POINT('',(13.35,-15.1,40.)) ;
#99562=CARTESIAN_POINT('',(13.65,-15.4,40.)) ;
#99563=CARTESIAN_POINT('Origin',(13.65,-15.1,40.)) ;
#99564=CARTESIAN_POINT('',(13.35,-5.40000000000002,40.)) ;
#99565=CARTESIAN_POINT('',(13.35,-5.25000000000002,40.)) ;
#99566=CARTESIAN_POINT('',(13.65,-5.10000000000002,40.)) ;
#99567=CARTESIAN_POINT('Origin',(13.65,-5.40000000000002,40.)) ;
#99568=CARTESIAN_POINT('',(16.35,-5.10000000000002,40.)) ;
#99569=CARTESIAN_POINT('',(16.5,-5.10000000000002,40.)) ;
#99570=CARTESIAN_POINT('',(16.65,-5.40000000000002,40.)) ;
#99571=CARTESIAN_POINT('Origin',(16.35,-5.40000000000002,40.)) ;
#99572=CARTESIAN_POINT('',(16.65,-15.1,40.)) ;
#99573=CARTESIAN_POINT('',(16.65,-15.25,40.)) ;
#99574=CARTESIAN_POINT('',(16.35,-15.4,40.)) ;
#99575=CARTESIAN_POINT('Origin',(16.35,-15.1,40.)) ;
#99576=CARTESIAN_POINT('',(13.5,-15.4,40.)) ;
#99577=CARTESIAN_POINT('Origin',(53.25,-19.75,39.25)) ;
#99578=CARTESIAN_POINT('',(0.14999999999997,-4.60000000000001,39.25)) ;
#99579=CARTESIAN_POINT('',(-0.150000000000028,-4.90000000000001,39.25)) ;
#99580=CARTESIAN_POINT('Origin',(-0.150000000000028,-4.60000000000001,39.25)) ;
#99581=CARTESIAN_POINT('',(0.14999999999997,-1.75000000000002,39.25)) ;
#99582=CARTESIAN_POINT('',(0.14999999999997,-1.75000000000001,39.25)) ;
#99583=CARTESIAN_POINT('',(52.25,-1.75000000000001,39.25)) ;
#99584=CARTESIAN_POINT('',(53.25,-1.75000000000002,39.25)) ;
#99585=CARTESIAN_POINT('',(53.,-1.75000000000002,39.25)) ;
#99586=CARTESIAN_POINT('',(53.25,-1.75000000000002,39.25)) ;
#99587=CARTESIAN_POINT('',(53.,-19.6,39.25)) ;
#99588=CARTESIAN_POINT('',(53.,-19.75,39.25)) ;
#99589=CARTESIAN_POINT('',(0.14999999999997,-19.6,39.25)) ;
#99590=CARTESIAN_POINT('',(-3.46944695195361E-14,-19.6,39.25)) ;
#99591=CARTESIAN_POINT('',(0.14999999999997,-6.90000000000001,39.25)) ;
#99592=CARTESIAN_POINT('',(0.14999999999997,-6.75000000000001,39.25)) ;
#99593=CARTESIAN_POINT('',(-0.150000000000028,-6.60000000000001,39.25)) ;
#99594=CARTESIAN_POINT('Origin',(-0.150000000000028,-6.90000000000001,39.25)) ;
#99595=CARTESIAN_POINT('',(-1.85000000000003,-6.60000000000001,39.25)) ;
#99596=CARTESIAN_POINT('',(-2.00000000000003,-6.60000000000001,39.25)) ;
#99597=CARTESIAN_POINT('',(-1.85000000000003,-4.90000000000001,39.25)) ;
#99598=CARTESIAN_POINT('',(-1.85000000000003,-4.75000000000002,39.25)) ;
#99599=CARTESIAN_POINT('',(-2.77555756156289E-14,-4.90000000000001,39.25)) ;
#99600=CARTESIAN_POINT('',(10.65,-15.1,39.25)) ;
#99601=CARTESIAN_POINT('',(10.35,-15.4,39.25)) ;
#99602=CARTESIAN_POINT('Origin',(10.35,-15.1,39.25)) ;
#99603=CARTESIAN_POINT('',(10.65,-5.40000000000002,39.25)) ;
#99604=CARTESIAN_POINT('',(10.65,-19.75,39.25)) ;
#99605=CARTESIAN_POINT('',(10.35,-5.10000000000002,39.25)) ;
#99606=CARTESIAN_POINT('Origin',(10.35,-5.40000000000002,39.25)) ;
#99607=CARTESIAN_POINT('',(7.64999999999996,-5.10000000000002,39.25)) ;
#99608=CARTESIAN_POINT('',(53.25,-5.10000000000002,39.25)) ;
#99609=CARTESIAN_POINT('',(7.34999999999996,-5.40000000000002,39.25)) ;
#99610=CARTESIAN_POINT('Origin',(7.64999999999996,-5.40000000000002,39.25)) ;
#99611=CARTESIAN_POINT('',(7.34999999999997,-15.1,39.25)) ;
#99612=CARTESIAN_POINT('',(7.34999999999997,-19.75,39.25)) ;
#99613=CARTESIAN_POINT('',(7.64999999999997,-15.4,39.25)) ;
#99614=CARTESIAN_POINT('Origin',(7.64999999999997,-15.1,39.25)) ;
#99615=CARTESIAN_POINT('',(53.25,-15.4,39.25)) ;
#99616=CARTESIAN_POINT('',(22.65,-15.1,39.25)) ;
#99617=CARTESIAN_POINT('',(22.35,-15.4,39.25)) ;
#99618=CARTESIAN_POINT('Origin',(22.35,-15.1,39.25)) ;
#99619=CARTESIAN_POINT('',(22.65,-5.40000000000002,39.25)) ;
#99620=CARTESIAN_POINT('',(22.65,-19.75,39.25)) ;
#99621=CARTESIAN_POINT('',(22.35,-5.10000000000002,39.25)) ;
#99622=CARTESIAN_POINT('Origin',(22.35,-5.40000000000002,39.25)) ;
#99623=CARTESIAN_POINT('',(19.65,-5.10000000000002,39.25)) ;
#99624=CARTESIAN_POINT('',(53.25,-5.10000000000002,39.25)) ;
#99625=CARTESIAN_POINT('',(19.35,-5.40000000000002,39.25)) ;
#99626=CARTESIAN_POINT('Origin',(19.65,-5.40000000000002,39.25)) ;
#99627=CARTESIAN_POINT('',(19.35,-15.1,39.25)) ;
#99628=CARTESIAN_POINT('',(19.35,-19.75,39.25)) ;
#99629=CARTESIAN_POINT('',(19.65,-15.4,39.25)) ;
#99630=CARTESIAN_POINT('Origin',(19.65,-15.1,39.25)) ;
#99631=CARTESIAN_POINT('',(53.25,-15.4,39.25)) ;
#99632=CARTESIAN_POINT('',(34.65,-15.1,39.25)) ;
#99633=CARTESIAN_POINT('',(34.35,-15.4,39.25)) ;
#99634=CARTESIAN_POINT('Origin',(34.35,-15.1,39.25)) ;
#99635=CARTESIAN_POINT('',(34.65,-5.40000000000002,39.25)) ;
#99636=CARTESIAN_POINT('',(34.65,-19.75,39.25)) ;
#99637=CARTESIAN_POINT('',(34.35,-5.10000000000002,39.25)) ;
#99638=CARTESIAN_POINT('Origin',(34.35,-5.40000000000002,39.25)) ;
#99639=CARTESIAN_POINT('',(31.65,-5.10000000000002,39.25)) ;
#99640=CARTESIAN_POINT('',(53.25,-5.10000000000002,39.25)) ;
#99641=CARTESIAN_POINT('',(31.35,-5.40000000000002,39.25)) ;
#99642=CARTESIAN_POINT('Origin',(31.65,-5.40000000000002,39.25)) ;
#99643=CARTESIAN_POINT('',(31.35,-15.1,39.25)) ;
#99644=CARTESIAN_POINT('',(31.35,-19.75,39.25)) ;
#99645=CARTESIAN_POINT('',(31.65,-15.4,39.25)) ;
#99646=CARTESIAN_POINT('Origin',(31.65,-15.1,39.25)) ;
#99647=CARTESIAN_POINT('',(53.25,-15.4,39.25)) ;
#99648=CARTESIAN_POINT('',(46.65,-15.1,39.25)) ;
#99649=CARTESIAN_POINT('',(46.35,-15.4,39.25)) ;
#99650=CARTESIAN_POINT('Origin',(46.35,-15.1,39.25)) ;
#99651=CARTESIAN_POINT('',(46.65,-5.40000000000002,39.25)) ;
#99652=CARTESIAN_POINT('',(46.65,-19.75,39.25)) ;
#99653=CARTESIAN_POINT('',(46.35,-5.10000000000002,39.25)) ;
#99654=CARTESIAN_POINT('Origin',(46.35,-5.40000000000002,39.25)) ;
#99655=CARTESIAN_POINT('',(43.65,-5.10000000000002,39.25)) ;
#99656=CARTESIAN_POINT('',(53.25,-5.10000000000002,39.25)) ;
#99657=CARTESIAN_POINT('',(43.35,-5.40000000000002,39.25)) ;
#99658=CARTESIAN_POINT('Origin',(43.65,-5.40000000000002,39.25)) ;
#99659=CARTESIAN_POINT('',(43.35,-15.1,39.25)) ;
#99660=CARTESIAN_POINT('',(43.35,-19.75,39.25)) ;
#99661=CARTESIAN_POINT('',(43.65,-15.4,39.25)) ;
#99662=CARTESIAN_POINT('Origin',(43.65,-15.1,39.25)) ;
#99663=CARTESIAN_POINT('',(53.25,-15.4,39.25)) ;
#99664=CARTESIAN_POINT('',(40.65,-15.1,39.25)) ;
#99665=CARTESIAN_POINT('',(40.35,-15.4,39.25)) ;
#99666=CARTESIAN_POINT('Origin',(40.35,-15.1,39.25)) ;
#99667=CARTESIAN_POINT('',(40.65,-5.40000000000002,39.25)) ;
#99668=CARTESIAN_POINT('',(40.65,-19.75,39.25)) ;
#99669=CARTESIAN_POINT('',(40.35,-5.10000000000002,39.25)) ;
#99670=CARTESIAN_POINT('Origin',(40.35,-5.40000000000002,39.25)) ;
#99671=CARTESIAN_POINT('',(37.65,-5.10000000000002,39.25)) ;
#99672=CARTESIAN_POINT('',(53.25,-5.10000000000002,39.25)) ;
#99673=CARTESIAN_POINT('',(37.35,-5.40000000000002,39.25)) ;
#99674=CARTESIAN_POINT('Origin',(37.65,-5.40000000000002,39.25)) ;
#99675=CARTESIAN_POINT('',(37.35,-15.1,39.25)) ;
#99676=CARTESIAN_POINT('',(37.35,-19.75,39.25)) ;
#99677=CARTESIAN_POINT('',(37.65,-15.4,39.25)) ;
#99678=CARTESIAN_POINT('Origin',(37.65,-15.1,39.25)) ;
#99679=CARTESIAN_POINT('',(53.25,-15.4,39.25)) ;
#99680=CARTESIAN_POINT('',(28.65,-15.1,39.25)) ;
#99681=CARTESIAN_POINT('',(28.35,-15.4,39.25)) ;
#99682=CARTESIAN_POINT('Origin',(28.35,-15.1,39.25)) ;
#99683=CARTESIAN_POINT('',(28.65,-5.40000000000002,39.25)) ;
#99684=CARTESIAN_POINT('',(28.65,-19.75,39.25)) ;
#99685=CARTESIAN_POINT('',(28.35,-5.10000000000002,39.25)) ;
#99686=CARTESIAN_POINT('Origin',(28.35,-5.40000000000002,39.25)) ;
#99687=CARTESIAN_POINT('',(25.65,-5.10000000000002,39.25)) ;
#99688=CARTESIAN_POINT('',(53.25,-5.10000000000002,39.25)) ;
#99689=CARTESIAN_POINT('',(25.35,-5.40000000000002,39.25)) ;
#99690=CARTESIAN_POINT('Origin',(25.65,-5.40000000000002,39.25)) ;
#99691=CARTESIAN_POINT('',(25.35,-15.1,39.25)) ;
#99692=CARTESIAN_POINT('',(25.35,-19.75,39.25)) ;
#99693=CARTESIAN_POINT('',(25.65,-15.4,39.25)) ;
#99694=CARTESIAN_POINT('Origin',(25.65,-15.1,39.25)) ;
#99695=CARTESIAN_POINT('',(53.25,-15.4,39.25)) ;
#99696=CARTESIAN_POINT('',(13.35,-5.40000000000002,39.25)) ;
#99697=CARTESIAN_POINT('',(13.65,-5.10000000000002,39.25)) ;
#99698=CARTESIAN_POINT('Origin',(13.65,-5.40000000000002,39.25)) ;
#99699=CARTESIAN_POINT('',(13.35,-15.1,39.25)) ;
#99700=CARTESIAN_POINT('',(13.35,-19.75,39.25)) ;
#99701=CARTESIAN_POINT('',(13.65,-15.4,39.25)) ;
#99702=CARTESIAN_POINT('Origin',(13.65,-15.1,39.25)) ;
#99703=CARTESIAN_POINT('',(16.35,-15.4,39.25)) ;
#99704=CARTESIAN_POINT('',(53.25,-15.4,39.25)) ;
#99705=CARTESIAN_POINT('',(16.65,-15.1,39.25)) ;
#99706=CARTESIAN_POINT('Origin',(16.35,-15.1,39.25)) ;
#99707=CARTESIAN_POINT('',(16.65,-5.40000000000002,39.25)) ;
#99708=CARTESIAN_POINT('',(16.65,-19.75,39.25)) ;
#99709=CARTESIAN_POINT('',(16.35,-5.10000000000002,39.25)) ;
#99710=CARTESIAN_POINT('Origin',(16.35,-5.40000000000002,39.25)) ;
#99711=CARTESIAN_POINT('',(53.25,-5.10000000000002,39.25)) ;
#99712=CARTESIAN_POINT('Origin',(53.25,-2.77555756156289E-14,40.)) ;
#99713=CARTESIAN_POINT('',(0.149999999999965,-2.30070076519351E-14,14.15)) ;
#99714=CARTESIAN_POINT('',(-0.150000000000035,-2.29518985459734E-14,13.85)) ;
#99715=CARTESIAN_POINT('Origin',(-0.150000000000035,-2.30121911110048E-14,
14.15)) ;
#99716=CARTESIAN_POINT('',(0.149999999999963,-2.77555756156289E-14,38.25)) ;
#99717=CARTESIAN_POINT('',(0.149999999999963,-2.77555756156289E-14,40.)) ;
#99718=CARTESIAN_POINT('',(52.25,1.95156391047391E-15,38.25)) ;
#99719=CARTESIAN_POINT('',(53.25,-2.77555756156289E-14,38.25)) ;
#99720=CARTESIAN_POINT('',(52.25,-1.38777878078145E-14,-38.25)) ;
#99721=CARTESIAN_POINT('',(52.25,-1.38777878078145E-14,38.25)) ;
#99722=CARTESIAN_POINT('',(0.149999999999963,-1.38777878078145E-14,-38.25)) ;
#99723=CARTESIAN_POINT('',(53.25,-1.38777878078145E-14,-38.25)) ;
#99724=CARTESIAN_POINT('',(0.149999999999965,-1.78083819895545E-14,-14.15)) ;
#99725=CARTESIAN_POINT('',(0.149999999999963,-2.77555756156289E-14,40.)) ;
#99726=CARTESIAN_POINT('',(-0.150000000000035,-1.78634910955162E-14,-13.85)) ;
#99727=CARTESIAN_POINT('Origin',(-0.150000000000035,-1.78080206830744E-14,
-14.15)) ;
#99728=CARTESIAN_POINT('',(-1.85000000000004,-1.78634910955162E-14,-13.85)) ;
#99729=CARTESIAN_POINT('',(53.25,-1.78634910955162E-14,-13.85)) ;
#99730=CARTESIAN_POINT('',(-1.85000000000004,-2.29518985459734E-14,13.85)) ;
#99731=CARTESIAN_POINT('',(-1.85000000000004,-2.77555756156289E-14,40.)) ;
#99732=CARTESIAN_POINT('',(53.25,-2.29518985459734E-14,13.85)) ;
#99733=CARTESIAN_POINT('Origin',(53.25,-0.750000000000028,40.)) ;
#99734=CARTESIAN_POINT('',(52.25,-0.749999999999998,38.25)) ;
#99735=CARTESIAN_POINT('',(0.149999999999963,-0.750000000000028,38.25)) ;
#99736=CARTESIAN_POINT('',(53.25,-0.750000000000028,38.25)) ;
#99737=CARTESIAN_POINT('',(0.149999999999963,-0.750000000000024,14.15)) ;
#99738=CARTESIAN_POINT('',(0.149999999999963,-0.750000000000024,14.)) ;
#99739=CARTESIAN_POINT('',(-0.150000000000035,-0.750000000000024,13.85)) ;
#99740=CARTESIAN_POINT('Origin',(-0.150000000000035,-0.750000000000024,
14.15)) ;
#99741=CARTESIAN_POINT('',(-1.85000000000004,-0.750000000000024,13.85)) ;
#99742=CARTESIAN_POINT('',(-2.00000000000004,-0.750000000000024,13.85)) ;
#99743=CARTESIAN_POINT('',(-1.85000000000004,-0.750000000000019,-13.85)) ;
#99744=CARTESIAN_POINT('',(-1.85000000000004,-0.750000000000019,-14.)) ;
#99745=CARTESIAN_POINT('',(-0.150000000000035,-0.750000000000019,-13.85)) ;
#99746=CARTESIAN_POINT('',(-4.85722573273506E-14,-0.750000000000019,-13.85)) ;
#99747=CARTESIAN_POINT('',(0.149999999999963,-0.750000000000018,-14.15)) ;
#99748=CARTESIAN_POINT('Origin',(-0.150000000000035,-0.750000000000018,
-14.15)) ;
#99749=CARTESIAN_POINT('',(0.149999999999963,-0.750000000000015,-38.25)) ;
#99750=CARTESIAN_POINT('',(0.149999999999963,-0.750000000000014,-38.25)) ;
#99751=CARTESIAN_POINT('',(52.25,-0.750000000000014,-38.25)) ;
#99752=CARTESIAN_POINT('',(53.25,-0.750000000000015,-38.25)) ;
#99753=CARTESIAN_POINT('',(52.25,-0.750000000000015,38.25)) ;
#99754=CARTESIAN_POINT('Origin',(-3.46944695195361E-14,-1.75,-39.25)) ;
#99755=CARTESIAN_POINT('',(-3.46944695195361E-14,-0.150000000000013,-38.25)) ;
#99756=CARTESIAN_POINT('',(-3.46944695195361E-14,-0.600000000000014,-38.25)) ;
#99757=CARTESIAN_POINT('',(-3.46944695195361E-14,0.,-38.25)) ;
#99758=CARTESIAN_POINT('',(-3.46944695195361E-14,-0.600000000000019,-14.15)) ;
#99759=CARTESIAN_POINT('',(-3.46944695195361E-14,-0.600000000000019,-14.)) ;
#99760=CARTESIAN_POINT('',(-3.46944695195361E-14,-0.150000000000018,-14.15)) ;
#99761=CARTESIAN_POINT('',(-3.46944695195361E-14,-1.38777878078145E-14,
-14.15)) ;
#99762=CARTESIAN_POINT('',(-3.46944695195361E-14,-0.150000000000013,-39.25)) ;
#99763=CARTESIAN_POINT('Origin',(-3.46944695195361E-14,-1.75,-39.25)) ;
#99764=CARTESIAN_POINT('',(-3.46944695195361E-14,-0.150000000000023,14.15)) ;
#99765=CARTESIAN_POINT('',(-3.46944695195361E-14,-0.600000000000024,14.15)) ;
#99766=CARTESIAN_POINT('',(-3.46944695195361E-14,-0.750000000000015,14.15)) ;
#99767=CARTESIAN_POINT('',(-3.46944695195361E-14,-0.600000000000028,38.25)) ;
#99768=CARTESIAN_POINT('',(-3.46944695195361E-14,-0.600000000000028,38.25)) ;
#99769=CARTESIAN_POINT('',(-3.46944695195361E-14,-0.150000000000027,38.25)) ;
#99770=CARTESIAN_POINT('',(-3.46944695195361E-14,-0.750000000000015,38.25)) ;
#99771=CARTESIAN_POINT('',(-3.46944695195361E-14,-0.150000000000013,-39.25)) ;
#99772=CARTESIAN_POINT('Origin',(-2.00000000000004,-0.750000000000028,14.)) ;
#99773=CARTESIAN_POINT('',(-2.00000000000004,-0.600000000000019,-13.85)) ;
#99774=CARTESIAN_POINT('',(-2.00000000000004,-0.600000000000024,13.85)) ;
#99775=CARTESIAN_POINT('',(-2.00000000000004,-0.600000000000024,14.)) ;
#99776=CARTESIAN_POINT('',(-2.00000000000004,-0.150000000000023,13.85)) ;
#99777=CARTESIAN_POINT('',(-2.00000000000004,-0.750000000000028,13.85)) ;
#99778=CARTESIAN_POINT('',(-2.00000000000004,-0.150000000000018,-13.85)) ;
#99779=CARTESIAN_POINT('',(-2.00000000000004,-0.150000000000023,14.)) ;
#99780=CARTESIAN_POINT('',(-2.00000000000004,-0.750000000000023,-13.85)) ;
#99781=CARTESIAN_POINT('Origin',(-4.85722573273506E-14,-0.750000000000015,
-14.)) ;
#99782=CARTESIAN_POINT('',(-0.150000000000035,-0.600000000000019,-14.)) ;
#99783=CARTESIAN_POINT('',(-1.85000000000004,-0.600000000000019,-14.)) ;
#99784=CARTESIAN_POINT('',(-2.00000000000005,-0.600000000000019,-14.)) ;
#99785=CARTESIAN_POINT('',(-1.85000000000004,-0.150000000000018,-14.)) ;
#99786=CARTESIAN_POINT('',(-1.85000000000004,-0.750000000000015,-14.)) ;
#99787=CARTESIAN_POINT('',(-0.150000000000035,-0.150000000000018,-14.)) ;
#99788=CARTESIAN_POINT('',(-4.85722573273506E-14,-0.150000000000018,-14.)) ;
#99789=CARTESIAN_POINT('',(-0.150000000000035,-0.750000000000008,-14.)) ;
#99790=CARTESIAN_POINT('Origin',(-3.46944695195361E-14,-0.750000000000015,
14.)) ;
#99791=CARTESIAN_POINT('',(-1.85000000000004,-0.600000000000024,14.)) ;
#99792=CARTESIAN_POINT('',(-0.150000000000035,-0.600000000000024,14.)) ;
#99793=CARTESIAN_POINT('',(-3.46944695195361E-14,-0.600000000000024,14.)) ;
#99794=CARTESIAN_POINT('',(-0.150000000000035,-0.150000000000023,14.)) ;
#99795=CARTESIAN_POINT('',(-0.150000000000035,-1.38502332548336E-14,14.)) ;
#99796=CARTESIAN_POINT('',(-1.85000000000004,-0.150000000000023,14.)) ;
#99797=CARTESIAN_POINT('',(-3.46944695195361E-14,-0.150000000000023,14.)) ;
#99798=CARTESIAN_POINT('',(-1.85000000000004,-0.750000000000015,14.)) ;
#99799=CARTESIAN_POINT('Origin',(-3.46944695195361E-14,-1.75000000000002,
38.25)) ;
#99800=CARTESIAN_POINT('',(-3.46944695195361E-14,-1.75000000000001,39.4)) ;
#99801=CARTESIAN_POINT('Origin',(-3.46944695195361E-14,-1.75000000000003,
38.25)) ;
#99802=CARTESIAN_POINT('',(-3.46944695195361E-14,-1.75000000000001,39.85)) ;
#99803=CARTESIAN_POINT('',(-3.46944695195361E-14,-1.75000000000001,40.)) ;
#99804=CARTESIAN_POINT('Origin',(-3.46944695195361E-14,-1.75000000000003,
38.25)) ;
#99805=CARTESIAN_POINT('Origin',(52.25,-1.75000000000002,38.25)) ;
#99806=CARTESIAN_POINT('Origin',(52.25,-1.75000000000002,38.25)) ;
#99807=CARTESIAN_POINT('',(52.25,-0.750000000000015,38.25)) ;
#99808=CARTESIAN_POINT('Origin',(52.25,-1.75000000000002,38.25)) ;
#99809=CARTESIAN_POINT('',(52.25,-1.75000000000001,40.)) ;
#99810=CARTESIAN_POINT('Origin',(-26.1749993327458,-1.75000000000003,38.25)) ;
#99811=CARTESIAN_POINT('Origin',(0.149999999999966,-1.75000000000003,38.25)) ;
#99812=CARTESIAN_POINT('Origin',(-26.1749993327458,-1.75000000000003,38.25)) ;
#99813=CARTESIAN_POINT('Origin',(0.149999999999966,-1.75000000000003,38.25)) ;
#99814=CARTESIAN_POINT('Origin',(53.25,-19.75,39.25)) ;
#99815=CARTESIAN_POINT('',(0.149999999999972,-19.75,39.85)) ;
#99816=CARTESIAN_POINT('',(0.149999999999972,-19.75,39.4)) ;
#99817=CARTESIAN_POINT('',(0.14999999999997,-19.75,39.25)) ;
#99818=CARTESIAN_POINT('',(53.,-19.75,39.4)) ;
#99819=CARTESIAN_POINT('',(53.15,-19.75,39.4)) ;
#99820=CARTESIAN_POINT('',(53.,-19.75,39.85)) ;
#99821=CARTESIAN_POINT('',(53.,-19.75,40.)) ;
#99822=CARTESIAN_POINT('',(53.25,-19.75,39.85)) ;
#99823=CARTESIAN_POINT('Origin',(-2.77555756156289E-14,-0.750000000000015,
38.25)) ;
#99824=CARTESIAN_POINT('',(-2.77555756156289E-14,-6.90000000000001,39.4)) ;
#99825=CARTESIAN_POINT('',(-2.77555756156289E-14,-19.6,39.4)) ;
#99826=CARTESIAN_POINT('',(-2.77555756156289E-14,-19.75,39.4)) ;
#99827=CARTESIAN_POINT('',(-2.77555756156289E-14,-19.6,39.85)) ;
#99828=CARTESIAN_POINT('',(-2.77555756156289E-14,-19.6,38.25)) ;
#99829=CARTESIAN_POINT('',(-2.77555756156289E-14,-6.90000000000001,39.85)) ;
#99830=CARTESIAN_POINT('',(-2.77555756156289E-14,-0.750000000000015,39.85)) ;
#99831=CARTESIAN_POINT('',(-2.77555756156289E-14,-6.90000000000001,39.25)) ;
#99832=CARTESIAN_POINT('Origin',(-2.77555756156289E-14,-6.75000000000001,
39.25)) ;
#99833=CARTESIAN_POINT('',(-1.85000000000003,-6.75000000000001,39.4)) ;
#99834=CARTESIAN_POINT('',(-0.150000000000028,-6.75000000000001,39.4)) ;
#99835=CARTESIAN_POINT('',(-2.77555756156289E-14,-6.75000000000001,39.4)) ;
#99836=CARTESIAN_POINT('',(-0.150000000000028,-6.75000000000001,39.85)) ;
#99837=CARTESIAN_POINT('',(-0.150000000000028,-6.75000000000001,40.)) ;
#99838=CARTESIAN_POINT('',(-1.85000000000003,-6.75000000000001,39.85)) ;
#99839=CARTESIAN_POINT('',(-2.77555756156289E-14,-6.75000000000001,39.85)) ;
#99840=CARTESIAN_POINT('',(-1.85000000000003,-6.75000000000001,39.25)) ;
#99841=CARTESIAN_POINT('Origin',(-2.00000000000003,-4.75000000000002,39.25)) ;
#99842=CARTESIAN_POINT('',(-2.00000000000003,-4.90000000000001,39.4)) ;
#99843=CARTESIAN_POINT('',(-2.00000000000003,-6.60000000000001,39.4)) ;
#99844=CARTESIAN_POINT('',(-2.00000000000003,-6.75000000000002,39.4)) ;
#99845=CARTESIAN_POINT('',(-2.00000000000003,-6.60000000000001,39.85)) ;
#99846=CARTESIAN_POINT('',(-2.00000000000003,-6.60000000000001,39.25)) ;
#99847=CARTESIAN_POINT('',(-2.00000000000003,-4.90000000000001,39.85)) ;
#99848=CARTESIAN_POINT('',(-2.00000000000003,-4.75000000000002,39.85)) ;
#99849=CARTESIAN_POINT('',(-2.00000000000003,-4.90000000000001,39.25)) ;
#99850=CARTESIAN_POINT('Origin',(-2.77555756156289E-14,-4.75000000000001,
39.25)) ;
#99851=CARTESIAN_POINT('',(-0.150000000000028,-4.75000000000001,39.4)) ;
#99852=CARTESIAN_POINT('',(-1.85000000000003,-4.75000000000001,39.4)) ;
#99853=CARTESIAN_POINT('',(-2.00000000000003,-4.75000000000001,39.4)) ;
#99854=CARTESIAN_POINT('',(-1.85000000000003,-4.75000000000001,39.85)) ;
#99855=CARTESIAN_POINT('',(-1.85000000000003,-4.75000000000001,39.25)) ;
#99856=CARTESIAN_POINT('',(-0.150000000000028,-4.75000000000001,39.85)) ;
#99857=CARTESIAN_POINT('',(-2.77555756156289E-14,-4.75000000000001,39.85)) ;
#99858=CARTESIAN_POINT('',(-0.150000000000028,-4.75000000000001,39.25)) ;
#99859=CARTESIAN_POINT('Origin',(53.1499999999998,56.3581964958473,39.25)) ;
#99860=CARTESIAN_POINT('',(53.15,-1.90000000000001,39.85)) ;
#99861=CARTESIAN_POINT('',(53.15,-19.6,39.85)) ;
#99862=CARTESIAN_POINT('',(53.15,-19.75,39.85)) ;
#99863=CARTESIAN_POINT('',(53.15,-19.6,39.4)) ;
#99864=CARTESIAN_POINT('',(53.15,-19.6,39.25)) ;
#99865=CARTESIAN_POINT('',(53.15,-1.90000000000001,39.4)) ;
#99866=CARTESIAN_POINT('',(53.1499999999998,56.3581964958473,39.4)) ;
#99867=CARTESIAN_POINT('',(53.15,-1.90000000000001,40.)) ;
#99868=CARTESIAN_POINT('Origin',(-2.77555756156289E-14,-0.750000000000015,
38.25)) ;
#99869=CARTESIAN_POINT('',(-2.77555756156289E-14,-4.60000000000001,39.4)) ;
#99870=CARTESIAN_POINT('',(-2.77555756156289E-14,-4.75000000000001,39.4)) ;
#99871=CARTESIAN_POINT('',(-2.77555756156289E-14,-4.60000000000001,39.85)) ;
#99872=CARTESIAN_POINT('',(-2.77555756156289E-14,-4.60000000000001,40.)) ;
#99873=CARTESIAN_POINT('',(-2.77555756156289E-14,-0.750000000000015,39.85)) ;
#99874=CARTESIAN_POINT('Origin',(-3.46944695195361E-14,-1.75000000000002,
7.18201007936591E-15)) ;
#99875=CARTESIAN_POINT('',(53.,-1.75000000000001,39.25)) ;
#99876=CARTESIAN_POINT('Origin',(54.,-1.74999999999998,-40.)) ;
#99877=CARTESIAN_POINT('',(53.85,-1.89999999999998,-40.)) ;
#99878=CARTESIAN_POINT('',(53.8500000000001,-19.6,-40.)) ;
#99879=CARTESIAN_POINT('',(53.8500000000001,-19.75,-40.)) ;
#99880=CARTESIAN_POINT('',(53.4000000000001,-19.6,-40.)) ;
#99881=CARTESIAN_POINT('',(53.2500000000001,-19.6,-40.)) ;
#99882=CARTESIAN_POINT('',(53.4,-1.89999999999998,-40.)) ;
#99883=CARTESIAN_POINT('',(53.4,-1.74999999999998,-40.)) ;
#99884=CARTESIAN_POINT('',(54.,-1.89999999999998,-40.)) ;
#99885=CARTESIAN_POINT('Origin',(54.0000000000001,-19.75,-38.25)) ;
#99886=CARTESIAN_POINT('',(53.8500000000001,-19.75,-39.85)) ;
#99887=CARTESIAN_POINT('',(53.8500000000001,-19.75,39.85)) ;
#99888=CARTESIAN_POINT('',(53.8500000000001,-19.75,-38.25)) ;
#99889=CARTESIAN_POINT('',(53.4000000000001,-19.75,39.85)) ;
#99890=CARTESIAN_POINT('',(54.0000000000001,-19.75,39.85)) ;
#99891=CARTESIAN_POINT('',(53.4000000000001,-19.75,-39.85)) ;
#99892=CARTESIAN_POINT('',(53.4000000000001,-19.75,-40.)) ;
#99893=CARTESIAN_POINT('',(54.0000000000001,-19.75,-39.85)) ;
#99894=CARTESIAN_POINT('Origin',(54.,-1.74999999999999,40.)) ;
#99895=CARTESIAN_POINT('',(53.8500000000001,-19.6,40.)) ;
#99896=CARTESIAN_POINT('',(53.85,-1.89999999999999,40.)) ;
#99897=CARTESIAN_POINT('',(53.85,-1.74999999999999,40.)) ;
#99898=CARTESIAN_POINT('',(53.4,-1.9,40.)) ;
#99899=CARTESIAN_POINT('',(54.,-1.89999999999999,40.)) ;
#99900=CARTESIAN_POINT('',(53.4000000000001,-19.6,40.)) ;
#99901=CARTESIAN_POINT('',(53.4000000000001,-19.75,40.)) ;
#99902=CARTESIAN_POINT('',(54.0000000000001,-19.6,40.)) ;
#99903=CARTESIAN_POINT('Origin',(54.,-1.74999999999999,38.25)) ;
#99904=CARTESIAN_POINT('',(54.,-1.74999999999999,39.85)) ;
#99905=CARTESIAN_POINT('',(53.25,-1.74999999999999,38.25)) ;
#99906=CARTESIAN_POINT('Origin',(54.,-1.74999999999998,-38.25)) ;
#99907=CARTESIAN_POINT('',(54.,-1.74999999999998,-39.85)) ;
#99908=CARTESIAN_POINT('',(53.25,-1.74999999999998,-38.25)) ;
#99909=CARTESIAN_POINT('Origin',(52.25,-1.74999999999998,-38.25)) ;
#99910=CARTESIAN_POINT('Origin',(52.25,-1.74999999999998,-38.25)) ;
#99911=CARTESIAN_POINT('',(52.25,-0.750000000000001,-38.25)) ;
#99912=CARTESIAN_POINT('Origin',(52.25,-1.74999999999998,-38.25)) ;
#99913=CARTESIAN_POINT('Origin',(52.25,-1.75,38.25)) ;
#99914=CARTESIAN_POINT('Origin',(52.25,-1.75,38.25)) ;
#99915=CARTESIAN_POINT('Origin',(52.25,-1.75,38.25)) ;
#99916=CARTESIAN_POINT('Origin',(52.25,-1.74999999999998,-76.5341585842897)) ;
#99917=CARTESIAN_POINT('Origin',(52.25,-1.74999999999998,-76.5341585842897)) ;
#99918=CARTESIAN_POINT('Origin',(-2.77555756156289E-14,-1.75000000000001,
-38.25)) ;
#99919=CARTESIAN_POINT('',(-3.46944695195361E-14,-1.74999999999999,-39.4)) ;
#99920=CARTESIAN_POINT('',(-3.46944695195361E-14,-1.74999999999999,-39.85)) ;
#99921=CARTESIAN_POINT('',(-3.46944695195361E-14,-1.74999999999999,-39.25)) ;
#99922=CARTESIAN_POINT('Origin',(-2.77555756156289E-14,-1.75000000000001,
-38.25)) ;
#99923=CARTESIAN_POINT('Origin',(-2.77555756156289E-14,-1.75000000000001,
-38.25)) ;
#99924=CARTESIAN_POINT('Origin',(52.25,-1.75000000000001,-38.25)) ;
#99925=CARTESIAN_POINT('Origin',(52.25,-1.75000000000001,-38.25)) ;
#99926=CARTESIAN_POINT('',(52.25,-1.74999999999999,-39.25)) ;
#99927=CARTESIAN_POINT('Origin',(52.25,-1.75000000000001,-38.25)) ;
#99928=CARTESIAN_POINT('Origin',(78.4249993327457,-1.75000000000001,-38.25)) ;
#99929=CARTESIAN_POINT('Origin',(0.14999999999997,-1.75000000000001,-38.25)) ;
#99930=CARTESIAN_POINT('Origin',(78.4249993327457,-1.75000000000001,-38.25)) ;
#99931=CARTESIAN_POINT('Origin',(0.14999999999997,-1.75000000000001,-38.25)) ;
#99932=CARTESIAN_POINT('Origin',(-2.77555756156289E-14,-4.75,-39.25)) ;
#99933=CARTESIAN_POINT('',(-1.85000000000003,-4.75,-39.4)) ;
#99934=CARTESIAN_POINT('',(-0.150000000000035,-4.75,-39.4)) ;
#99935=CARTESIAN_POINT('',(-2.77555756156289E-14,-4.75,-39.4)) ;
#99936=CARTESIAN_POINT('',(-0.150000000000035,-4.75,-39.85)) ;
#99937=CARTESIAN_POINT('',(-0.150000000000035,-4.75,-40.)) ;
#99938=CARTESIAN_POINT('',(-1.85000000000003,-4.75,-39.85)) ;
#99939=CARTESIAN_POINT('',(-2.00000000000003,-4.75,-39.85)) ;
#99940=CARTESIAN_POINT('',(-1.85000000000003,-4.75,-39.25)) ;
#99941=CARTESIAN_POINT('Origin',(-2.00000000000003,-4.75000000000001,-39.25)) ;
#99942=CARTESIAN_POINT('',(-2.00000000000003,-6.60000000000001,-39.4)) ;
#99943=CARTESIAN_POINT('',(-2.00000000000003,-4.9,-39.4)) ;
#99944=CARTESIAN_POINT('',(-2.00000000000003,-4.75000000000001,-39.4)) ;
#99945=CARTESIAN_POINT('',(-2.00000000000003,-4.9,-39.85)) ;
#99946=CARTESIAN_POINT('',(-2.00000000000003,-4.9,-39.25)) ;
#99947=CARTESIAN_POINT('',(-2.00000000000003,-6.60000000000001,-39.85)) ;
#99948=CARTESIAN_POINT('',(-2.00000000000003,-6.75000000000001,-39.85)) ;
#99949=CARTESIAN_POINT('',(-2.00000000000003,-6.60000000000001,-39.25)) ;
#99950=CARTESIAN_POINT('Origin',(-3.46944695195361E-14,-6.75000000000001,
-39.25)) ;
#99951=CARTESIAN_POINT('',(-0.150000000000035,-6.75000000000001,-39.4)) ;
#99952=CARTESIAN_POINT('',(-1.85000000000003,-6.75000000000001,-39.4)) ;
#99953=CARTESIAN_POINT('',(-3.46944695195361E-14,-6.75000000000001,-39.4)) ;
#99954=CARTESIAN_POINT('',(-1.85000000000003,-6.75000000000001,-39.85)) ;
#99955=CARTESIAN_POINT('',(-1.85000000000003,-6.75000000000001,-39.25)) ;
#99956=CARTESIAN_POINT('',(-0.150000000000035,-6.75000000000001,-39.85)) ;
#99957=CARTESIAN_POINT('',(-3.46944695195361E-14,-6.75000000000001,-39.85)) ;
#99958=CARTESIAN_POINT('',(-0.150000000000035,-6.75000000000001,-39.25)) ;
#99959=CARTESIAN_POINT('Origin',(-3.46944695195361E-14,-1.74999999999999,
-38.25)) ;
#99960=CARTESIAN_POINT('',(-3.46944695195361E-14,-19.6,-39.4)) ;
#99961=CARTESIAN_POINT('',(-3.46944695195361E-14,-6.90000000000001,-39.4)) ;
#99962=CARTESIAN_POINT('',(-3.46944695195361E-14,-1.74999999999999,-39.4)) ;
#99963=CARTESIAN_POINT('',(-3.46944695195361E-14,-6.90000000000001,-39.85)) ;
#99964=CARTESIAN_POINT('',(-3.46944695195361E-14,-6.90000000000001,-40.)) ;
#99965=CARTESIAN_POINT('',(-3.46944695195361E-14,-19.6,-39.85)) ;
#99966=CARTESIAN_POINT('',(-3.46944695195361E-14,-19.75,-39.85)) ;
#99967=CARTESIAN_POINT('',(-3.46944695195361E-14,-19.6,-39.25)) ;
#99968=CARTESIAN_POINT('Origin',(53.25,-19.75,-40.)) ;
#99969=CARTESIAN_POINT('',(53.0000000000001,-19.75,-39.4)) ;
#99970=CARTESIAN_POINT('',(0.149999999999965,-19.75,-39.4)) ;
#99971=CARTESIAN_POINT('',(-2.77555756156289E-14,-19.75,-39.4)) ;
#99972=CARTESIAN_POINT('',(0.149999999999965,-19.75,-39.85)) ;
#99973=CARTESIAN_POINT('',(0.149999999999965,-19.75,-40.)) ;
#99974=CARTESIAN_POINT('',(53.0000000000001,-19.75,-39.85)) ;
#99975=CARTESIAN_POINT('',(53.25,-19.75,-39.85)) ;
#99976=CARTESIAN_POINT('',(53.0000000000001,-19.75,-40.)) ;
#99977=CARTESIAN_POINT('Origin',(53.1499999999998,56.3581964958473,-39.25)) ;
#99978=CARTESIAN_POINT('',(53.1500000000001,-19.6,-39.4)) ;
#99979=CARTESIAN_POINT('',(53.1500000000001,-19.6,-39.85)) ;
#99980=CARTESIAN_POINT('',(53.1500000000001,-19.6,-39.25)) ;
#99981=CARTESIAN_POINT('',(53.15,-1.89999999999998,-39.85)) ;
#99982=CARTESIAN_POINT('',(53.1499999999998,56.3581964958473,-39.85)) ;
#99983=CARTESIAN_POINT('',(53.15,-1.89999999999998,-39.4)) ;
#99984=CARTESIAN_POINT('',(53.15,-1.89999999999999,-39.25)) ;
#99985=CARTESIAN_POINT('',(53.1500000000001,-19.75,-39.4)) ;
#99986=CARTESIAN_POINT('Origin',(-3.46944695195361E-14,-1.75000000000002,
-1.38777878078145E-14)) ;
#99987=CARTESIAN_POINT('',(53.,-1.75000000000002,-1.38777878078145E-14)) ;
#99988=CARTESIAN_POINT('Origin',(-3.46944695195361E-14,-1.74999999999999,
-38.25)) ;
#99989=CARTESIAN_POINT('',(-3.46944695195361E-14,-4.6,-39.85)) ;
#99990=CARTESIAN_POINT('',(-3.46944695195361E-14,-4.6,-39.4)) ;
#99991=CARTESIAN_POINT('',(-3.46944695195361E-14,-4.6,-39.25)) ;
#99992=CARTESIAN_POINT('',(-3.46944695195361E-14,-1.74999999999999,-39.4)) ;
#99993=CARTESIAN_POINT('',(-3.46944695195361E-14,-4.75,-39.85)) ;
#99994=CARTESIAN_POINT('Origin',(43.5,-15.25,-40.001)) ;
#99995=CARTESIAN_POINT('',(43.65,-15.25,39.85)) ;
#99996=CARTESIAN_POINT('',(46.35,-15.25,39.85)) ;
#99997=CARTESIAN_POINT('',(46.5,-15.25,39.85)) ;
#99998=CARTESIAN_POINT('',(46.35,-15.25,39.4)) ;
#99999=CARTESIAN_POINT('',(46.35,-15.25,39.25)) ;
#100000=CARTESIAN_POINT('',(43.65,-15.25,39.4)) ;
#100001=CARTESIAN_POINT('',(43.5,-15.25,39.4)) ;
#100002=CARTESIAN_POINT('',(43.65,-15.25,40.)) ;
#100003=CARTESIAN_POINT('Origin',(43.5,-5.25000000000002,-40.001)) ;
#100004=CARTESIAN_POINT('',(43.5,-5.40000000000002,39.85)) ;
#100005=CARTESIAN_POINT('',(43.5,-15.1,39.85)) ;
#100006=CARTESIAN_POINT('',(43.5,-15.25,39.85)) ;
#100007=CARTESIAN_POINT('',(43.5,-15.1,39.4)) ;
#100008=CARTESIAN_POINT('',(43.5,-15.1,39.25)) ;
#100009=CARTESIAN_POINT('',(43.5,-5.40000000000002,39.4)) ;
#100010=CARTESIAN_POINT('',(43.5,-5.25000000000002,39.4)) ;
#100011=CARTESIAN_POINT('',(43.5,-5.40000000000002,40.)) ;
#100012=CARTESIAN_POINT('Origin',(43.5,-5.25000000000002,-40.001)) ;
#100013=CARTESIAN_POINT('',(43.65,-5.25000000000002,39.4)) ;
#100014=CARTESIAN_POINT('',(46.35,-5.25000000000002,39.4)) ;
#100015=CARTESIAN_POINT('',(43.5,-5.25000000000002,39.4)) ;
#100016=CARTESIAN_POINT('',(46.35,-5.25000000000002,39.85)) ;
#100017=CARTESIAN_POINT('',(46.35,-5.25000000000002,40.)) ;
#100018=CARTESIAN_POINT('',(43.65,-5.25000000000002,39.85)) ;
#100019=CARTESIAN_POINT('',(43.5,-5.25000000000002,39.85)) ;
#100020=CARTESIAN_POINT('',(43.65,-5.25000000000002,39.25)) ;
#100021=CARTESIAN_POINT('Origin',(46.5,-5.25000000000002,-40.001)) ;
#100022=CARTESIAN_POINT('',(46.5,-15.1,39.85)) ;
#100023=CARTESIAN_POINT('',(46.5,-5.40000000000002,39.85)) ;
#100024=CARTESIAN_POINT('',(46.5,-5.25000000000002,39.85)) ;
#100025=CARTESIAN_POINT('',(46.5,-5.40000000000002,39.4)) ;
#100026=CARTESIAN_POINT('',(46.5,-5.40000000000002,39.25)) ;
#100027=CARTESIAN_POINT('',(46.5,-15.1,39.4)) ;
#100028=CARTESIAN_POINT('',(46.5,-5.25000000000002,39.4)) ;
#100029=CARTESIAN_POINT('',(46.5,-15.1,40.)) ;
#100030=CARTESIAN_POINT('Origin',(37.5,-15.25,-40.001)) ;
#100031=CARTESIAN_POINT('',(37.65,-15.25,39.85)) ;
#100032=CARTESIAN_POINT('',(40.35,-15.25,39.85)) ;
#100033=CARTESIAN_POINT('',(40.5,-15.25,39.85)) ;
#100034=CARTESIAN_POINT('',(40.35,-15.25,39.4)) ;
#100035=CARTESIAN_POINT('',(40.35,-15.25,39.25)) ;
#100036=CARTESIAN_POINT('',(37.65,-15.25,39.4)) ;
#100037=CARTESIAN_POINT('',(37.5,-15.25,39.4)) ;
#100038=CARTESIAN_POINT('',(37.65,-15.25,40.)) ;
#100039=CARTESIAN_POINT('Origin',(37.5,-5.25000000000002,-40.001)) ;
#100040=CARTESIAN_POINT('',(37.5,-5.40000000000002,39.85)) ;
#100041=CARTESIAN_POINT('',(37.5,-15.1,39.85)) ;
#100042=CARTESIAN_POINT('',(37.5,-15.25,39.85)) ;
#100043=CARTESIAN_POINT('',(37.5,-15.1,39.4)) ;
#100044=CARTESIAN_POINT('',(37.5,-15.1,39.25)) ;
#100045=CARTESIAN_POINT('',(37.5,-5.40000000000002,39.4)) ;
#100046=CARTESIAN_POINT('',(37.5,-5.25000000000002,39.4)) ;
#100047=CARTESIAN_POINT('',(37.5,-5.40000000000002,40.)) ;
#100048=CARTESIAN_POINT('Origin',(37.5,-5.25000000000002,-40.001)) ;
#100049=CARTESIAN_POINT('',(37.65,-5.25000000000002,39.4)) ;
#100050=CARTESIAN_POINT('',(40.35,-5.25000000000002,39.4)) ;
#100051=CARTESIAN_POINT('',(37.5,-5.25000000000002,39.4)) ;
#100052=CARTESIAN_POINT('',(40.35,-5.25000000000002,39.85)) ;
#100053=CARTESIAN_POINT('',(40.35,-5.25000000000002,40.)) ;
#100054=CARTESIAN_POINT('',(37.65,-5.25000000000002,39.85)) ;
#100055=CARTESIAN_POINT('',(37.5,-5.25000000000002,39.85)) ;
#100056=CARTESIAN_POINT('',(37.65,-5.25000000000002,39.25)) ;
#100057=CARTESIAN_POINT('Origin',(40.5,-5.25000000000002,-40.001)) ;
#100058=CARTESIAN_POINT('',(40.5,-15.1,39.85)) ;
#100059=CARTESIAN_POINT('',(40.5,-5.40000000000002,39.85)) ;
#100060=CARTESIAN_POINT('',(40.5,-5.25000000000002,39.85)) ;
#100061=CARTESIAN_POINT('',(40.5,-5.40000000000002,39.4)) ;
#100062=CARTESIAN_POINT('',(40.5,-5.40000000000002,39.25)) ;
#100063=CARTESIAN_POINT('',(40.5,-15.1,39.4)) ;
#100064=CARTESIAN_POINT('',(40.5,-5.25000000000002,39.4)) ;
#100065=CARTESIAN_POINT('',(40.5,-15.1,40.)) ;
#100066=CARTESIAN_POINT('Origin',(31.5,-15.25,-40.001)) ;
#100067=CARTESIAN_POINT('',(31.65,-15.25,39.85)) ;
#100068=CARTESIAN_POINT('',(34.35,-15.25,39.85)) ;
#100069=CARTESIAN_POINT('',(34.5,-15.25,39.85)) ;
#100070=CARTESIAN_POINT('',(34.35,-15.25,39.4)) ;
#100071=CARTESIAN_POINT('',(34.35,-15.25,39.25)) ;
#100072=CARTESIAN_POINT('',(31.65,-15.25,39.4)) ;
#100073=CARTESIAN_POINT('',(31.5,-15.25,39.4)) ;
#100074=CARTESIAN_POINT('',(31.65,-15.25,40.)) ;
#100075=CARTESIAN_POINT('Origin',(31.5,-5.25000000000002,-40.001)) ;
#100076=CARTESIAN_POINT('',(31.5,-5.40000000000002,39.85)) ;
#100077=CARTESIAN_POINT('',(31.5,-15.1,39.85)) ;
#100078=CARTESIAN_POINT('',(31.5,-15.25,39.85)) ;
#100079=CARTESIAN_POINT('',(31.5,-15.1,39.4)) ;
#100080=CARTESIAN_POINT('',(31.5,-15.1,39.25)) ;
#100081=CARTESIAN_POINT('',(31.5,-5.40000000000002,39.4)) ;
#100082=CARTESIAN_POINT('',(31.5,-5.25000000000002,39.4)) ;
#100083=CARTESIAN_POINT('',(31.5,-5.40000000000002,40.)) ;
#100084=CARTESIAN_POINT('Origin',(31.5,-5.25000000000002,-40.001)) ;
#100085=CARTESIAN_POINT('',(31.65,-5.25000000000002,39.4)) ;
#100086=CARTESIAN_POINT('',(34.35,-5.25000000000002,39.4)) ;
#100087=CARTESIAN_POINT('',(31.5,-5.25000000000002,39.4)) ;
#100088=CARTESIAN_POINT('',(34.35,-5.25000000000002,39.85)) ;
#100089=CARTESIAN_POINT('',(34.35,-5.25000000000002,40.)) ;
#100090=CARTESIAN_POINT('',(31.65,-5.25000000000002,39.85)) ;
#100091=CARTESIAN_POINT('',(31.5,-5.25000000000002,39.85)) ;
#100092=CARTESIAN_POINT('',(31.65,-5.25000000000002,39.25)) ;
#100093=CARTESIAN_POINT('Origin',(34.5,-5.25000000000002,-40.001)) ;
#100094=CARTESIAN_POINT('',(34.5,-15.1,39.85)) ;
#100095=CARTESIAN_POINT('',(34.5,-5.40000000000002,39.85)) ;
#100096=CARTESIAN_POINT('',(34.5,-5.25000000000002,39.85)) ;
#100097=CARTESIAN_POINT('',(34.5,-5.40000000000002,39.4)) ;
#100098=CARTESIAN_POINT('',(34.5,-5.40000000000002,39.25)) ;
#100099=CARTESIAN_POINT('',(34.5,-15.1,39.4)) ;
#100100=CARTESIAN_POINT('',(34.5,-5.25000000000002,39.4)) ;
#100101=CARTESIAN_POINT('',(34.5,-15.1,40.)) ;
#100102=CARTESIAN_POINT('Origin',(25.5,-15.25,-40.001)) ;
#100103=CARTESIAN_POINT('',(25.65,-15.25,39.85)) ;
#100104=CARTESIAN_POINT('',(28.35,-15.25,39.85)) ;
#100105=CARTESIAN_POINT('',(28.5,-15.25,39.85)) ;
#100106=CARTESIAN_POINT('',(28.35,-15.25,39.4)) ;
#100107=CARTESIAN_POINT('',(28.35,-15.25,39.25)) ;
#100108=CARTESIAN_POINT('',(25.65,-15.25,39.4)) ;
#100109=CARTESIAN_POINT('',(25.5,-15.25,39.4)) ;
#100110=CARTESIAN_POINT('',(25.65,-15.25,40.)) ;
#100111=CARTESIAN_POINT('Origin',(25.5,-5.25000000000002,-40.001)) ;
#100112=CARTESIAN_POINT('',(25.5,-5.40000000000002,39.85)) ;
#100113=CARTESIAN_POINT('',(25.5,-15.1,39.85)) ;
#100114=CARTESIAN_POINT('',(25.5,-15.25,39.85)) ;
#100115=CARTESIAN_POINT('',(25.5,-15.1,39.4)) ;
#100116=CARTESIAN_POINT('',(25.5,-15.1,39.25)) ;
#100117=CARTESIAN_POINT('',(25.5,-5.40000000000002,39.4)) ;
#100118=CARTESIAN_POINT('',(25.5,-5.25000000000002,39.4)) ;
#100119=CARTESIAN_POINT('',(25.5,-5.40000000000002,40.)) ;
#100120=CARTESIAN_POINT('Origin',(25.5,-5.25000000000002,-40.001)) ;
#100121=CARTESIAN_POINT('',(25.65,-5.25000000000002,39.4)) ;
#100122=CARTESIAN_POINT('',(28.35,-5.25000000000002,39.4)) ;
#100123=CARTESIAN_POINT('',(25.5,-5.25000000000002,39.4)) ;
#100124=CARTESIAN_POINT('',(28.35,-5.25000000000002,39.85)) ;
#100125=CARTESIAN_POINT('',(28.35,-5.25000000000002,40.)) ;
#100126=CARTESIAN_POINT('',(25.65,-5.25000000000002,39.85)) ;
#100127=CARTESIAN_POINT('',(25.5,-5.25000000000002,39.85)) ;
#100128=CARTESIAN_POINT('',(25.65,-5.25000000000002,39.25)) ;
#100129=CARTESIAN_POINT('Origin',(28.5,-5.25000000000002,-40.001)) ;
#100130=CARTESIAN_POINT('',(28.5,-15.1,39.85)) ;
#100131=CARTESIAN_POINT('',(28.5,-5.40000000000002,39.85)) ;
#100132=CARTESIAN_POINT('',(28.5,-5.25000000000002,39.85)) ;
#100133=CARTESIAN_POINT('',(28.5,-5.40000000000002,39.4)) ;
#100134=CARTESIAN_POINT('',(28.5,-5.40000000000002,39.25)) ;
#100135=CARTESIAN_POINT('',(28.5,-15.1,39.4)) ;
#100136=CARTESIAN_POINT('',(28.5,-5.25000000000002,39.4)) ;
#100137=CARTESIAN_POINT('',(28.5,-15.1,40.)) ;
#100138=CARTESIAN_POINT('Origin',(19.5,-15.25,-40.001)) ;
#100139=CARTESIAN_POINT('',(19.65,-15.25,39.85)) ;
#100140=CARTESIAN_POINT('',(22.35,-15.25,39.85)) ;
#100141=CARTESIAN_POINT('',(22.5,-15.25,39.85)) ;
#100142=CARTESIAN_POINT('',(22.35,-15.25,39.4)) ;
#100143=CARTESIAN_POINT('',(22.35,-15.25,39.25)) ;
#100144=CARTESIAN_POINT('',(19.65,-15.25,39.4)) ;
#100145=CARTESIAN_POINT('',(19.5,-15.25,39.4)) ;
#100146=CARTESIAN_POINT('',(19.65,-15.25,40.)) ;
#100147=CARTESIAN_POINT('Origin',(19.5,-5.25000000000002,-40.001)) ;
#100148=CARTESIAN_POINT('',(19.5,-5.40000000000002,39.85)) ;
#100149=CARTESIAN_POINT('',(19.5,-15.1,39.85)) ;
#100150=CARTESIAN_POINT('',(19.5,-15.25,39.85)) ;
#100151=CARTESIAN_POINT('',(19.5,-15.1,39.4)) ;
#100152=CARTESIAN_POINT('',(19.5,-15.1,39.25)) ;
#100153=CARTESIAN_POINT('',(19.5,-5.40000000000002,39.4)) ;
#100154=CARTESIAN_POINT('',(19.5,-5.25000000000002,39.4)) ;
#100155=CARTESIAN_POINT('',(19.5,-5.40000000000002,40.)) ;
#100156=CARTESIAN_POINT('Origin',(19.5,-5.25000000000002,-40.001)) ;
#100157=CARTESIAN_POINT('',(19.65,-5.25000000000002,39.4)) ;
#100158=CARTESIAN_POINT('',(22.35,-5.25000000000002,39.4)) ;
#100159=CARTESIAN_POINT('',(19.5,-5.25000000000002,39.4)) ;
#100160=CARTESIAN_POINT('',(22.35,-5.25000000000002,39.85)) ;
#100161=CARTESIAN_POINT('',(22.35,-5.25000000000002,40.)) ;
#100162=CARTESIAN_POINT('',(19.65,-5.25000000000002,39.85)) ;
#100163=CARTESIAN_POINT('',(19.5,-5.25000000000002,39.85)) ;
#100164=CARTESIAN_POINT('',(19.65,-5.25000000000002,39.25)) ;
#100165=CARTESIAN_POINT('Origin',(22.5,-5.25000000000002,-40.001)) ;
#100166=CARTESIAN_POINT('',(22.5,-15.1,39.85)) ;
#100167=CARTESIAN_POINT('',(22.5,-5.40000000000002,39.85)) ;
#100168=CARTESIAN_POINT('',(22.5,-5.25000000000002,39.85)) ;
#100169=CARTESIAN_POINT('',(22.5,-5.40000000000002,39.4)) ;
#100170=CARTESIAN_POINT('',(22.5,-5.40000000000002,39.25)) ;
#100171=CARTESIAN_POINT('',(22.5,-15.1,39.4)) ;
#100172=CARTESIAN_POINT('',(22.5,-5.25000000000002,39.4)) ;
#100173=CARTESIAN_POINT('',(22.5,-15.1,40.)) ;
#100174=CARTESIAN_POINT('Origin',(13.5,-15.25,-40.001)) ;
#100175=CARTESIAN_POINT('',(16.35,-15.25,39.4)) ;
#100176=CARTESIAN_POINT('',(13.65,-15.25,39.4)) ;
#100177=CARTESIAN_POINT('',(13.5,-15.25,39.4)) ;
#100178=CARTESIAN_POINT('',(13.65,-15.25,39.85)) ;
#100179=CARTESIAN_POINT('',(13.65,-15.25,40.)) ;
#100180=CARTESIAN_POINT('',(16.35,-15.25,39.85)) ;
#100181=CARTESIAN_POINT('',(16.5,-15.25,39.85)) ;
#100182=CARTESIAN_POINT('',(16.35,-15.25,39.25)) ;
#100183=CARTESIAN_POINT('Origin',(13.5,-5.25000000000002,-40.001)) ;
#100184=CARTESIAN_POINT('',(13.5,-5.40000000000002,39.85)) ;
#100185=CARTESIAN_POINT('',(13.5,-15.1,39.85)) ;
#100186=CARTESIAN_POINT('',(13.5,-15.25,39.85)) ;
#100187=CARTESIAN_POINT('',(13.5,-15.1,39.4)) ;
#100188=CARTESIAN_POINT('',(13.5,-15.1,39.25)) ;
#100189=CARTESIAN_POINT('',(13.5,-5.40000000000002,39.4)) ;
#100190=CARTESIAN_POINT('',(13.5,-5.25000000000002,39.4)) ;
#100191=CARTESIAN_POINT('',(13.5,-5.40000000000002,40.)) ;
#100192=CARTESIAN_POINT('Origin',(13.5,-5.25000000000002,-40.001)) ;
#100193=CARTESIAN_POINT('',(16.35,-5.25000000000002,39.85)) ;
#100194=CARTESIAN_POINT('',(13.65,-5.25000000000002,39.85)) ;
#100195=CARTESIAN_POINT('',(13.5,-5.25000000000002,39.85)) ;
#100196=CARTESIAN_POINT('',(13.65,-5.25000000000002,39.4)) ;
#100197=CARTESIAN_POINT('',(13.65,-5.25000000000002,39.25)) ;
#100198=CARTESIAN_POINT('',(16.35,-5.25000000000002,39.4)) ;
#100199=CARTESIAN_POINT('',(13.5,-5.25000000000002,39.4)) ;
#100200=CARTESIAN_POINT('',(16.35,-5.25000000000002,40.)) ;
#100201=CARTESIAN_POINT('Origin',(16.5,-5.25000000000002,-40.001)) ;
#100202=CARTESIAN_POINT('',(16.5,-15.1,39.85)) ;
#100203=CARTESIAN_POINT('',(16.5,-5.40000000000002,39.85)) ;
#100204=CARTESIAN_POINT('',(16.5,-5.25000000000002,39.85)) ;
#100205=CARTESIAN_POINT('',(16.5,-5.40000000000002,39.4)) ;
#100206=CARTESIAN_POINT('',(16.5,-5.40000000000002,39.25)) ;
#100207=CARTESIAN_POINT('',(16.5,-15.1,39.4)) ;
#100208=CARTESIAN_POINT('',(16.5,-5.25000000000002,39.4)) ;
#100209=CARTESIAN_POINT('',(16.5,-15.1,40.)) ;
#100210=CARTESIAN_POINT('Origin',(10.5,-5.25000000000002,-40.001)) ;
#100211=CARTESIAN_POINT('',(10.5,-15.1,39.85)) ;
#100212=CARTESIAN_POINT('',(10.5,-5.40000000000002,39.85)) ;
#100213=CARTESIAN_POINT('',(10.5,-5.25000000000002,39.85)) ;
#100214=CARTESIAN_POINT('',(10.5,-5.40000000000002,39.4)) ;
#100215=CARTESIAN_POINT('',(10.5,-5.40000000000002,39.25)) ;
#100216=CARTESIAN_POINT('',(10.5,-15.1,39.4)) ;
#100217=CARTESIAN_POINT('',(10.5,-5.25000000000002,39.4)) ;
#100218=CARTESIAN_POINT('',(10.5,-15.1,40.)) ;
#100219=CARTESIAN_POINT('Origin',(7.49999999999997,-15.25,-40.001)) ;
#100220=CARTESIAN_POINT('',(7.64999999999997,-15.25,39.85)) ;
#100221=CARTESIAN_POINT('',(10.35,-15.25,39.85)) ;
#100222=CARTESIAN_POINT('',(10.5,-15.25,39.85)) ;
#100223=CARTESIAN_POINT('',(10.35,-15.25,39.4)) ;
#100224=CARTESIAN_POINT('',(10.35,-15.25,39.25)) ;
#100225=CARTESIAN_POINT('',(7.64999999999997,-15.25,39.4)) ;
#100226=CARTESIAN_POINT('',(7.49999999999997,-15.25,39.4)) ;
#100227=CARTESIAN_POINT('',(7.64999999999997,-15.25,40.)) ;
#100228=CARTESIAN_POINT('Origin',(7.49999999999996,-5.25000000000002,-40.001)) ;
#100229=CARTESIAN_POINT('',(7.49999999999996,-5.40000000000002,39.85)) ;
#100230=CARTESIAN_POINT('',(7.49999999999997,-15.1,39.85)) ;
#100231=CARTESIAN_POINT('',(7.49999999999997,-15.25,39.85)) ;
#100232=CARTESIAN_POINT('',(7.49999999999997,-15.1,39.4)) ;
#100233=CARTESIAN_POINT('',(7.49999999999997,-15.1,39.25)) ;
#100234=CARTESIAN_POINT('',(7.49999999999996,-5.40000000000002,39.4)) ;
#100235=CARTESIAN_POINT('',(7.49999999999996,-5.25000000000002,39.4)) ;
#100236=CARTESIAN_POINT('',(7.49999999999996,-5.40000000000002,40.)) ;
#100237=CARTESIAN_POINT('Origin',(7.49999999999996,-5.25000000000002,-40.001)) ;
#100238=CARTESIAN_POINT('',(7.64999999999996,-5.25000000000002,39.4)) ;
#100239=CARTESIAN_POINT('',(10.35,-5.25000000000002,39.4)) ;
#100240=CARTESIAN_POINT('',(7.49999999999996,-5.25000000000002,39.4)) ;
#100241=CARTESIAN_POINT('',(10.35,-5.25000000000002,39.85)) ;
#100242=CARTESIAN_POINT('',(10.35,-5.25000000000002,40.)) ;
#100243=CARTESIAN_POINT('',(7.64999999999996,-5.25000000000002,39.85)) ;
#100244=CARTESIAN_POINT('',(7.49999999999996,-5.25000000000002,39.85)) ;
#100245=CARTESIAN_POINT('',(7.64999999999996,-5.25000000000002,39.25)) ;
#100246=CARTESIAN_POINT('Origin',(46.5,-15.2500000000003,40.001)) ;
#100247=CARTESIAN_POINT('',(43.65,-15.2500000000003,-39.4)) ;
#100248=CARTESIAN_POINT('',(46.35,-15.2500000000003,-39.4)) ;
#100249=CARTESIAN_POINT('',(46.5,-15.2500000000003,-39.4)) ;
#100250=CARTESIAN_POINT('',(46.35,-15.2500000000003,-39.85)) ;
#100251=CARTESIAN_POINT('',(46.35,-15.2500000000003,-40.)) ;
#100252=CARTESIAN_POINT('',(43.65,-15.2500000000003,-39.85)) ;
#100253=CARTESIAN_POINT('',(43.5,-15.2500000000003,-39.85)) ;
#100254=CARTESIAN_POINT('',(43.65,-15.2500000000003,-39.25)) ;
#100255=CARTESIAN_POINT('Origin',(46.5,-5.25000000000033,40.001)) ;
#100256=CARTESIAN_POINT('',(46.5,-5.40000000000027,-39.85)) ;
#100257=CARTESIAN_POINT('',(46.5,-15.1000000000003,-39.85)) ;
#100258=CARTESIAN_POINT('',(46.5,-15.2500000000003,-39.85)) ;
#100259=CARTESIAN_POINT('',(46.5,-15.1000000000003,-39.4)) ;
#100260=CARTESIAN_POINT('',(46.5,-15.1000000000003,-39.25)) ;
#100261=CARTESIAN_POINT('',(46.5,-5.40000000000027,-39.4)) ;
#100262=CARTESIAN_POINT('',(46.5,-5.25000000000027,-39.4)) ;
#100263=CARTESIAN_POINT('',(46.5,-5.40000000000027,-40.)) ;
#100264=CARTESIAN_POINT('Origin',(46.5,-5.25000000000033,40.001)) ;
#100265=CARTESIAN_POINT('',(43.65,-5.25000000000027,-39.85)) ;
#100266=CARTESIAN_POINT('',(46.35,-5.25000000000027,-39.85)) ;
#100267=CARTESIAN_POINT('',(46.5,-5.25000000000027,-39.85)) ;
#100268=CARTESIAN_POINT('',(46.35,-5.25000000000027,-39.4)) ;
#100269=CARTESIAN_POINT('',(46.35,-5.25000000000027,-39.25)) ;
#100270=CARTESIAN_POINT('',(43.65,-5.25000000000027,-39.4)) ;
#100271=CARTESIAN_POINT('',(46.5,-5.25000000000027,-39.4)) ;
#100272=CARTESIAN_POINT('',(43.65,-5.25000000000027,-40.)) ;
#100273=CARTESIAN_POINT('Origin',(43.5,-5.25000000000033,40.001)) ;
#100274=CARTESIAN_POINT('',(43.5,-15.1000000000003,-39.85)) ;
#100275=CARTESIAN_POINT('',(43.5,-5.40000000000027,-39.85)) ;
#100276=CARTESIAN_POINT('',(43.5,-5.25000000000027,-39.85)) ;
#100277=CARTESIAN_POINT('',(43.5,-5.40000000000027,-39.4)) ;
#100278=CARTESIAN_POINT('',(43.5,-5.40000000000027,-39.25)) ;
#100279=CARTESIAN_POINT('',(43.5,-15.1000000000003,-39.4)) ;
#100280=CARTESIAN_POINT('',(43.5,-5.25000000000027,-39.4)) ;
#100281=CARTESIAN_POINT('',(43.5,-15.1000000000003,-40.)) ;
#100282=CARTESIAN_POINT('Origin',(38.25,-2.75000000000007,40.001)) ;
#100283=CARTESIAN_POINT('',(38.1,-2.75000000000002,-39.4)) ;
#100284=CARTESIAN_POINT('',(19.4,-2.75000000000002,-39.4)) ;
#100285=CARTESIAN_POINT('',(38.25,-2.75000000000002,-39.4)) ;
#100286=CARTESIAN_POINT('',(19.4,-2.75000000000002,-39.85)) ;
#100287=CARTESIAN_POINT('',(19.4,-2.75000000000002,-40.)) ;
#100288=CARTESIAN_POINT('',(38.1,-2.75000000000002,-39.85)) ;
#100289=CARTESIAN_POINT('',(38.25,-2.75000000000002,-39.85)) ;
#100290=CARTESIAN_POINT('',(38.1,-2.75000000000002,-39.25)) ;
#100291=CARTESIAN_POINT('Origin',(38.25,-2.75000000000007,40.001)) ;
#100292=CARTESIAN_POINT('',(38.25,-2.90000000000002,-39.85)) ;
#100293=CARTESIAN_POINT('',(38.25,-13.1,-39.85)) ;
#100294=CARTESIAN_POINT('',(38.25,-13.25,-39.85)) ;
#100295=CARTESIAN_POINT('',(38.25,-13.1,-39.4)) ;
#100296=CARTESIAN_POINT('',(38.25,-13.1,-39.25)) ;
#100297=CARTESIAN_POINT('',(38.25,-2.90000000000002,-39.4)) ;
#100298=CARTESIAN_POINT('',(38.25,-2.75000000000002,-39.4)) ;
#100299=CARTESIAN_POINT('',(38.25,-2.90000000000002,-40.)) ;
#100300=CARTESIAN_POINT('Origin',(38.25,-13.2500000000001,40.001)) ;
#100301=CARTESIAN_POINT('',(38.1,-13.25,-39.85)) ;
#100302=CARTESIAN_POINT('',(19.4,-13.25,-39.85)) ;
#100303=CARTESIAN_POINT('',(19.25,-13.25,-39.85)) ;
#100304=CARTESIAN_POINT('',(19.4,-13.25,-39.4)) ;
#100305=CARTESIAN_POINT('',(19.4,-13.25,-39.25)) ;
#100306=CARTESIAN_POINT('',(38.1,-13.25,-39.4)) ;
#100307=CARTESIAN_POINT('',(38.25,-13.25,-39.4)) ;
#100308=CARTESIAN_POINT('',(38.1,-13.25,-40.)) ;
#100309=CARTESIAN_POINT('Origin',(19.25,-2.75000000000007,40.001)) ;
#100310=CARTESIAN_POINT('',(19.25,-13.1,-39.85)) ;
#100311=CARTESIAN_POINT('',(19.25,-2.90000000000002,-39.85)) ;
#100312=CARTESIAN_POINT('',(19.25,-2.75000000000002,-39.85)) ;
#100313=CARTESIAN_POINT('',(19.25,-2.90000000000002,-39.4)) ;
#100314=CARTESIAN_POINT('',(19.25,-2.90000000000002,-39.25)) ;
#100315=CARTESIAN_POINT('',(19.25,-13.1,-39.4)) ;
#100316=CARTESIAN_POINT('',(19.25,-2.75000000000002,-39.4)) ;
#100317=CARTESIAN_POINT('',(19.25,-13.1,-40.)) ;
#100318=CARTESIAN_POINT('Origin',(16.5,-15.2500000000001,40.001)) ;
#100319=CARTESIAN_POINT('',(13.65,-15.2500000000001,-39.4)) ;
#100320=CARTESIAN_POINT('',(16.35,-15.2500000000001,-39.4)) ;
#100321=CARTESIAN_POINT('',(16.5,-15.2500000000001,-39.4)) ;
#100322=CARTESIAN_POINT('',(16.35,-15.2500000000001,-39.85)) ;
#100323=CARTESIAN_POINT('',(16.35,-15.2500000000001,-40.)) ;
#100324=CARTESIAN_POINT('',(13.65,-15.2500000000001,-39.85)) ;
#100325=CARTESIAN_POINT('',(13.5,-15.2500000000001,-39.85)) ;
#100326=CARTESIAN_POINT('',(13.65,-15.2500000000001,-39.25)) ;
#100327=CARTESIAN_POINT('Origin',(16.5,-5.25000000000011,40.001)) ;
#100328=CARTESIAN_POINT('',(16.5,-5.40000000000006,-39.85)) ;
#100329=CARTESIAN_POINT('',(16.5,-15.1000000000001,-39.85)) ;
#100330=CARTESIAN_POINT('',(16.5,-15.2500000000001,-39.85)) ;
#100331=CARTESIAN_POINT('',(16.5,-15.1000000000001,-39.4)) ;
#100332=CARTESIAN_POINT('',(16.5,-15.1000000000001,-39.25)) ;
#100333=CARTESIAN_POINT('',(16.5,-5.40000000000006,-39.4)) ;
#100334=CARTESIAN_POINT('',(16.5,-5.25000000000006,-39.4)) ;
#100335=CARTESIAN_POINT('',(16.5,-5.40000000000006,-40.)) ;
#100336=CARTESIAN_POINT('Origin',(16.5,-5.25000000000011,40.001)) ;
#100337=CARTESIAN_POINT('',(13.65,-5.25000000000006,-39.85)) ;
#100338=CARTESIAN_POINT('',(16.35,-5.25000000000006,-39.85)) ;
#100339=CARTESIAN_POINT('',(16.5,-5.25000000000006,-39.85)) ;
#100340=CARTESIAN_POINT('',(16.35,-5.25000000000006,-39.4)) ;
#100341=CARTESIAN_POINT('',(16.35,-5.25000000000006,-39.25)) ;
#100342=CARTESIAN_POINT('',(13.65,-5.25000000000006,-39.4)) ;
#100343=CARTESIAN_POINT('',(16.5,-5.25000000000006,-39.4)) ;
#100344=CARTESIAN_POINT('',(13.65,-5.25000000000006,-40.)) ;
#100345=CARTESIAN_POINT('Origin',(13.5,-5.25000000000011,40.001)) ;
#100346=CARTESIAN_POINT('',(13.5,-15.1000000000001,-39.85)) ;
#100347=CARTESIAN_POINT('',(13.5,-5.40000000000006,-39.85)) ;
#100348=CARTESIAN_POINT('',(13.5,-5.25000000000006,-39.85)) ;
#100349=CARTESIAN_POINT('',(13.5,-5.40000000000006,-39.4)) ;
#100350=CARTESIAN_POINT('',(13.5,-5.40000000000006,-39.25)) ;
#100351=CARTESIAN_POINT('',(13.5,-15.1000000000001,-39.4)) ;
#100352=CARTESIAN_POINT('',(13.5,-5.25000000000006,-39.4)) ;
#100353=CARTESIAN_POINT('',(13.5,-15.1000000000001,-40.)) ;
#100354=CARTESIAN_POINT('Origin',(7.49999999999997,-5.25000000000007,40.001)) ;
#100355=CARTESIAN_POINT('',(7.49999999999996,-15.1,-39.85)) ;
#100356=CARTESIAN_POINT('',(7.49999999999997,-5.40000000000002,-39.85)) ;
#100357=CARTESIAN_POINT('',(7.49999999999997,-5.25000000000002,-39.85)) ;
#100358=CARTESIAN_POINT('',(7.49999999999997,-5.40000000000002,-39.4)) ;
#100359=CARTESIAN_POINT('',(7.49999999999997,-5.40000000000002,-39.25)) ;
#100360=CARTESIAN_POINT('',(7.49999999999996,-15.1,-39.4)) ;
#100361=CARTESIAN_POINT('',(7.49999999999997,-5.25000000000002,-39.4)) ;
#100362=CARTESIAN_POINT('',(7.49999999999996,-15.1,-40.)) ;
#100363=CARTESIAN_POINT('Origin',(10.5,-15.2500000000001,40.001)) ;
#100364=CARTESIAN_POINT('',(10.35,-15.25,-39.85)) ;
#100365=CARTESIAN_POINT('',(7.64999999999996,-15.25,-39.85)) ;
#100366=CARTESIAN_POINT('',(7.49999999999996,-15.25,-39.85)) ;
#100367=CARTESIAN_POINT('',(7.64999999999996,-15.25,-39.4)) ;
#100368=CARTESIAN_POINT('',(7.64999999999996,-15.25,-39.25)) ;
#100369=CARTESIAN_POINT('',(10.35,-15.25,-39.4)) ;
#100370=CARTESIAN_POINT('',(10.5,-15.25,-39.4)) ;
#100371=CARTESIAN_POINT('',(10.35,-15.25,-40.)) ;
#100372=CARTESIAN_POINT('Origin',(10.5,-5.25000000000007,40.001)) ;
#100373=CARTESIAN_POINT('',(10.5,-5.40000000000002,-39.85)) ;
#100374=CARTESIAN_POINT('',(10.5,-15.1,-39.85)) ;
#100375=CARTESIAN_POINT('',(10.5,-15.25,-39.85)) ;
#100376=CARTESIAN_POINT('',(10.5,-15.1,-39.4)) ;
#100377=CARTESIAN_POINT('',(10.5,-15.1,-39.25)) ;
#100378=CARTESIAN_POINT('',(10.5,-5.40000000000002,-39.4)) ;
#100379=CARTESIAN_POINT('',(10.5,-5.25000000000002,-39.4)) ;
#100380=CARTESIAN_POINT('',(10.5,-5.40000000000002,-40.)) ;
#100381=CARTESIAN_POINT('Origin',(10.5,-5.25000000000007,40.001)) ;
#100382=CARTESIAN_POINT('',(10.35,-5.25000000000002,-39.4)) ;
#100383=CARTESIAN_POINT('',(7.64999999999997,-5.25000000000002,-39.4)) ;
#100384=CARTESIAN_POINT('',(10.5,-5.25000000000002,-39.4)) ;
#100385=CARTESIAN_POINT('',(7.64999999999997,-5.25000000000002,-39.85)) ;
#100386=CARTESIAN_POINT('',(7.64999999999997,-5.25000000000002,-40.)) ;
#100387=CARTESIAN_POINT('',(10.35,-5.25000000000002,-39.85)) ;
#100388=CARTESIAN_POINT('',(10.5,-5.25000000000002,-39.85)) ;
#100389=CARTESIAN_POINT('',(10.35,-5.25000000000002,-39.25)) ;
#100390=CARTESIAN_POINT('Origin',(-2.00100000000011,-4.2500000000002,-32.5)) ;
#100391=CARTESIAN_POINT('',(53.85,-4.39999999999999,-32.5)) ;
#100392=CARTESIAN_POINT('',(53.4,-4.4,-32.5)) ;
#100393=CARTESIAN_POINT('',(53.25,-4.4,-32.5)) ;
#100394=CARTESIAN_POINT('',(53.4,-14.1,-32.5)) ;
#100395=CARTESIAN_POINT('',(53.4,-14.25,-32.5)) ;
#100396=CARTESIAN_POINT('',(53.8500000000001,-14.1,-32.5)) ;
#100397=CARTESIAN_POINT('',(54.0000000000001,-14.1,-32.5)) ;
#100398=CARTESIAN_POINT('',(53.85,-4.24999999999999,-32.5)) ;
#100399=CARTESIAN_POINT('Origin',(-2.00100000000007,-14.2500000000002,34.)) ;
#100400=CARTESIAN_POINT('',(53.8500000000001,-14.25,33.85)) ;
#100401=CARTESIAN_POINT('',(53.8500000000001,-14.25,-32.35)) ;
#100402=CARTESIAN_POINT('',(53.8500000000001,-14.25,34.)) ;
#100403=CARTESIAN_POINT('',(53.4,-14.25,-32.35)) ;
#100404=CARTESIAN_POINT('',(53.2500000000001,-14.25,-32.35)) ;
#100405=CARTESIAN_POINT('',(53.4,-14.25,33.85)) ;
#100406=CARTESIAN_POINT('',(53.4,-14.25,34.)) ;
#100407=CARTESIAN_POINT('',(54.0000000000001,-14.25,33.85)) ;
#100408=CARTESIAN_POINT('Origin',(-2.00100000000011,-4.2500000000002,34.)) ;
#100409=CARTESIAN_POINT('',(53.8500000000001,-14.1,34.)) ;
#100410=CARTESIAN_POINT('',(53.4,-14.1,34.)) ;
#100411=CARTESIAN_POINT('',(53.2500000000001,-14.1,34.)) ;
#100412=CARTESIAN_POINT('',(53.4,-4.4,34.)) ;
#100413=CARTESIAN_POINT('',(53.4,-4.25,34.)) ;
#100414=CARTESIAN_POINT('',(53.85,-4.4,34.)) ;
#100415=CARTESIAN_POINT('',(54.,-4.39999999999999,34.)) ;
#100416=CARTESIAN_POINT('',(53.85,-4.24999999999999,34.)) ;
#100417=CARTESIAN_POINT('Origin',(-2.00100000000011,-4.2500000000002,34.)) ;
#100418=CARTESIAN_POINT('',(53.4,-4.25,33.85)) ;
#100419=CARTESIAN_POINT('',(53.4,-4.25,-32.35)) ;
#100420=CARTESIAN_POINT('',(53.4,-4.25,-32.5)) ;
#100421=CARTESIAN_POINT('',(53.85,-4.24999999999999,-32.35)) ;
#100422=CARTESIAN_POINT('',(54.,-4.24999999999999,-32.35)) ;
#100423=CARTESIAN_POINT('',(53.85,-4.24999999999999,33.85)) ;
#100424=CARTESIAN_POINT('',(53.85,-4.24999999999999,34.)) ;
#100425=CARTESIAN_POINT('',(53.25,-4.25,33.85)) ;
#100426=CARTESIAN_POINT('Origin',(53.,-7.91804761436593E-15,-39.85)) ;
#100427=CARTESIAN_POINT('Origin',(53.0000000000001,-19.6,-39.85)) ;
#100428=CARTESIAN_POINT('Origin',(53.0000000000001,-1.89999999999994,-39.8500000000001)) ;
#100429=CARTESIAN_POINT('Origin',(53.,-1.89999999999999,-39.25)) ;
#100430=CARTESIAN_POINT('Origin',(52.9999999999994,-1.90000000000071,-39.4000000000007)) ;
#100431=CARTESIAN_POINT('Origin',(53.0000000000001,-19.6,-39.85)) ;
#100432=CARTESIAN_POINT('Origin',(53.0000000000001,-19.6,-39.85)) ;
#100433=CARTESIAN_POINT('Origin',(53.0000000000001,-19.6,-39.85)) ;
#100434=CARTESIAN_POINT('Origin',(52.9999999999998,56.3581964958473,-39.4)) ;
#100435=CARTESIAN_POINT('Origin',(53.0000000000001,-19.6,-39.4)) ;
#100436=CARTESIAN_POINT('Origin',(53.0000000000001,-19.6,-40.)) ;
#100437=CARTESIAN_POINT('Origin',(53.0000000000001,-19.6,-39.4)) ;
#100438=CARTESIAN_POINT('Origin',(53.25,-19.6,-39.85)) ;
#100439=CARTESIAN_POINT('Origin',(0.149999999999965,-19.6,-39.85)) ;
#100440=CARTESIAN_POINT('Origin',(53.0000000000001,-19.6,-39.4)) ;
#100441=CARTESIAN_POINT('Origin',(53.0000000000001,-19.6,-39.4)) ;
#100442=CARTESIAN_POINT('Origin',(0.149999999999965,-19.6,-39.85)) ;
#100443=CARTESIAN_POINT('Origin',(0.149999999999965,-19.6,-39.85)) ;
#100444=CARTESIAN_POINT('Origin',(0.149999999999965,-19.6,-39.85)) ;
#100445=CARTESIAN_POINT('Origin',(53.25,-19.6,-39.4)) ;
#100446=CARTESIAN_POINT('Origin',(0.149999999999965,-19.6,-39.4)) ;
#100447=CARTESIAN_POINT('Origin',(0.149999999999965,-19.6,-38.25)) ;
#100448=CARTESIAN_POINT('Origin',(0.149999999999965,-19.6,-39.4)) ;
#100449=CARTESIAN_POINT('Origin',(0.149999999999965,-1.74999999999999,-39.85)) ;
#100450=CARTESIAN_POINT('Origin',(0.149999999999965,-6.90000000000001,-39.85)) ;
#100451=CARTESIAN_POINT('Origin',(0.149999999999965,-19.6,-39.4)) ;
#100452=CARTESIAN_POINT('Origin',(0.149999999999963,-19.6,-39.4)) ;
#100453=CARTESIAN_POINT('Origin',(-0.150000000000035,-6.90000000000001,
-39.85)) ;
#100454=CARTESIAN_POINT('Origin',(-0.150000000000035,-6.90000000000001,
-39.85)) ;
#100455=CARTESIAN_POINT('Origin',(-0.150000000000035,-6.60000000000001,
-39.85)) ;
#100456=CARTESIAN_POINT('Origin',(0.149999999999963,-6.83349298384788E-15,
-39.4)) ;
#100457=CARTESIAN_POINT('Origin',(0.149999999999965,-6.90000000000001,-39.4)) ;
#100458=CARTESIAN_POINT('Origin',(-0.150000000000035,-6.90000000000001,
-38.25)) ;
#100459=CARTESIAN_POINT('Origin',(-0.150000000000035,-6.90000000000001,
-39.4)) ;
#100460=CARTESIAN_POINT('Origin',(-3.46944695195361E-14,-6.60000000000001,
-39.85)) ;
#100461=CARTESIAN_POINT('Origin',(-1.85000000000003,-6.60000000000001,-39.85)) ;
#100462=CARTESIAN_POINT('Origin',(-0.150000000000035,-6.90000000000001,
-39.4)) ;
#100463=CARTESIAN_POINT('Origin',(-0.150000000000035,-6.60000000000001,
-39.4)) ;
#100464=CARTESIAN_POINT('Origin',(-1.85000000000003,-6.60000000000001,-39.85)) ;
#100465=CARTESIAN_POINT('Origin',(-1.85000000000003,-6.60000000000001,-39.85)) ;
#100466=CARTESIAN_POINT('Origin',(-1.85000000000003,-6.60000000000001,-39.85)) ;
#100467=CARTESIAN_POINT('Origin',(53.25,-6.60000000000001,-39.4)) ;
#100468=CARTESIAN_POINT('Origin',(-1.85000000000003,-6.60000000000001,-39.4)) ;
#100469=CARTESIAN_POINT('Origin',(-1.85000000000003,-6.60000000000001,-39.25)) ;
#100470=CARTESIAN_POINT('Origin',(-1.85000000000003,-6.60000000000001,-39.4)) ;
#100471=CARTESIAN_POINT('Origin',(-1.85000000000003,-4.75000000000001,-39.85)) ;
#100472=CARTESIAN_POINT('Origin',(-1.85000000000003,-4.9,-39.85)) ;
#100473=CARTESIAN_POINT('Origin',(-1.85000000000003,-6.60000000000001,-39.4)) ;
#100474=CARTESIAN_POINT('Origin',(-1.85000000000003,-6.60000000000001,-39.4)) ;
#100475=CARTESIAN_POINT('Origin',(-1.85000000000003,-4.9,-39.85)) ;
#100476=CARTESIAN_POINT('Origin',(-1.85000000000003,-4.9,-39.85)) ;
#100477=CARTESIAN_POINT('Origin',(-1.85000000000003,-4.9,-39.85)) ;
#100478=CARTESIAN_POINT('Origin',(-1.85000000000003,-1.87814009246381E-14,
-39.4)) ;
#100479=CARTESIAN_POINT('Origin',(-1.85000000000003,-4.9,-39.4)) ;
#100480=CARTESIAN_POINT('Origin',(-1.85000000000003,-4.9,-39.25)) ;
#100481=CARTESIAN_POINT('Origin',(-1.85000000000003,-4.9,-39.4)) ;
#100482=CARTESIAN_POINT('Origin',(-2.77555756156289E-14,-4.9,-39.85)) ;
#100483=CARTESIAN_POINT('Origin',(-0.150000000000035,-4.9,-39.85)) ;
#100484=CARTESIAN_POINT('Origin',(52.9999999999998,56.3581964958473,39.85)) ;
#100485=CARTESIAN_POINT('Origin',(52.9999999999998,-1.90000000000013,39.8499999999999)) ;
#100486=CARTESIAN_POINT('Origin',(53.,-19.6,39.85)) ;
#100487=CARTESIAN_POINT('Origin',(-1.85000000000003,-4.9,-39.4)) ;
#100488=CARTESIAN_POINT('Origin',(-1.85000000000003,-4.9,-39.4)) ;
#100489=CARTESIAN_POINT('Origin',(-0.150000000000035,-4.6,-39.85)) ;
#100490=CARTESIAN_POINT('Origin',(-0.150000000000035,-4.6,-39.85)) ;
#100491=CARTESIAN_POINT('Origin',(0.149999999999965,-4.6,-39.85)) ;
#100492=CARTESIAN_POINT('Origin',(53.,-19.6,39.85)) ;
#100493=CARTESIAN_POINT('Origin',(53.,-19.6,39.85)) ;
#100494=CARTESIAN_POINT('Origin',(53.,-19.6,39.85)) ;
#100495=CARTESIAN_POINT('Origin',(53.,-1.90000000000001,39.25)) ;
#100496=CARTESIAN_POINT('Origin',(52.9999999999997,-1.90000000000036,39.4000000000004)) ;
#100497=CARTESIAN_POINT('Origin',(53.25,-4.9,-39.4)) ;
#100498=CARTESIAN_POINT('Origin',(-0.150000000000035,-4.9,-39.4)) ;
#100499=CARTESIAN_POINT('Origin',(-0.150000000000035,-4.6,-39.25)) ;
#100500=CARTESIAN_POINT('Origin',(-0.150000000000035,-4.6,-39.4)) ;
#100501=CARTESIAN_POINT('Origin',(0.149999999999965,-1.74999999999999,-39.85)) ;
#100502=CARTESIAN_POINT('Origin',(0.149999999999965,-1.75,-39.85)) ;
#100503=CARTESIAN_POINT('Origin',(53.25,-19.6,39.85)) ;
#100504=CARTESIAN_POINT('Origin',(0.149999999999972,-19.6,39.85)) ;
#100505=CARTESIAN_POINT('Origin',(53.,-19.6,39.25)) ;
#100506=CARTESIAN_POINT('Origin',(53.,-19.6,39.4)) ;
#100507=CARTESIAN_POINT('Origin',(53.,-19.75,39.4)) ;
#100508=CARTESIAN_POINT('Origin',(53.,-19.6,39.4)) ;
#100509=CARTESIAN_POINT('Origin',(-0.150000000000035,-4.6,-39.4)) ;
#100510=CARTESIAN_POINT('Origin',(0.149999999999963,-4.6,-39.4)) ;
#100511=CARTESIAN_POINT('Origin',(0.14999999999997,-1.75000000000001,-38.25)) ;
#100512=CARTESIAN_POINT('Origin',(0.15000000000005,-0.150000000000014,-38.25)) ;
#100513=CARTESIAN_POINT('Origin',(0.149999999999972,-19.6,39.85)) ;
#100514=CARTESIAN_POINT('Origin',(0.149999999999972,-19.6,39.85)) ;
#100515=CARTESIAN_POINT('Origin',(0.149999999999972,-19.6,39.85)) ;
#100516=CARTESIAN_POINT('Origin',(53.,-19.6,39.4)) ;
#100517=CARTESIAN_POINT('Origin',(53.,-19.6,39.4)) ;
#100518=CARTESIAN_POINT('Origin',(0.149999999999963,-6.83349298384788E-15,
-39.4)) ;
#100519=CARTESIAN_POINT('Origin',(0.149999999999965,-1.74999999999999,-39.4)) ;
#100520=CARTESIAN_POINT('Origin',(0.149999999999965,-0.150000000000013,
-39.25)) ;
#100521=CARTESIAN_POINT('Origin',(0.149999999999965,-0.150000000000018,
-14.15)) ;
#100522=CARTESIAN_POINT('Origin',(0.149999999999972,-0.750000000000015,
39.85)) ;
#100523=CARTESIAN_POINT('Origin',(0.149999999999972,-6.90000000000001,39.85)) ;
#100524=CARTESIAN_POINT('Origin',(0.149999999999972,-19.6,38.25)) ;
#100525=CARTESIAN_POINT('Origin',(0.149999999999972,-19.6,39.4)) ;
#100526=CARTESIAN_POINT('Origin',(53.25,-19.6,39.4)) ;
#100527=CARTESIAN_POINT('Origin',(0.14999999999997,-19.6,39.4)) ;
#100528=CARTESIAN_POINT('Origin',(0.14999999999997,-1.75000000000001,-38.25)) ;
#100529=CARTESIAN_POINT('Origin',(0.150000000000031,-0.600000000000014,
-38.25)) ;
#100530=CARTESIAN_POINT('Origin',(-0.150000000000035,-0.150000000000018,
-14.15)) ;
#100531=CARTESIAN_POINT('Origin',(-0.150000000000035,-0.150000000000018,
-14.15)) ;
#100532=CARTESIAN_POINT('Origin',(-0.150000000000035,-0.150000000000018,
-13.85)) ;
#100533=CARTESIAN_POINT('Origin',(-0.150000000000028,-6.90000000000001,
39.85)) ;
#100534=CARTESIAN_POINT('Origin',(-0.150000000000028,-6.60000000000001,
39.85)) ;
#100535=CARTESIAN_POINT('Origin',(-0.150000000000028,-6.90000000000001,
39.85)) ;
#100536=CARTESIAN_POINT('Origin',(0.149999999999972,-19.6,39.4)) ;
#100537=CARTESIAN_POINT('Origin',(0.149999999999972,-19.6,39.4)) ;
#100538=CARTESIAN_POINT('Origin',(0.149999999999963,-0.600000000000029,
40.)) ;
#100539=CARTESIAN_POINT('Origin',(0.149999999999965,-0.600000000000019,
-14.15)) ;
#100540=CARTESIAN_POINT('Origin',(-0.150000000000035,-1.75000000000001,
-14.15)) ;
#100541=CARTESIAN_POINT('Origin',(-0.150000000000035,-0.600000000000019,
-14.15)) ;
#100542=CARTESIAN_POINT('Origin',(53.25,-0.150000000000018,-13.85)) ;
#100543=CARTESIAN_POINT('Origin',(-1.85000000000004,-0.150000000000018,
-13.85)) ;
#100544=CARTESIAN_POINT('Origin',(53.25,-6.60000000000001,39.85)) ;
#100545=CARTESIAN_POINT('Origin',(-1.85000000000003,-6.60000000000001,39.85)) ;
#100546=CARTESIAN_POINT('Origin',(-0.150000000000028,-6.90000000000001,
39.25)) ;
#100547=CARTESIAN_POINT('Origin',(-0.150000000000028,-6.90000000000001,
39.4)) ;
#100548=CARTESIAN_POINT('Origin',(0.14999999999997,-19.75,39.4)) ;
#100549=CARTESIAN_POINT('Origin',(0.14999999999997,-6.90000000000001,39.4)) ;
#100550=CARTESIAN_POINT('Origin',(-0.150000000000035,-0.600000000000019,
-14.15)) ;
#100551=CARTESIAN_POINT('Origin',(-0.150000000000035,-0.600000000000019,
-13.85)) ;
#100552=CARTESIAN_POINT('Origin',(-1.85000000000004,-0.150000000000018,
-13.85)) ;
#100553=CARTESIAN_POINT('Origin',(-1.85000000000004,-0.150000000000018,
-13.85)) ;
#100554=CARTESIAN_POINT('Origin',(-1.85000000000004,-0.150000000000018,
-13.85)) ;
#100555=CARTESIAN_POINT('Origin',(-1.85000000000003,-6.60000000000001,39.85)) ;
#100556=CARTESIAN_POINT('Origin',(-1.85000000000003,-6.60000000000001,39.85)) ;
#100557=CARTESIAN_POINT('Origin',(-1.85000000000003,-6.60000000000001,39.85)) ;
#100558=CARTESIAN_POINT('Origin',(-0.150000000000028,-6.90000000000001,
39.4)) ;
#100559=CARTESIAN_POINT('Origin',(-0.150000000000028,-6.60000000000001,
39.4)) ;
#100560=CARTESIAN_POINT('Origin',(-4.85722573273506E-14,-0.600000000000019,
-13.85)) ;
#100561=CARTESIAN_POINT('Origin',(-1.85000000000004,-0.600000000000019,
-13.85)) ;
#100562=CARTESIAN_POINT('Origin',(-1.85000000000004,-0.750000000000015,
-13.85)) ;
#100563=CARTESIAN_POINT('Origin',(-1.85000000000004,-0.600000000000019,
-13.85)) ;
#100564=CARTESIAN_POINT('Origin',(-1.85000000000004,-0.150000000000028,
40.)) ;
#100565=CARTESIAN_POINT('Origin',(-1.85000000000004,-0.150000000000023,
13.85)) ;
#100566=CARTESIAN_POINT('Origin',(-1.85000000000003,-19.75,39.85)) ;
#100567=CARTESIAN_POINT('Origin',(-1.85000000000003,-4.90000000000001,39.85)) ;
#100568=CARTESIAN_POINT('Origin',(-1.85000000000003,-6.60000000000001,39.25)) ;
#100569=CARTESIAN_POINT('Origin',(-1.85000000000003,-6.60000000000001,39.4)) ;
#100570=CARTESIAN_POINT('Origin',(-2.77555756156289E-14,-6.60000000000001,
39.4)) ;
#100571=CARTESIAN_POINT('Origin',(-1.85000000000003,-6.60000000000001,39.4)) ;
#100572=CARTESIAN_POINT('Origin',(-1.85000000000004,-0.600000000000019,
-13.85)) ;
#100573=CARTESIAN_POINT('Origin',(-1.85000000000004,-0.600000000000019,
-13.85)) ;
#100574=CARTESIAN_POINT('Origin',(-1.85000000000004,-0.150000000000023,
13.85)) ;
#100575=CARTESIAN_POINT('Origin',(-1.85000000000004,-0.150000000000023,
13.85)) ;
#100576=CARTESIAN_POINT('Origin',(-1.85000000000004,-0.150000000000023,
13.85)) ;
#100577=CARTESIAN_POINT('Origin',(0.149999999999966,-1.75000000000003,38.25)) ;
#100578=CARTESIAN_POINT('Origin',(0.149999999999966,-1.75000000000002,39.85)) ;
#100579=CARTESIAN_POINT('Origin',(0.149999999999965,-0.150000000000029,
38.25)) ;
#100580=CARTESIAN_POINT('Origin',(-1.85000000000003,-4.90000000000001,39.85)) ;
#100581=CARTESIAN_POINT('Origin',(-1.85000000000003,-4.90000000000001,39.85)) ;
#100582=CARTESIAN_POINT('Origin',(-1.85000000000004,-4.90000000000001,39.85)) ;
#100583=CARTESIAN_POINT('Origin',(-1.85000000000003,-6.60000000000001,39.4)) ;
#100584=CARTESIAN_POINT('Origin',(-1.85000000000003,-6.60000000000001,39.4)) ;
#100585=CARTESIAN_POINT('Origin',(-1.85000000000004,-0.600000000000024,
14.)) ;
#100586=CARTESIAN_POINT('Origin',(-1.85000000000004,-0.600000000000024,
13.85)) ;
#100587=CARTESIAN_POINT('Origin',(-1.85000000000004,-0.750000000000028,
13.85)) ;
#100588=CARTESIAN_POINT('Origin',(-1.85000000000004,-0.600000000000024,
13.85)) ;
#100589=CARTESIAN_POINT('Origin',(53.25,-0.150000000000023,13.85)) ;
#100590=CARTESIAN_POINT('Origin',(-0.150000000000035,-0.150000000000023,
13.85)) ;
#100591=CARTESIAN_POINT('Origin',(0.149999999999965,-0.150000000000013,
-39.25)) ;
#100592=CARTESIAN_POINT('Origin',(0.149999999999965,-0.150000000000023,
14.15)) ;
#100593=CARTESIAN_POINT('Origin',(0.149999999999972,-0.750000000000015,
39.85)) ;
#100594=CARTESIAN_POINT('Origin',(0.149999999999972,-4.60000000000001,39.85)) ;
#100595=CARTESIAN_POINT('Origin',(53.25,-4.90000000000001,39.85)) ;
#100596=CARTESIAN_POINT('Origin',(-0.150000000000028,-4.90000000000001,
39.85)) ;
#100597=CARTESIAN_POINT('Origin',(-1.85000000000003,-4.90000000000001,39.25)) ;
#100598=CARTESIAN_POINT('Origin',(-1.85000000000003,-4.90000000000001,39.4)) ;
#100599=CARTESIAN_POINT('Origin',(-1.85000000000003,-4.75000000000002,39.4)) ;
#100600=CARTESIAN_POINT('Origin',(-1.85000000000003,-4.90000000000001,39.4)) ;
#100601=CARTESIAN_POINT('Origin',(-1.85000000000004,-0.600000000000024,
13.85)) ;
#100602=CARTESIAN_POINT('Origin',(-1.85000000000004,-0.600000000000024,
13.85)) ;
#100603=CARTESIAN_POINT('Origin',(-0.150000000000035,-0.150000000000023,
14.15)) ;
#100604=CARTESIAN_POINT('Origin',(-0.150000000000035,-0.150000000000023,
14.15)) ;
#100605=CARTESIAN_POINT('Origin',(-0.150000000000028,-4.60000000000001,
39.85)) ;
#100606=CARTESIAN_POINT('Origin',(-0.150000000000028,-4.60000000000001,
39.85)) ;
#100607=CARTESIAN_POINT('Origin',(-1.85000000000003,-4.90000000000001,39.4)) ;
#100608=CARTESIAN_POINT('Origin',(-1.85000000000003,-4.90000000000001,39.4)) ;
#100609=CARTESIAN_POINT('Origin',(-3.46944695195361E-14,-0.600000000000024,
13.85)) ;
#100610=CARTESIAN_POINT('Origin',(-0.150000000000035,-0.600000000000024,
13.85)) ;
#100611=CARTESIAN_POINT('Origin',(-0.150000000000035,-0.750000000000015,
14.15)) ;
#100612=CARTESIAN_POINT('Origin',(-0.150000000000035,-0.600000000000024,
14.15)) ;
#100613=CARTESIAN_POINT('Origin',(-0.150000000000028,-4.60000000000001,
38.25)) ;
#100614=CARTESIAN_POINT('Origin',(-0.150000000000028,-4.60000000000001,
39.4)) ;
#100615=CARTESIAN_POINT('Origin',(-2.77555756156289E-14,-4.90000000000001,
39.4)) ;
#100616=CARTESIAN_POINT('Origin',(-0.150000000000028,-4.90000000000001,
39.4)) ;
#100617=CARTESIAN_POINT('Origin',(-0.150000000000035,-0.600000000000024,
14.15)) ;
#100618=CARTESIAN_POINT('Origin',(0.149999999999963,-0.600000000000024,
14.15)) ;
#100619=CARTESIAN_POINT('Origin',(-0.150000000000028,-4.60000000000001,
39.4)) ;
#100620=CARTESIAN_POINT('Origin',(0.149999999999972,-4.60000000000001,39.4)) ;
#100621=CARTESIAN_POINT('Origin',(0.149999999999963,-0.600000000000029,
40.)) ;
#100622=CARTESIAN_POINT('Origin',(0.149999999999965,-0.600000000000028,
38.25)) ;
#100623=CARTESIAN_POINT('Origin',(0.14999999999997,-19.75,39.4)) ;
#100624=CARTESIAN_POINT('Origin',(0.14999999999997,-1.75000000000002,39.4)) ;
#100625=CARTESIAN_POINT('Origin',(0.149999999999966,-1.75000000000003,38.25)) ;
#100626=CARTESIAN_POINT('Origin',(10.5,-5.10000000000002,-39.85)) ;
#100627=CARTESIAN_POINT('Origin',(7.64999999999997,-5.10000000000002,-39.85)) ;
#100628=CARTESIAN_POINT('Origin',(10.35,-5.10000000000002,-39.85)) ;
#100629=CARTESIAN_POINT('Origin',(7.64999999999997,-5.40000000000002,-39.85)) ;
#100630=CARTESIAN_POINT('Origin',(7.64999999999997,-5.40000000000002,-39.85)) ;
#100631=CARTESIAN_POINT('Origin',(7.34999999999997,-5.40000000000002,-39.85)) ;
#100632=CARTESIAN_POINT('Origin',(10.35,-5.40000000000002,-39.85)) ;
#100633=CARTESIAN_POINT('Origin',(10.65,-5.40000000000002,-39.85)) ;
#100634=CARTESIAN_POINT('Origin',(10.35,-5.40000000000002,-39.85)) ;
#100635=CARTESIAN_POINT('Origin',(7.64999999999997,-5.40000000000007,40.001)) ;
#100636=CARTESIAN_POINT('Origin',(7.64999999999997,-5.40000000000002,-39.4)) ;
#100637=CARTESIAN_POINT('Origin',(7.34999999999997,-5.25000000000002,-39.85)) ;
#100638=CARTESIAN_POINT('Origin',(7.34999999999996,-15.1,-39.85)) ;
#100639=CARTESIAN_POINT('Origin',(10.5,-15.4,-39.85)) ;
#100640=CARTESIAN_POINT('Origin',(10.35,-15.4,-39.85)) ;
#100641=CARTESIAN_POINT('Origin',(7.64999999999996,-15.4,-39.85)) ;
#100642=CARTESIAN_POINT('Origin',(10.65,-5.25000000000002,-39.85)) ;
#100643=CARTESIAN_POINT('Origin',(10.65,-15.1,-39.85)) ;
#100644=CARTESIAN_POINT('Origin',(10.35,-5.40000000000007,40.001)) ;
#100645=CARTESIAN_POINT('Origin',(10.35,-5.40000000000002,-39.4)) ;
#100646=CARTESIAN_POINT('Origin',(10.5,-5.10000000000002,-39.4)) ;
#100647=CARTESIAN_POINT('Origin',(10.35,-5.10000000000002,-39.4)) ;
#100648=CARTESIAN_POINT('Origin',(7.64999999999997,-5.10000000000002,-39.4)) ;
#100649=CARTESIAN_POINT('Origin',(7.64999999999997,-5.40000000000002,-39.4)) ;
#100650=CARTESIAN_POINT('Origin',(7.34999999999997,-5.40000000000002,-39.4)) ;
#100651=CARTESIAN_POINT('Origin',(7.64999999999996,-15.1,-39.85)) ;
#100652=CARTESIAN_POINT('Origin',(7.64999999999996,-15.1,-39.85)) ;
#100653=CARTESIAN_POINT('Origin',(10.35,-15.1,-39.85)) ;
#100654=CARTESIAN_POINT('Origin',(10.35,-15.1,-39.85)) ;
#100655=CARTESIAN_POINT('Origin',(10.35,-5.40000000000002,-39.4)) ;
#100656=CARTESIAN_POINT('Origin',(10.65,-5.40000000000002,-39.4)) ;
#100657=CARTESIAN_POINT('Origin',(7.34999999999997,-5.25000000000002,-39.4)) ;
#100658=CARTESIAN_POINT('Origin',(7.34999999999996,-15.1,-39.4)) ;
#100659=CARTESIAN_POINT('Origin',(7.64999999999996,-15.1000000000001,40.001)) ;
#100660=CARTESIAN_POINT('Origin',(7.64999999999996,-15.1,-39.4)) ;
#100661=CARTESIAN_POINT('Origin',(10.35,-15.1000000000001,40.001)) ;
#100662=CARTESIAN_POINT('Origin',(10.35,-15.1,-39.4)) ;
#100663=CARTESIAN_POINT('Origin',(10.65,-5.25000000000002,-39.4)) ;
#100664=CARTESIAN_POINT('Origin',(10.65,-15.1,-39.4)) ;
#100665=CARTESIAN_POINT('Origin',(7.64999999999996,-15.1,-39.4)) ;
#100666=CARTESIAN_POINT('Origin',(7.64999999999996,-15.4,-39.4)) ;
#100667=CARTESIAN_POINT('Origin',(10.35,-15.1,-39.4)) ;
#100668=CARTESIAN_POINT('Origin',(10.35,-15.4,-39.4)) ;
#100669=CARTESIAN_POINT('Origin',(10.5,-15.4,-39.4)) ;
#100670=CARTESIAN_POINT('Origin',(16.5,-15.4000000000001,-39.85)) ;
#100671=CARTESIAN_POINT('Origin',(16.35,-15.4000000000001,-39.85)) ;
#100672=CARTESIAN_POINT('Origin',(13.65,-15.4000000000001,-39.85)) ;
#100673=CARTESIAN_POINT('Origin',(16.35,-15.1000000000001,-39.85)) ;
#100674=CARTESIAN_POINT('Origin',(16.35,-15.1000000000001,-39.85)) ;
#100675=CARTESIAN_POINT('Origin',(16.65,-15.1000000000001,-39.85)) ;
#100676=CARTESIAN_POINT('Origin',(13.65,-15.1000000000001,-39.85)) ;
#100677=CARTESIAN_POINT('Origin',(13.35,-15.1000000000001,-39.85)) ;
#100678=CARTESIAN_POINT('Origin',(13.65,-15.1000000000001,-39.85)) ;
#100679=CARTESIAN_POINT('Origin',(16.35,-15.1000000000001,40.001)) ;
#100680=CARTESIAN_POINT('Origin',(16.35,-15.1000000000001,-39.4)) ;
#100681=CARTESIAN_POINT('Origin',(16.65,-5.25000000000006,-39.85)) ;
#100682=CARTESIAN_POINT('Origin',(16.65,-5.40000000000006,-39.85)) ;
#100683=CARTESIAN_POINT('Origin',(16.5,-5.10000000000006,-39.85)) ;
#100684=CARTESIAN_POINT('Origin',(13.65,-5.10000000000006,-39.85)) ;
#100685=CARTESIAN_POINT('Origin',(16.35,-5.10000000000006,-39.85)) ;
#100686=CARTESIAN_POINT('Origin',(13.35,-5.25000000000006,-39.85)) ;
#100687=CARTESIAN_POINT('Origin',(13.35,-5.40000000000006,-39.85)) ;
#100688=CARTESIAN_POINT('Origin',(13.65,-15.1000000000001,40.001)) ;
#100689=CARTESIAN_POINT('Origin',(13.65,-15.1000000000001,-39.4)) ;
#100690=CARTESIAN_POINT('Origin',(16.5,-15.4000000000001,-39.4)) ;
#100691=CARTESIAN_POINT('Origin',(13.65,-15.4000000000001,-39.4)) ;
#100692=CARTESIAN_POINT('Origin',(16.35,-15.4000000000001,-39.4)) ;
#100693=CARTESIAN_POINT('Origin',(16.35,-15.1000000000001,-39.4)) ;
#100694=CARTESIAN_POINT('Origin',(16.65,-15.1000000000001,-39.4)) ;
#100695=CARTESIAN_POINT('Origin',(16.35,-5.40000000000006,-39.85)) ;
#100696=CARTESIAN_POINT('Origin',(16.35,-5.40000000000006,-39.85)) ;
#100697=CARTESIAN_POINT('Origin',(13.65,-5.40000000000006,-39.85)) ;
#100698=CARTESIAN_POINT('Origin',(13.65,-5.40000000000006,-39.85)) ;
#100699=CARTESIAN_POINT('Origin',(13.65,-15.1000000000001,-39.4)) ;
#100700=CARTESIAN_POINT('Origin',(13.35,-15.1000000000001,-39.4)) ;
#100701=CARTESIAN_POINT('Origin',(16.65,-5.25000000000006,-39.4)) ;
#100702=CARTESIAN_POINT('Origin',(16.65,-5.40000000000006,-39.4)) ;
#100703=CARTESIAN_POINT('Origin',(16.35,-5.40000000000011,40.001)) ;
#100704=CARTESIAN_POINT('Origin',(16.35,-5.40000000000006,-39.4)) ;
#100705=CARTESIAN_POINT('Origin',(13.65,-5.40000000000011,40.001)) ;
#100706=CARTESIAN_POINT('Origin',(13.65,-5.40000000000006,-39.4)) ;
#100707=CARTESIAN_POINT('Origin',(13.35,-5.25000000000006,-39.4)) ;
#100708=CARTESIAN_POINT('Origin',(13.35,-5.40000000000006,-39.4)) ;
#100709=CARTESIAN_POINT('Origin',(16.35,-5.40000000000006,-39.4)) ;
#100710=CARTESIAN_POINT('Origin',(16.35,-5.10000000000006,-39.4)) ;
#100711=CARTESIAN_POINT('Origin',(13.65,-5.40000000000006,-39.4)) ;
#100712=CARTESIAN_POINT('Origin',(13.65,-5.10000000000006,-39.4)) ;
#100713=CARTESIAN_POINT('Origin',(16.5,-5.10000000000006,-39.4)) ;
#100714=CARTESIAN_POINT('Origin',(38.25,-2.60000000000002,-39.85)) ;
#100715=CARTESIAN_POINT('Origin',(19.4,-2.60000000000002,-39.85)) ;
#100716=CARTESIAN_POINT('Origin',(38.1,-2.60000000000002,-39.85)) ;
#100717=CARTESIAN_POINT('Origin',(19.4,-2.90000000000002,-39.85)) ;
#100718=CARTESIAN_POINT('Origin',(19.4,-2.90000000000002,-39.85)) ;
#100719=CARTESIAN_POINT('Origin',(19.1,-2.90000000000002,-39.85)) ;
#100720=CARTESIAN_POINT('Origin',(38.1,-2.90000000000002,-39.85)) ;
#100721=CARTESIAN_POINT('Origin',(38.4,-2.90000000000002,-39.85)) ;
#100722=CARTESIAN_POINT('Origin',(38.1,-2.90000000000002,-39.85)) ;
#100723=CARTESIAN_POINT('Origin',(19.4,-2.90000000000007,40.001)) ;
#100724=CARTESIAN_POINT('Origin',(19.4,-2.90000000000002,-39.4)) ;
#100725=CARTESIAN_POINT('Origin',(19.1,-2.75000000000002,-39.85)) ;
#100726=CARTESIAN_POINT('Origin',(19.1,-13.1,-39.85)) ;
#100727=CARTESIAN_POINT('Origin',(38.25,-13.4,-39.85)) ;
#100728=CARTESIAN_POINT('Origin',(38.1,-13.4,-39.85)) ;
#100729=CARTESIAN_POINT('Origin',(19.4,-13.4,-39.85)) ;
#100730=CARTESIAN_POINT('Origin',(38.4,-2.75000000000002,-39.85)) ;
#100731=CARTESIAN_POINT('Origin',(38.4,-13.1,-39.85)) ;
#100732=CARTESIAN_POINT('Origin',(38.1,-2.90000000000007,40.001)) ;
#100733=CARTESIAN_POINT('Origin',(38.1,-2.90000000000002,-39.4)) ;
#100734=CARTESIAN_POINT('Origin',(38.25,-2.60000000000002,-39.4)) ;
#100735=CARTESIAN_POINT('Origin',(38.1,-2.60000000000002,-39.4)) ;
#100736=CARTESIAN_POINT('Origin',(19.4,-2.60000000000002,-39.4)) ;
#100737=CARTESIAN_POINT('Origin',(19.4,-2.90000000000002,-39.4)) ;
#100738=CARTESIAN_POINT('Origin',(19.1,-2.90000000000002,-39.4)) ;
#100739=CARTESIAN_POINT('Origin',(19.4,-13.1,-39.85)) ;
#100740=CARTESIAN_POINT('Origin',(19.4,-13.1,-39.85)) ;
#100741=CARTESIAN_POINT('Origin',(38.1,-13.1,-39.85)) ;
#100742=CARTESIAN_POINT('Origin',(38.1,-13.1,-39.85)) ;
#100743=CARTESIAN_POINT('Origin',(38.1,-2.90000000000002,-39.4)) ;
#100744=CARTESIAN_POINT('Origin',(38.4,-2.90000000000002,-39.4)) ;
#100745=CARTESIAN_POINT('Origin',(19.1,-2.75000000000002,-39.4)) ;
#100746=CARTESIAN_POINT('Origin',(19.1,-13.1,-39.4)) ;
#100747=CARTESIAN_POINT('Origin',(19.4,-13.1000000000001,40.001)) ;
#100748=CARTESIAN_POINT('Origin',(19.4,-13.1,-39.4)) ;
#100749=CARTESIAN_POINT('Origin',(38.1,-13.1000000000001,40.001)) ;
#100750=CARTESIAN_POINT('Origin',(38.1,-13.1,-39.4)) ;
#100751=CARTESIAN_POINT('Origin',(38.4,-2.75000000000002,-39.4)) ;
#100752=CARTESIAN_POINT('Origin',(38.4,-13.1,-39.4)) ;
#100753=CARTESIAN_POINT('Origin',(19.4,-13.1,-39.4)) ;
#100754=CARTESIAN_POINT('Origin',(19.4,-13.4,-39.4)) ;
#100755=CARTESIAN_POINT('Origin',(38.1,-13.1,-39.4)) ;
#100756=CARTESIAN_POINT('Origin',(38.1,-13.4,-39.4)) ;
#100757=CARTESIAN_POINT('Origin',(38.25,-13.4,-39.4)) ;
#100758=CARTESIAN_POINT('Origin',(46.5,-15.4000000000003,-39.85)) ;
#100759=CARTESIAN_POINT('Origin',(46.35,-15.4000000000003,-39.85)) ;
#100760=CARTESIAN_POINT('Origin',(43.65,-15.4000000000003,-39.85)) ;
#100761=CARTESIAN_POINT('Origin',(46.35,-15.1000000000003,-39.85)) ;
#100762=CARTESIAN_POINT('Origin',(46.35,-15.1000000000003,-39.85)) ;
#100763=CARTESIAN_POINT('Origin',(46.65,-15.1000000000003,-39.85)) ;
#100764=CARTESIAN_POINT('Origin',(43.65,-15.1000000000003,-39.85)) ;
#100765=CARTESIAN_POINT('Origin',(43.35,-15.1000000000003,-39.85)) ;
#100766=CARTESIAN_POINT('Origin',(43.65,-15.1000000000003,-39.85)) ;
#100767=CARTESIAN_POINT('Origin',(46.35,-15.1000000000003,40.001)) ;
#100768=CARTESIAN_POINT('Origin',(46.35,-15.1000000000003,-39.4)) ;
#100769=CARTESIAN_POINT('Origin',(46.65,-5.25000000000027,-39.85)) ;
#100770=CARTESIAN_POINT('Origin',(46.65,-5.40000000000027,-39.85)) ;
#100771=CARTESIAN_POINT('Origin',(46.5,-5.10000000000027,-39.85)) ;
#100772=CARTESIAN_POINT('Origin',(43.65,-5.10000000000027,-39.85)) ;
#100773=CARTESIAN_POINT('Origin',(46.35,-5.10000000000027,-39.85)) ;
#100774=CARTESIAN_POINT('Origin',(43.35,-5.25000000000027,-39.85)) ;
#100775=CARTESIAN_POINT('Origin',(43.35,-5.40000000000027,-39.85)) ;
#100776=CARTESIAN_POINT('Origin',(43.65,-15.1000000000003,40.001)) ;
#100777=CARTESIAN_POINT('Origin',(43.65,-15.1000000000003,-39.4)) ;
#100778=CARTESIAN_POINT('Origin',(46.5,-15.4000000000003,-39.4)) ;
#100779=CARTESIAN_POINT('Origin',(43.65,-15.4000000000003,-39.4)) ;
#100780=CARTESIAN_POINT('Origin',(46.35,-15.4000000000003,-39.4)) ;
#100781=CARTESIAN_POINT('Origin',(46.35,-15.1000000000003,-39.4)) ;
#100782=CARTESIAN_POINT('Origin',(46.65,-15.1000000000003,-39.4)) ;
#100783=CARTESIAN_POINT('Origin',(46.35,-5.40000000000027,-39.85)) ;
#100784=CARTESIAN_POINT('Origin',(46.35,-5.40000000000027,-39.85)) ;
#100785=CARTESIAN_POINT('Origin',(43.65,-5.40000000000027,-39.85)) ;
#100786=CARTESIAN_POINT('Origin',(43.65,-5.40000000000027,-39.85)) ;
#100787=CARTESIAN_POINT('Origin',(43.65,-15.1000000000003,-39.4)) ;
#100788=CARTESIAN_POINT('Origin',(43.35,-15.1000000000003,-39.4)) ;
#100789=CARTESIAN_POINT('Origin',(46.65,-5.25000000000027,-39.4)) ;
#100790=CARTESIAN_POINT('Origin',(46.65,-5.40000000000027,-39.4)) ;
#100791=CARTESIAN_POINT('Origin',(46.35,-5.40000000000032,40.001)) ;
#100792=CARTESIAN_POINT('Origin',(46.35,-5.40000000000027,-39.4)) ;
#100793=CARTESIAN_POINT('Origin',(43.65,-5.40000000000032,40.001)) ;
#100794=CARTESIAN_POINT('Origin',(43.65,-5.40000000000027,-39.4)) ;
#100795=CARTESIAN_POINT('Origin',(43.35,-5.25000000000027,-39.4)) ;
#100796=CARTESIAN_POINT('Origin',(43.35,-5.40000000000027,-39.4)) ;
#100797=CARTESIAN_POINT('Origin',(46.35,-5.40000000000027,-39.4)) ;
#100798=CARTESIAN_POINT('Origin',(46.35,-5.10000000000027,-39.4)) ;
#100799=CARTESIAN_POINT('Origin',(43.65,-5.40000000000027,-39.4)) ;
#100800=CARTESIAN_POINT('Origin',(43.65,-5.10000000000027,-39.4)) ;
#100801=CARTESIAN_POINT('Origin',(46.5,-5.10000000000027,-39.4)) ;
#100802=CARTESIAN_POINT('Origin',(53.8500000000001,-14.4,34.)) ;
#100803=CARTESIAN_POINT('Origin',(53.8500000000001,-14.4,33.85)) ;
#100804=CARTESIAN_POINT('Origin',(53.8500000000001,-14.4,-32.35)) ;
#100805=CARTESIAN_POINT('Origin',(53.8500000000001,-14.1,-32.35)) ;
#100806=CARTESIAN_POINT('Origin',(53.8500000000001,-14.1,-32.65)) ;
#100807=CARTESIAN_POINT('Origin',(53.8500000000001,-14.1,-32.35)) ;
#100808=CARTESIAN_POINT('Origin',(53.8500000000001,-14.1,33.85)) ;
#100809=CARTESIAN_POINT('Origin',(53.8500000000001,-14.1,33.85)) ;
#100810=CARTESIAN_POINT('Origin',(53.8500000000001,-14.1,34.15)) ;
#100811=CARTESIAN_POINT('Origin',(53.85,-4.24999999999999,-32.65)) ;
#100812=CARTESIAN_POINT('Origin',(53.85,-4.39999999999999,-32.65)) ;
#100813=CARTESIAN_POINT('Origin',(-2.00100000000007,-14.1000000000002,-32.35)) ;
#100814=CARTESIAN_POINT('Origin',(53.4,-14.1,-32.35)) ;
#100815=CARTESIAN_POINT('Origin',(53.4,-14.4,3.59310653001811E-29)) ;
#100816=CARTESIAN_POINT('Origin',(53.4,-14.4,33.85)) ;
#100817=CARTESIAN_POINT('Origin',(53.4,-14.4,-32.35)) ;
#100818=CARTESIAN_POINT('Origin',(-2.00100000000007,-14.1000000000002,33.85)) ;
#100819=CARTESIAN_POINT('Origin',(53.4,-14.1,33.85)) ;
#100820=CARTESIAN_POINT('Origin',(53.85,-4.24999999999999,34.15)) ;
#100821=CARTESIAN_POINT('Origin',(53.85,-4.4,34.15)) ;
#100822=CARTESIAN_POINT('Origin',(53.85,-4.1,34.)) ;
#100823=CARTESIAN_POINT('Origin',(53.85,-4.1,-32.35)) ;
#100824=CARTESIAN_POINT('Origin',(53.85,-4.1,33.85)) ;
#100825=CARTESIAN_POINT('Origin',(53.85,-4.4,-32.35)) ;
#100826=CARTESIAN_POINT('Origin',(53.85,-4.4,-32.35)) ;
#100827=CARTESIAN_POINT('Origin',(53.4,-14.1,-32.35)) ;
#100828=CARTESIAN_POINT('Origin',(53.4,-14.1,-32.65)) ;
#100829=CARTESIAN_POINT('Origin',(53.4,-14.1,33.85)) ;
#100830=CARTESIAN_POINT('Origin',(53.4,-14.1,34.15)) ;
#100831=CARTESIAN_POINT('Origin',(53.85,-4.4,33.85)) ;
#100832=CARTESIAN_POINT('Origin',(53.85,-4.4,33.85)) ;
#100833=CARTESIAN_POINT('Origin',(-2.00100000000011,-4.4000000000002,-32.35)) ;
#100834=CARTESIAN_POINT('Origin',(53.4,-4.4,-32.35)) ;
#100835=CARTESIAN_POINT('Origin',(53.4,1.95019439194024E-13,-32.65)) ;
#100836=CARTESIAN_POINT('Origin',(53.4,-4.4,-32.65)) ;
#100837=CARTESIAN_POINT('Origin',(53.4,1.95019439194024E-13,34.15)) ;
#100838=CARTESIAN_POINT('Origin',(53.4,-4.4,34.15)) ;
#100839=CARTESIAN_POINT('Origin',(-2.00100000000011,-4.4000000000002,33.85)) ;
#100840=CARTESIAN_POINT('Origin',(53.4,-4.4,33.85)) ;
#100841=CARTESIAN_POINT('Origin',(53.4,-4.4,-32.35)) ;
#100842=CARTESIAN_POINT('Origin',(53.4,-4.1,-32.35)) ;
#100843=CARTESIAN_POINT('Origin',(53.4,-4.4,33.85)) ;
#100844=CARTESIAN_POINT('Origin',(53.4,-4.1,33.85)) ;
#100845=CARTESIAN_POINT('Origin',(53.4,-4.1,3.59310653001811E-29)) ;
#100846=CARTESIAN_POINT('Origin',(43.5,-5.10000000000002,39.85)) ;
#100847=CARTESIAN_POINT('Origin',(46.35,-5.10000000000002,39.85)) ;
#100848=CARTESIAN_POINT('Origin',(43.65,-5.10000000000002,39.85)) ;
#100849=CARTESIAN_POINT('Origin',(46.35,-5.40000000000002,39.85)) ;
#100850=CARTESIAN_POINT('Origin',(46.35,-5.40000000000002,39.85)) ;
#100851=CARTESIAN_POINT('Origin',(46.65,-5.40000000000002,39.85)) ;
#100852=CARTESIAN_POINT('Origin',(43.65,-5.40000000000002,39.85)) ;
#100853=CARTESIAN_POINT('Origin',(43.35,-5.40000000000002,39.85)) ;
#100854=CARTESIAN_POINT('Origin',(43.65,-5.40000000000002,39.85)) ;
#100855=CARTESIAN_POINT('Origin',(46.35,-5.40000000000002,-40.001)) ;
#100856=CARTESIAN_POINT('Origin',(46.35,-5.40000000000002,39.4)) ;
#100857=CARTESIAN_POINT('Origin',(46.65,-5.25000000000002,39.85)) ;
#100858=CARTESIAN_POINT('Origin',(46.65,-15.1,39.85)) ;
#100859=CARTESIAN_POINT('Origin',(43.5,-15.4,39.85)) ;
#100860=CARTESIAN_POINT('Origin',(43.65,-15.4,39.85)) ;
#100861=CARTESIAN_POINT('Origin',(46.35,-15.4,39.85)) ;
#100862=CARTESIAN_POINT('Origin',(43.35,-5.25000000000002,39.85)) ;
#100863=CARTESIAN_POINT('Origin',(43.35,-15.1,39.85)) ;
#100864=CARTESIAN_POINT('Origin',(43.65,-5.40000000000002,-40.001)) ;
#100865=CARTESIAN_POINT('Origin',(43.65,-5.40000000000002,39.4)) ;
#100866=CARTESIAN_POINT('Origin',(43.5,-5.10000000000002,39.4)) ;
#100867=CARTESIAN_POINT('Origin',(43.65,-5.10000000000002,39.4)) ;
#100868=CARTESIAN_POINT('Origin',(46.35,-5.10000000000002,39.4)) ;
#100869=CARTESIAN_POINT('Origin',(46.35,-5.40000000000002,39.4)) ;
#100870=CARTESIAN_POINT('Origin',(46.65,-5.40000000000002,39.4)) ;
#100871=CARTESIAN_POINT('Origin',(46.35,-15.1,39.85)) ;
#100872=CARTESIAN_POINT('Origin',(46.35,-15.1,39.85)) ;
#100873=CARTESIAN_POINT('Origin',(43.65,-15.1,39.85)) ;
#100874=CARTESIAN_POINT('Origin',(43.65,-15.1,39.85)) ;
#100875=CARTESIAN_POINT('Origin',(43.65,-5.40000000000002,39.4)) ;
#100876=CARTESIAN_POINT('Origin',(43.35,-5.40000000000002,39.4)) ;
#100877=CARTESIAN_POINT('Origin',(46.65,-5.25000000000002,39.4)) ;
#100878=CARTESIAN_POINT('Origin',(46.65,-15.1,39.4)) ;
#100879=CARTESIAN_POINT('Origin',(46.35,-15.1,-40.001)) ;
#100880=CARTESIAN_POINT('Origin',(46.35,-15.1,39.4)) ;
#100881=CARTESIAN_POINT('Origin',(43.65,-15.1,-40.001)) ;
#100882=CARTESIAN_POINT('Origin',(43.65,-15.1,39.4)) ;
#100883=CARTESIAN_POINT('Origin',(43.35,-5.25000000000002,39.4)) ;
#100884=CARTESIAN_POINT('Origin',(43.35,-15.1,39.4)) ;
#100885=CARTESIAN_POINT('Origin',(46.35,-15.1,39.4)) ;
#100886=CARTESIAN_POINT('Origin',(46.35,-15.4,39.4)) ;
#100887=CARTESIAN_POINT('Origin',(43.65,-15.1,39.4)) ;
#100888=CARTESIAN_POINT('Origin',(43.65,-15.4,39.4)) ;
#100889=CARTESIAN_POINT('Origin',(43.5,-15.4,39.4)) ;
#100890=CARTESIAN_POINT('Origin',(37.5,-5.10000000000002,39.85)) ;
#100891=CARTESIAN_POINT('Origin',(40.35,-5.10000000000002,39.85)) ;
#100892=CARTESIAN_POINT('Origin',(37.65,-5.10000000000002,39.85)) ;
#100893=CARTESIAN_POINT('Origin',(40.35,-5.40000000000002,39.85)) ;
#100894=CARTESIAN_POINT('Origin',(40.35,-5.40000000000002,39.85)) ;
#100895=CARTESIAN_POINT('Origin',(40.65,-5.40000000000002,39.85)) ;
#100896=CARTESIAN_POINT('Origin',(37.65,-5.40000000000002,39.85)) ;
#100897=CARTESIAN_POINT('Origin',(37.35,-5.40000000000002,39.85)) ;
#100898=CARTESIAN_POINT('Origin',(37.65,-5.40000000000002,39.85)) ;
#100899=CARTESIAN_POINT('Origin',(40.35,-5.40000000000002,-40.001)) ;
#100900=CARTESIAN_POINT('Origin',(40.35,-5.40000000000002,39.4)) ;
#100901=CARTESIAN_POINT('Origin',(40.65,-5.25000000000002,39.85)) ;
#100902=CARTESIAN_POINT('Origin',(40.65,-15.1,39.85)) ;
#100903=CARTESIAN_POINT('Origin',(37.5,-15.4,39.85)) ;
#100904=CARTESIAN_POINT('Origin',(37.65,-15.4,39.85)) ;
#100905=CARTESIAN_POINT('Origin',(40.35,-15.4,39.85)) ;
#100906=CARTESIAN_POINT('Origin',(37.35,-5.25000000000002,39.85)) ;
#100907=CARTESIAN_POINT('Origin',(37.35,-15.1,39.85)) ;
#100908=CARTESIAN_POINT('Origin',(37.65,-5.40000000000002,-40.001)) ;
#100909=CARTESIAN_POINT('Origin',(37.65,-5.40000000000002,39.4)) ;
#100910=CARTESIAN_POINT('Origin',(37.5,-5.10000000000002,39.4)) ;
#100911=CARTESIAN_POINT('Origin',(37.65,-5.10000000000002,39.4)) ;
#100912=CARTESIAN_POINT('Origin',(40.35,-5.10000000000002,39.4)) ;
#100913=CARTESIAN_POINT('Origin',(40.35,-5.40000000000002,39.4)) ;
#100914=CARTESIAN_POINT('Origin',(40.65,-5.40000000000002,39.4)) ;
#100915=CARTESIAN_POINT('Origin',(40.35,-15.1,39.85)) ;
#100916=CARTESIAN_POINT('Origin',(40.35,-15.1,39.85)) ;
#100917=CARTESIAN_POINT('Origin',(37.65,-15.1,39.85)) ;
#100918=CARTESIAN_POINT('Origin',(37.65,-15.1,39.85)) ;
#100919=CARTESIAN_POINT('Origin',(37.65,-5.40000000000002,39.4)) ;
#100920=CARTESIAN_POINT('Origin',(37.35,-5.40000000000002,39.4)) ;
#100921=CARTESIAN_POINT('Origin',(40.65,-5.25000000000002,39.4)) ;
#100922=CARTESIAN_POINT('Origin',(40.65,-15.1,39.4)) ;
#100923=CARTESIAN_POINT('Origin',(40.35,-15.1,-40.001)) ;
#100924=CARTESIAN_POINT('Origin',(40.35,-15.1,39.4)) ;
#100925=CARTESIAN_POINT('Origin',(37.65,-15.1,-40.001)) ;
#100926=CARTESIAN_POINT('Origin',(37.65,-15.1,39.4)) ;
#100927=CARTESIAN_POINT('Origin',(37.35,-5.25000000000002,39.4)) ;
#100928=CARTESIAN_POINT('Origin',(37.35,-15.1,39.4)) ;
#100929=CARTESIAN_POINT('Origin',(40.35,-15.1,39.4)) ;
#100930=CARTESIAN_POINT('Origin',(40.35,-15.4,39.4)) ;
#100931=CARTESIAN_POINT('Origin',(37.65,-15.1,39.4)) ;
#100932=CARTESIAN_POINT('Origin',(37.65,-15.4,39.4)) ;
#100933=CARTESIAN_POINT('Origin',(37.5,-15.4,39.4)) ;
#100934=CARTESIAN_POINT('Origin',(31.5,-5.10000000000002,39.85)) ;
#100935=CARTESIAN_POINT('Origin',(34.35,-5.10000000000002,39.85)) ;
#100936=CARTESIAN_POINT('Origin',(31.65,-5.10000000000002,39.85)) ;
#100937=CARTESIAN_POINT('Origin',(34.35,-5.40000000000002,39.85)) ;
#100938=CARTESIAN_POINT('Origin',(34.35,-5.40000000000002,39.85)) ;
#100939=CARTESIAN_POINT('Origin',(34.65,-5.40000000000002,39.85)) ;
#100940=CARTESIAN_POINT('Origin',(31.65,-5.40000000000002,39.85)) ;
#100941=CARTESIAN_POINT('Origin',(31.35,-5.40000000000002,39.85)) ;
#100942=CARTESIAN_POINT('Origin',(31.65,-5.40000000000002,39.85)) ;
#100943=CARTESIAN_POINT('Origin',(34.35,-5.40000000000002,-40.001)) ;
#100944=CARTESIAN_POINT('Origin',(34.35,-5.40000000000002,39.4)) ;
#100945=CARTESIAN_POINT('Origin',(34.65,-5.25000000000002,39.85)) ;
#100946=CARTESIAN_POINT('Origin',(34.65,-15.1,39.85)) ;
#100947=CARTESIAN_POINT('Origin',(31.5,-15.4,39.85)) ;
#100948=CARTESIAN_POINT('Origin',(31.65,-15.4,39.85)) ;
#100949=CARTESIAN_POINT('Origin',(34.35,-15.4,39.85)) ;
#100950=CARTESIAN_POINT('Origin',(31.35,-5.25000000000002,39.85)) ;
#100951=CARTESIAN_POINT('Origin',(31.35,-15.1,39.85)) ;
#100952=CARTESIAN_POINT('Origin',(31.65,-5.40000000000002,-40.001)) ;
#100953=CARTESIAN_POINT('Origin',(31.65,-5.40000000000002,39.4)) ;
#100954=CARTESIAN_POINT('Origin',(31.5,-5.10000000000002,39.4)) ;
#100955=CARTESIAN_POINT('Origin',(31.65,-5.10000000000002,39.4)) ;
#100956=CARTESIAN_POINT('Origin',(34.35,-5.10000000000002,39.4)) ;
#100957=CARTESIAN_POINT('Origin',(34.35,-5.40000000000002,39.4)) ;
#100958=CARTESIAN_POINT('Origin',(34.65,-5.40000000000002,39.4)) ;
#100959=CARTESIAN_POINT('Origin',(34.35,-15.1,39.85)) ;
#100960=CARTESIAN_POINT('Origin',(34.35,-15.1,39.85)) ;
#100961=CARTESIAN_POINT('Origin',(31.65,-15.1,39.85)) ;
#100962=CARTESIAN_POINT('Origin',(31.65,-15.1,39.85)) ;
#100963=CARTESIAN_POINT('Origin',(31.65,-5.40000000000002,39.4)) ;
#100964=CARTESIAN_POINT('Origin',(31.35,-5.40000000000002,39.4)) ;
#100965=CARTESIAN_POINT('Origin',(34.65,-5.25000000000002,39.4)) ;
#100966=CARTESIAN_POINT('Origin',(34.65,-15.1,39.4)) ;
#100967=CARTESIAN_POINT('Origin',(34.35,-15.1,-40.001)) ;
#100968=CARTESIAN_POINT('Origin',(34.35,-15.1,39.4)) ;
#100969=CARTESIAN_POINT('Origin',(31.65,-15.1,-40.001)) ;
#100970=CARTESIAN_POINT('Origin',(31.65,-15.1,39.4)) ;
#100971=CARTESIAN_POINT('Origin',(31.35,-5.25000000000002,39.4)) ;
#100972=CARTESIAN_POINT('Origin',(31.35,-15.1,39.4)) ;
#100973=CARTESIAN_POINT('Origin',(34.35,-15.1,39.4)) ;
#100974=CARTESIAN_POINT('Origin',(34.35,-15.4,39.4)) ;
#100975=CARTESIAN_POINT('Origin',(31.65,-15.1,39.4)) ;
#100976=CARTESIAN_POINT('Origin',(31.65,-15.4,39.4)) ;
#100977=CARTESIAN_POINT('Origin',(31.5,-15.4,39.4)) ;
#100978=CARTESIAN_POINT('Origin',(25.5,-5.10000000000002,39.85)) ;
#100979=CARTESIAN_POINT('Origin',(28.35,-5.10000000000002,39.85)) ;
#100980=CARTESIAN_POINT('Origin',(25.65,-5.10000000000002,39.85)) ;
#100981=CARTESIAN_POINT('Origin',(28.35,-5.40000000000002,39.85)) ;
#100982=CARTESIAN_POINT('Origin',(28.35,-5.40000000000002,39.85)) ;
#100983=CARTESIAN_POINT('Origin',(28.65,-5.40000000000002,39.85)) ;
#100984=CARTESIAN_POINT('Origin',(25.65,-5.40000000000002,39.85)) ;
#100985=CARTESIAN_POINT('Origin',(25.35,-5.40000000000002,39.85)) ;
#100986=CARTESIAN_POINT('Origin',(25.65,-5.40000000000002,39.85)) ;
#100987=CARTESIAN_POINT('Origin',(28.35,-5.40000000000002,-40.001)) ;
#100988=CARTESIAN_POINT('Origin',(28.35,-5.40000000000002,39.4)) ;
#100989=CARTESIAN_POINT('Origin',(28.65,-5.25000000000002,39.85)) ;
#100990=CARTESIAN_POINT('Origin',(28.65,-15.1,39.85)) ;
#100991=CARTESIAN_POINT('Origin',(25.5,-15.4,39.85)) ;
#100992=CARTESIAN_POINT('Origin',(25.65,-15.4,39.85)) ;
#100993=CARTESIAN_POINT('Origin',(28.35,-15.4,39.85)) ;
#100994=CARTESIAN_POINT('Origin',(25.35,-5.25000000000002,39.85)) ;
#100995=CARTESIAN_POINT('Origin',(25.35,-15.1,39.85)) ;
#100996=CARTESIAN_POINT('Origin',(25.65,-5.40000000000002,-40.001)) ;
#100997=CARTESIAN_POINT('Origin',(25.65,-5.40000000000002,39.4)) ;
#100998=CARTESIAN_POINT('Origin',(25.5,-5.10000000000002,39.4)) ;
#100999=CARTESIAN_POINT('Origin',(25.65,-5.10000000000002,39.4)) ;
#101000=CARTESIAN_POINT('Origin',(28.35,-5.10000000000002,39.4)) ;
#101001=CARTESIAN_POINT('Origin',(28.35,-5.40000000000002,39.4)) ;
#101002=CARTESIAN_POINT('Origin',(28.65,-5.40000000000002,39.4)) ;
#101003=CARTESIAN_POINT('Origin',(28.35,-15.1,39.85)) ;
#101004=CARTESIAN_POINT('Origin',(28.35,-15.1,39.85)) ;
#101005=CARTESIAN_POINT('Origin',(25.65,-15.1,39.85)) ;
#101006=CARTESIAN_POINT('Origin',(25.65,-15.1,39.85)) ;
#101007=CARTESIAN_POINT('Origin',(25.65,-5.40000000000002,39.4)) ;
#101008=CARTESIAN_POINT('Origin',(25.35,-5.40000000000002,39.4)) ;
#101009=CARTESIAN_POINT('Origin',(28.65,-5.25000000000002,39.4)) ;
#101010=CARTESIAN_POINT('Origin',(28.65,-15.1,39.4)) ;
#101011=CARTESIAN_POINT('Origin',(28.35,-15.1,-40.001)) ;
#101012=CARTESIAN_POINT('Origin',(28.35,-15.1,39.4)) ;
#101013=CARTESIAN_POINT('Origin',(25.65,-15.1,-40.001)) ;
#101014=CARTESIAN_POINT('Origin',(25.65,-15.1,39.4)) ;
#101015=CARTESIAN_POINT('Origin',(25.35,-5.25000000000002,39.4)) ;
#101016=CARTESIAN_POINT('Origin',(25.35,-15.1,39.4)) ;
#101017=CARTESIAN_POINT('Origin',(28.35,-15.1,39.4)) ;
#101018=CARTESIAN_POINT('Origin',(28.35,-15.4,39.4)) ;
#101019=CARTESIAN_POINT('Origin',(25.65,-15.1,39.4)) ;
#101020=CARTESIAN_POINT('Origin',(25.65,-15.4,39.4)) ;
#101021=CARTESIAN_POINT('Origin',(25.5,-15.4,39.4)) ;
#101022=CARTESIAN_POINT('Origin',(19.5,-5.10000000000002,39.85)) ;
#101023=CARTESIAN_POINT('Origin',(22.35,-5.10000000000002,39.85)) ;
#101024=CARTESIAN_POINT('Origin',(19.65,-5.10000000000002,39.85)) ;
#101025=CARTESIAN_POINT('Origin',(22.35,-5.40000000000002,39.85)) ;
#101026=CARTESIAN_POINT('Origin',(22.35,-5.40000000000002,39.85)) ;
#101027=CARTESIAN_POINT('Origin',(22.65,-5.40000000000002,39.85)) ;
#101028=CARTESIAN_POINT('Origin',(19.65,-5.40000000000002,39.85)) ;
#101029=CARTESIAN_POINT('Origin',(19.35,-5.40000000000002,39.85)) ;
#101030=CARTESIAN_POINT('Origin',(19.65,-5.40000000000002,39.85)) ;
#101031=CARTESIAN_POINT('Origin',(22.35,-5.40000000000002,-40.001)) ;
#101032=CARTESIAN_POINT('Origin',(22.35,-5.40000000000002,39.4)) ;
#101033=CARTESIAN_POINT('Origin',(22.65,-5.25000000000002,39.85)) ;
#101034=CARTESIAN_POINT('Origin',(22.65,-15.1,39.85)) ;
#101035=CARTESIAN_POINT('Origin',(19.5,-15.4,39.85)) ;
#101036=CARTESIAN_POINT('Origin',(19.65,-15.4,39.85)) ;
#101037=CARTESIAN_POINT('Origin',(22.35,-15.4,39.85)) ;
#101038=CARTESIAN_POINT('Origin',(19.35,-5.25000000000002,39.85)) ;
#101039=CARTESIAN_POINT('Origin',(19.35,-15.1,39.85)) ;
#101040=CARTESIAN_POINT('Origin',(19.65,-5.40000000000002,-40.001)) ;
#101041=CARTESIAN_POINT('Origin',(19.65,-5.40000000000002,39.4)) ;
#101042=CARTESIAN_POINT('Origin',(19.5,-5.10000000000002,39.4)) ;
#101043=CARTESIAN_POINT('Origin',(19.65,-5.10000000000002,39.4)) ;
#101044=CARTESIAN_POINT('Origin',(22.35,-5.10000000000002,39.4)) ;
#101045=CARTESIAN_POINT('Origin',(22.35,-5.40000000000002,39.4)) ;
#101046=CARTESIAN_POINT('Origin',(22.65,-5.40000000000002,39.4)) ;
#101047=CARTESIAN_POINT('Origin',(22.35,-15.1,39.85)) ;
#101048=CARTESIAN_POINT('Origin',(22.35,-15.1,39.85)) ;
#101049=CARTESIAN_POINT('Origin',(19.65,-15.1,39.85)) ;
#101050=CARTESIAN_POINT('Origin',(19.65,-15.1,39.85)) ;
#101051=CARTESIAN_POINT('Origin',(19.65,-5.40000000000002,39.4)) ;
#101052=CARTESIAN_POINT('Origin',(19.35,-5.40000000000002,39.4)) ;
#101053=CARTESIAN_POINT('Origin',(22.65,-5.25000000000002,39.4)) ;
#101054=CARTESIAN_POINT('Origin',(22.65,-15.1,39.4)) ;
#101055=CARTESIAN_POINT('Origin',(22.35,-15.1,-40.001)) ;
#101056=CARTESIAN_POINT('Origin',(22.35,-15.1,39.4)) ;
#101057=CARTESIAN_POINT('Origin',(19.65,-15.1,-40.001)) ;
#101058=CARTESIAN_POINT('Origin',(19.65,-15.1,39.4)) ;
#101059=CARTESIAN_POINT('Origin',(19.35,-5.25000000000002,39.4)) ;
#101060=CARTESIAN_POINT('Origin',(19.35,-15.1,39.4)) ;
#101061=CARTESIAN_POINT('Origin',(22.35,-15.1,39.4)) ;
#101062=CARTESIAN_POINT('Origin',(22.35,-15.4,39.4)) ;
#101063=CARTESIAN_POINT('Origin',(19.65,-15.1,39.4)) ;
#101064=CARTESIAN_POINT('Origin',(19.65,-15.4,39.4)) ;
#101065=CARTESIAN_POINT('Origin',(19.5,-15.4,39.4)) ;
#101066=CARTESIAN_POINT('Origin',(13.5,-15.4,39.85)) ;
#101067=CARTESIAN_POINT('Origin',(13.65,-15.4,39.85)) ;
#101068=CARTESIAN_POINT('Origin',(16.35,-15.4,39.85)) ;
#101069=CARTESIAN_POINT('Origin',(13.65,-15.1,39.85)) ;
#101070=CARTESIAN_POINT('Origin',(13.65,-15.1,39.85)) ;
#101071=CARTESIAN_POINT('Origin',(13.35,-15.1,39.85)) ;
#101072=CARTESIAN_POINT('Origin',(16.35,-15.1,39.85)) ;
#101073=CARTESIAN_POINT('Origin',(16.65,-15.1,39.85)) ;
#101074=CARTESIAN_POINT('Origin',(16.35,-15.1,39.85)) ;
#101075=CARTESIAN_POINT('Origin',(13.65,-15.1,-40.001)) ;
#101076=CARTESIAN_POINT('Origin',(13.65,-15.1,39.4)) ;
#101077=CARTESIAN_POINT('Origin',(13.35,-5.25000000000002,39.85)) ;
#101078=CARTESIAN_POINT('Origin',(13.35,-5.40000000000002,39.85)) ;
#101079=CARTESIAN_POINT('Origin',(13.5,-5.10000000000002,39.85)) ;
#101080=CARTESIAN_POINT('Origin',(16.35,-5.10000000000002,39.85)) ;
#101081=CARTESIAN_POINT('Origin',(13.65,-5.10000000000002,39.85)) ;
#101082=CARTESIAN_POINT('Origin',(16.65,-5.25000000000002,39.85)) ;
#101083=CARTESIAN_POINT('Origin',(16.65,-5.40000000000002,39.85)) ;
#101084=CARTESIAN_POINT('Origin',(16.35,-15.1,-40.001)) ;
#101085=CARTESIAN_POINT('Origin',(16.35,-15.1,39.4)) ;
#101086=CARTESIAN_POINT('Origin',(13.5,-15.4,39.4)) ;
#101087=CARTESIAN_POINT('Origin',(16.35,-15.4,39.4)) ;
#101088=CARTESIAN_POINT('Origin',(13.65,-15.4,39.4)) ;
#101089=CARTESIAN_POINT('Origin',(13.65,-15.1,39.4)) ;
#101090=CARTESIAN_POINT('Origin',(13.35,-15.1,39.4)) ;
#101091=CARTESIAN_POINT('Origin',(13.65,-5.40000000000002,39.85)) ;
#101092=CARTESIAN_POINT('Origin',(13.65,-5.40000000000002,39.85)) ;
#101093=CARTESIAN_POINT('Origin',(16.35,-5.40000000000002,39.85)) ;
#101094=CARTESIAN_POINT('Origin',(16.35,-5.40000000000002,39.85)) ;
#101095=CARTESIAN_POINT('Origin',(16.35,-15.1,39.4)) ;
#101096=CARTESIAN_POINT('Origin',(16.65,-15.1,39.4)) ;
#101097=CARTESIAN_POINT('Origin',(13.35,-5.25000000000002,39.4)) ;
#101098=CARTESIAN_POINT('Origin',(13.35,-5.40000000000002,39.4)) ;
#101099=CARTESIAN_POINT('Origin',(13.65,-5.40000000000002,-40.001)) ;
#101100=CARTESIAN_POINT('Origin',(13.65,-5.40000000000002,39.4)) ;
#101101=CARTESIAN_POINT('Origin',(16.35,-5.40000000000002,-40.001)) ;
#101102=CARTESIAN_POINT('Origin',(16.35,-5.40000000000002,39.4)) ;
#101103=CARTESIAN_POINT('Origin',(16.65,-5.25000000000002,39.4)) ;
#101104=CARTESIAN_POINT('Origin',(16.65,-5.40000000000002,39.4)) ;
#101105=CARTESIAN_POINT('Origin',(13.65,-5.40000000000002,39.4)) ;
#101106=CARTESIAN_POINT('Origin',(13.65,-5.10000000000002,39.4)) ;
#101107=CARTESIAN_POINT('Origin',(16.35,-5.40000000000002,39.4)) ;
#101108=CARTESIAN_POINT('Origin',(16.35,-5.10000000000002,39.4)) ;
#101109=CARTESIAN_POINT('Origin',(13.5,-5.10000000000002,39.4)) ;
#101110=CARTESIAN_POINT('Origin',(7.49999999999996,-5.10000000000002,39.85)) ;
#101111=CARTESIAN_POINT('Origin',(10.35,-5.10000000000002,39.85)) ;
#101112=CARTESIAN_POINT('Origin',(7.64999999999996,-5.10000000000002,39.85)) ;
#101113=CARTESIAN_POINT('Origin',(10.35,-5.40000000000002,39.85)) ;
#101114=CARTESIAN_POINT('Origin',(10.35,-5.40000000000002,39.85)) ;
#101115=CARTESIAN_POINT('Origin',(10.65,-5.40000000000002,39.85)) ;
#101116=CARTESIAN_POINT('Origin',(7.64999999999996,-5.40000000000002,39.85)) ;
#101117=CARTESIAN_POINT('Origin',(7.34999999999996,-5.40000000000002,39.85)) ;
#101118=CARTESIAN_POINT('Origin',(7.64999999999996,-5.40000000000002,39.85)) ;
#101119=CARTESIAN_POINT('Origin',(10.35,-5.40000000000002,-40.001)) ;
#101120=CARTESIAN_POINT('Origin',(10.35,-5.40000000000002,39.4)) ;
#101121=CARTESIAN_POINT('Origin',(10.65,-5.25000000000002,39.85)) ;
#101122=CARTESIAN_POINT('Origin',(10.65,-15.1,39.85)) ;
#101123=CARTESIAN_POINT('Origin',(7.49999999999997,-15.4,39.85)) ;
#101124=CARTESIAN_POINT('Origin',(7.64999999999997,-15.4,39.85)) ;
#101125=CARTESIAN_POINT('Origin',(10.35,-15.4,39.85)) ;
#101126=CARTESIAN_POINT('Origin',(7.34999999999996,-5.25000000000002,39.85)) ;
#101127=CARTESIAN_POINT('Origin',(7.34999999999997,-15.1,39.85)) ;
#101128=CARTESIAN_POINT('Origin',(7.64999999999996,-5.40000000000002,-40.001)) ;
#101129=CARTESIAN_POINT('Origin',(7.64999999999996,-5.40000000000002,39.4)) ;
#101130=CARTESIAN_POINT('Origin',(7.49999999999996,-5.10000000000002,39.4)) ;
#101131=CARTESIAN_POINT('Origin',(7.64999999999996,-5.10000000000002,39.4)) ;
#101132=CARTESIAN_POINT('Origin',(10.35,-5.10000000000002,39.4)) ;
#101133=CARTESIAN_POINT('Origin',(10.35,-5.40000000000002,39.4)) ;
#101134=CARTESIAN_POINT('Origin',(10.65,-5.40000000000002,39.4)) ;
#101135=CARTESIAN_POINT('Origin',(10.35,-15.1,39.85)) ;
#101136=CARTESIAN_POINT('Origin',(10.35,-15.1,39.85)) ;
#101137=CARTESIAN_POINT('Origin',(7.64999999999997,-15.1,39.85)) ;
#101138=CARTESIAN_POINT('Origin',(7.64999999999997,-15.1,39.85)) ;
#101139=CARTESIAN_POINT('Origin',(7.64999999999996,-5.40000000000002,39.4)) ;
#101140=CARTESIAN_POINT('Origin',(7.34999999999996,-5.40000000000002,39.4)) ;
#101141=CARTESIAN_POINT('Origin',(10.65,-5.25000000000002,39.4)) ;
#101142=CARTESIAN_POINT('Origin',(10.65,-15.1,39.4)) ;
#101143=CARTESIAN_POINT('Origin',(10.35,-15.1,-40.001)) ;
#101144=CARTESIAN_POINT('Origin',(10.35,-15.1,39.4)) ;
#101145=CARTESIAN_POINT('Origin',(7.64999999999997,-15.1,-40.001)) ;
#101146=CARTESIAN_POINT('Origin',(7.64999999999997,-15.1,39.4)) ;
#101147=CARTESIAN_POINT('Origin',(7.34999999999996,-5.25000000000002,39.4)) ;
#101148=CARTESIAN_POINT('Origin',(7.34999999999997,-15.1,39.4)) ;
#101149=CARTESIAN_POINT('Origin',(10.35,-15.1,39.4)) ;
#101150=CARTESIAN_POINT('Origin',(10.35,-15.4,39.4)) ;
#101151=CARTESIAN_POINT('Origin',(7.64999999999997,-15.1,39.4)) ;
#101152=CARTESIAN_POINT('Origin',(7.64999999999997,-15.4,39.4)) ;
#101153=CARTESIAN_POINT('Origin',(7.49999999999997,-15.4,39.4)) ;
#101154=CARTESIAN_POINT('Origin',(53.4,-1.75,39.85)) ;
#101155=CARTESIAN_POINT('Origin',(53.4000000000002,-1.90000000000016,39.8499999999998)) ;
#101156=CARTESIAN_POINT('Origin',(53.4000000000001,-19.6,39.85)) ;
#101157=CARTESIAN_POINT('Origin',(53.4,2.25743319424102E-13,-39.85)) ;
#101158=CARTESIAN_POINT('Origin',(53.4000000000001,-19.6,-39.85)) ;
#101159=CARTESIAN_POINT('Origin',(53.4,-1.89999999999994,-39.8500000000001)) ;
#101160=CARTESIAN_POINT('Origin',(53.4000000000001,-19.6,-38.25)) ;
#101161=CARTESIAN_POINT('Origin',(53.4000000000001,-19.6,39.85)) ;
#101162=CARTESIAN_POINT('Origin',(53.4000000000001,-19.6,-39.85)) ;
#101163=CARTESIAN_POINT('Origin',(53.4000000000001,-19.6,39.85)) ;
#101164=CARTESIAN_POINT('Origin',(53.4000000000001,-19.6,39.85)) ;
#101165=CARTESIAN_POINT('Origin',(54.,-1.89999999999999,39.85)) ;
#101166=CARTESIAN_POINT('Origin',(53.8500000000008,-1.89999999999927,39.8500000000007)) ;
#101167=CARTESIAN_POINT('Origin',(54.,-1.89999999999998,-39.85)) ;
#101168=CARTESIAN_POINT('Origin',(53.85,-1.9,-39.85)) ;
#101169=CARTESIAN_POINT('Origin',(53.4000000000001,-19.6,-39.85)) ;
#101170=CARTESIAN_POINT('Origin',(53.4000000000001,-19.6,-39.85)) ;
#101171=CARTESIAN_POINT('Origin',(54.0000000000001,-19.6,39.85)) ;
#101172=CARTESIAN_POINT('Origin',(53.8500000000001,-19.6,39.85)) ;
#101173=CARTESIAN_POINT('Origin',(53.85,1.96542435371224E-13,39.85)) ;
#101174=CARTESIAN_POINT('Origin',(53.8500000000001,-19.6,39.85)) ;
#101175=CARTESIAN_POINT('Origin',(53.85,-1.74999999999998,-39.85)) ;
#101176=CARTESIAN_POINT('Origin',(53.8500000000001,-19.6,-39.85)) ;
#101177=CARTESIAN_POINT('Origin',(54.0000000000001,-19.6,-39.85)) ;
#101178=CARTESIAN_POINT('Origin',(53.8500000000001,-19.6,-39.85)) ;
#101179=CARTESIAN_POINT('Origin',(53.8500000000001,-19.6,39.85)) ;
#101180=CARTESIAN_POINT('Origin',(53.8500000000001,-19.6,39.85)) ;
#101181=CARTESIAN_POINT('Origin',(53.8500000000001,-19.6,-39.85)) ;
#101182=CARTESIAN_POINT('Origin',(53.8500000000001,-19.6,-39.85)) ;
#101183=CARTESIAN_POINT('Origin',(53.8500000000001,-19.6,-3.55561622265573E-15)) ;
#126557=UNCERTAINTY_MEASURE_WITH_UNIT(LENGTH_MEASURE(0.01),#126572,
'DISTANCE_ACCURACY_VALUE',
'Maximum model space distance between geometric entities at asserted c
onnectivities') ;
#126563=UNCERTAINTY_MEASURE_WITH_UNIT(LENGTH_MEASURE(0.01),#126572,
'DISTANCE_ACCURACY_VALUE',
'Maximum model space distance between geometric entities at asserted c
onnectivities') ;
#126565=(
GEOMETRIC_REPRESENTATION_CONTEXT(3)
GLOBAL_UNCERTAINTY_ASSIGNED_CONTEXT((#126557))
GLOBAL_UNIT_ASSIGNED_CONTEXT((#126572,#126574,#126575))
REPRESENTATION_CONTEXT('','3D')
) ;
#126571=(
GEOMETRIC_REPRESENTATION_CONTEXT(3)
GLOBAL_UNCERTAINTY_ASSIGNED_CONTEXT((#126563))
GLOBAL_UNIT_ASSIGNED_CONTEXT((#126572,#126574,#126575))
REPRESENTATION_CONTEXT('','3D')
) ;
#126572=(
LENGTH_UNIT()
NAMED_UNIT(*)
SI_UNIT(.MILLI.,.METRE.)
) ;
#126574=(
NAMED_UNIT(*)
PLANE_ANGLE_UNIT()
SI_UNIT($,.RADIAN.)
) ;
#126575=(
NAMED_UNIT(*)
SI_UNIT($,.STERADIAN.)
SOLID_ANGLE_UNIT()
) ;
#126577=SHAPE_DEFINITION_REPRESENTATION(#126584,#126599) ;
#126584=PRODUCT_DEFINITION_SHAPE('',$,#126607) ;
#126599=SHAPE_REPRESENTATION('',(#67764),#126565) ;
#126605=PRODUCT_DEFINITION_CONTEXT('part definition',#126628,'design') ;
#126607=PRODUCT_DEFINITION('Enclosure_Cover','Enclosure_Cover',#126614,#126605) ;
#126614=PRODUCT_DEFINITION_FORMATION('',$,#126631) ;
#126628=APPLICATION_CONTEXT(
'Core Data for Automotive Mechanical Design Process') ;
#126629=PRODUCT_CONTEXT('part definition',#126628,'mechanical') ;
#126631=PRODUCT('Enclosure_Cover','Enclosure_Cover',$,(#126629)) ;
#126638=PRESENTATION_STYLE_ASSIGNMENT((#126647)) ;
#126647=SURFACE_STYLE_USAGE(.BOTH.,#126656) ;
#126656=SURFACE_SIDE_STYLE('',(#126665)) ;
#126665=SURFACE_STYLE_FILL_AREA(#126674) ;
#126674=FILL_AREA_STYLE('Opaque(228,233,237)',(#126683)) ;
#126683=FILL_AREA_STYLE_COLOUR('Opaque(228,233,237)',#126692) ;
#126692=COLOUR_RGB('Opaque(228,233,237)', 0.09019608, 0.27058824, 0.51372549) ;
ENDSEC;
END-ISO-10303-21;
